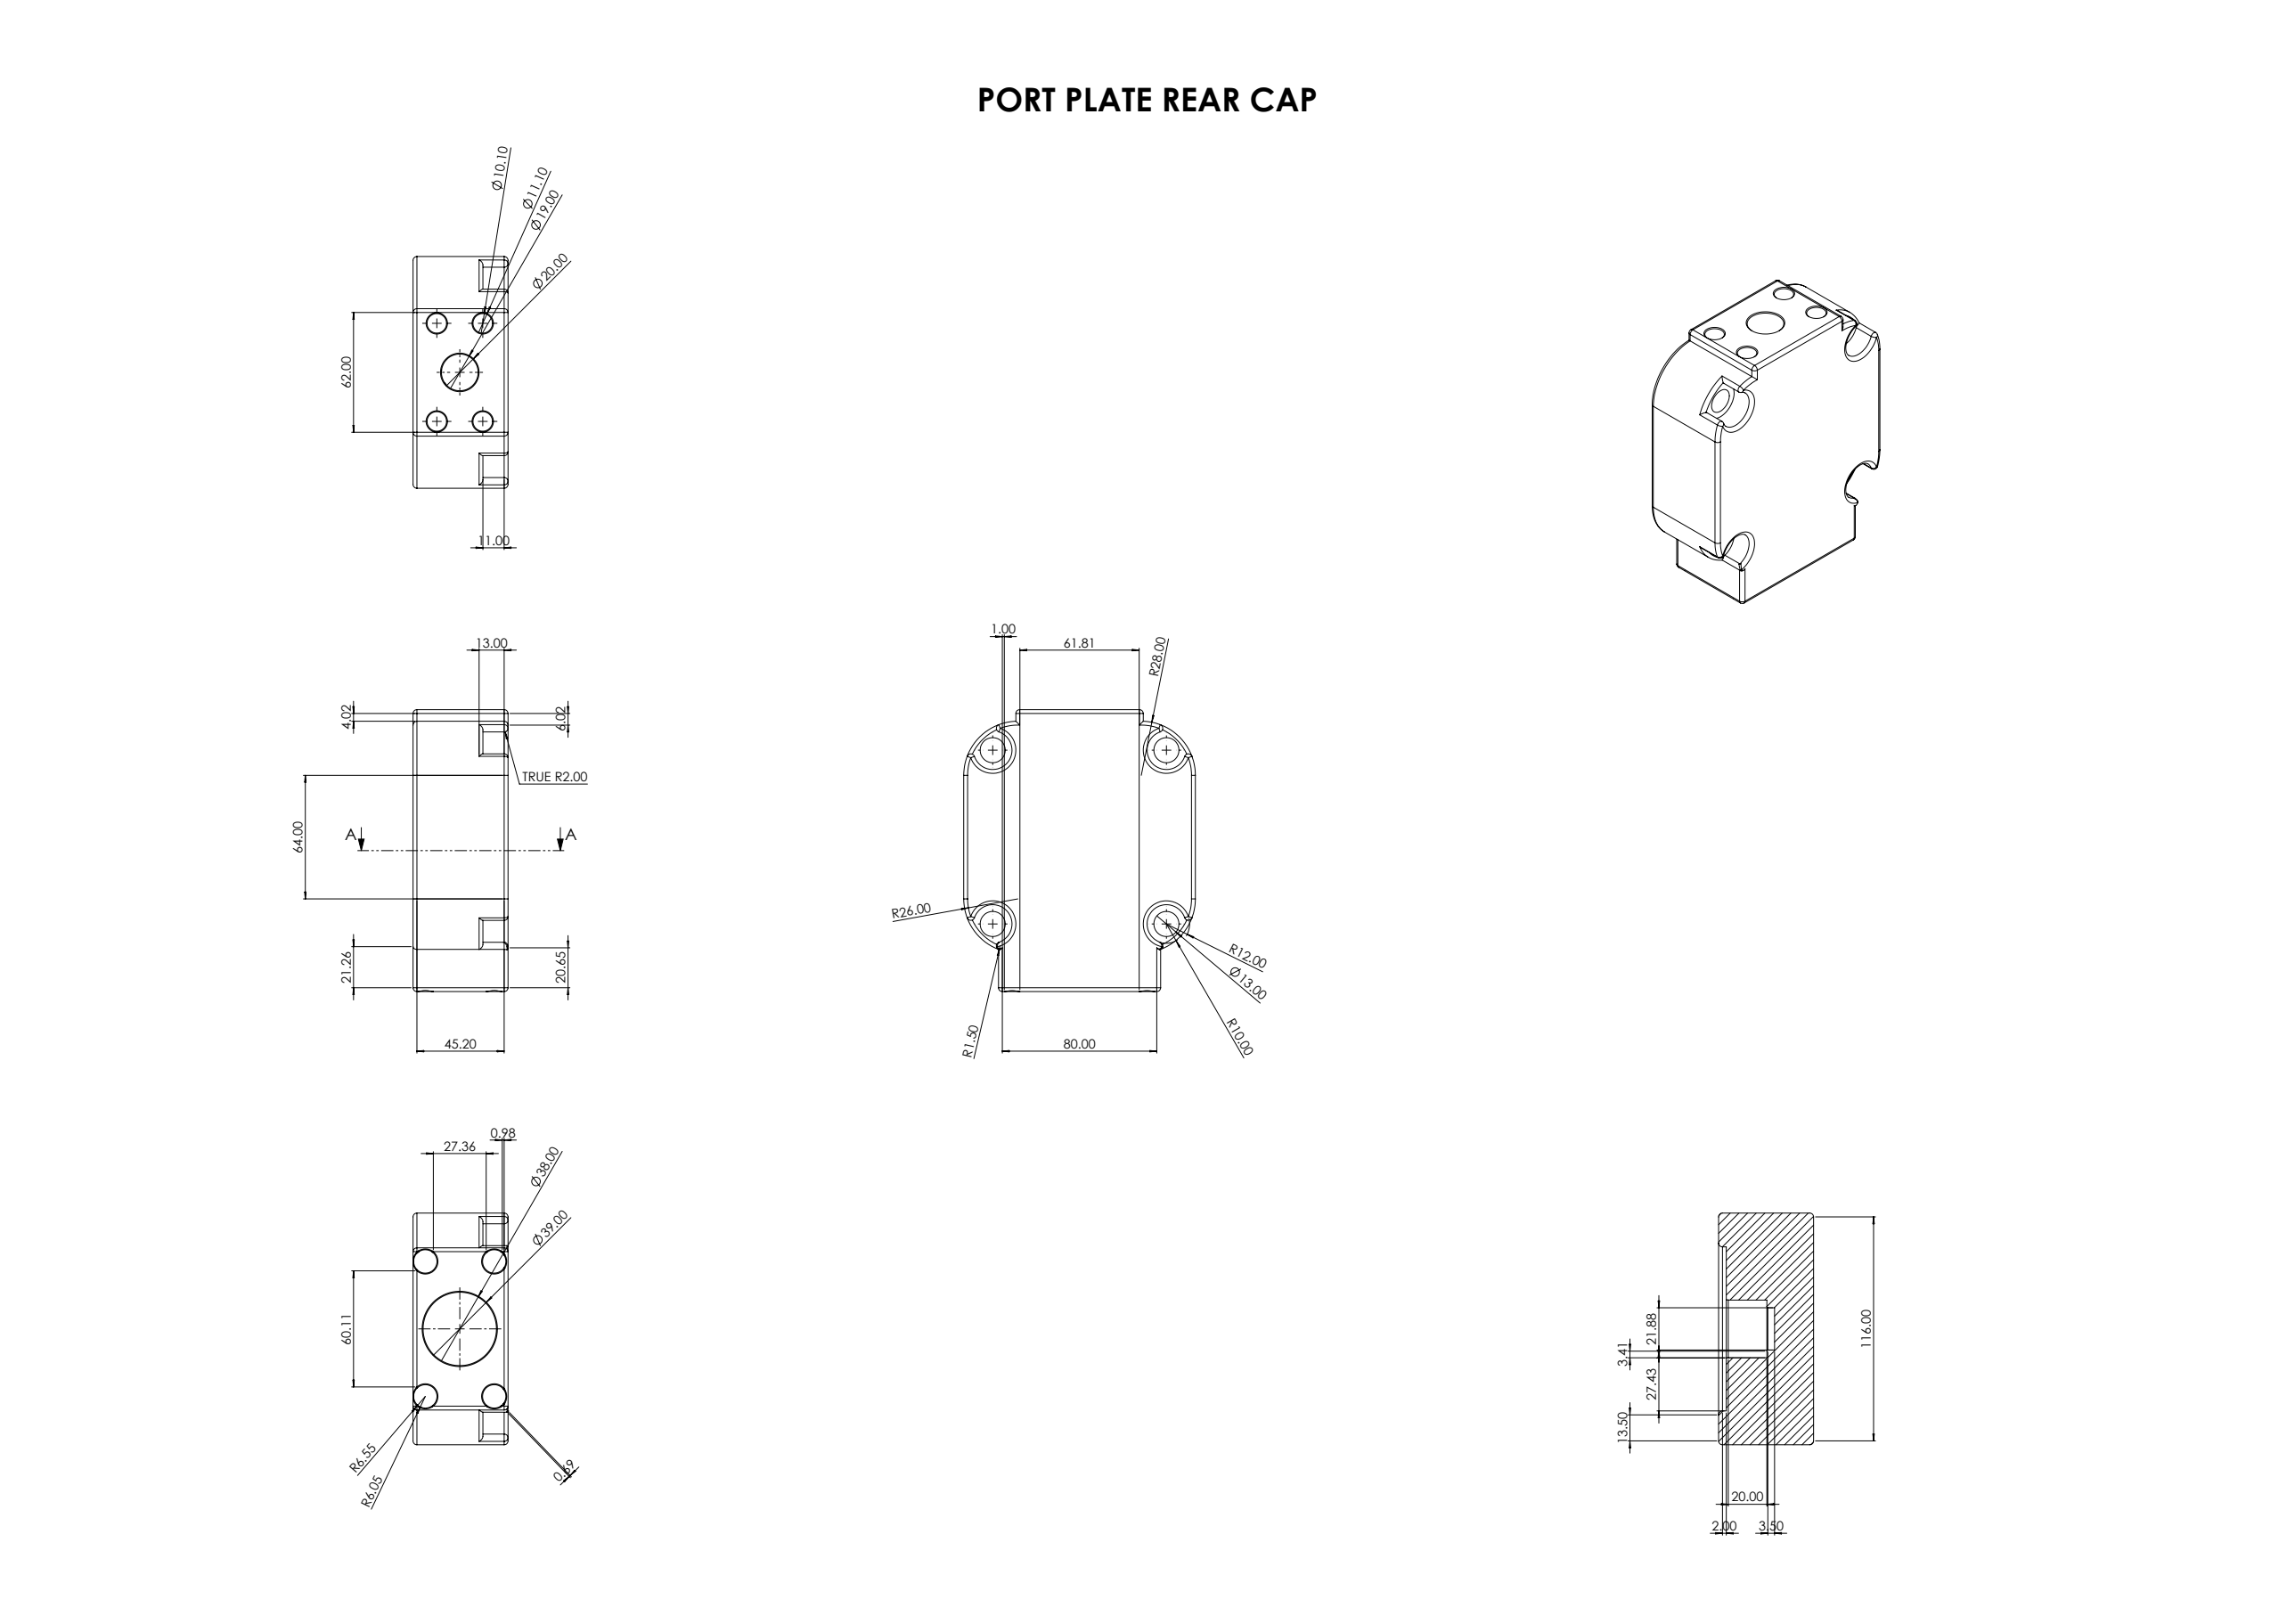
ISO-10303-21;
HEADER;
/* Generated by software containing ST-Developer
 * from STEP Tools, Inc. (www.steptools.com) 
 */

FILE_DESCRIPTION(
/* description */ (''),
/* implementation_level */ '2;1');

FILE_NAME(
/* name */ '02_Port_Plate_Rear_Cap.step',
/* time_stamp */ '2026-10-26T07:49:00-07:00',
/* author */ (''),
/* organization */ (''),
/* preprocessor_version */ 'ST-DEVELOPER v20.2',
/* originating_system */ 'Autodesk Translation Framework v15.15.0.0',
/* authorisation */ '');

FILE_SCHEMA (('AUTOMOTIVE_DESIGN { 1 0 10303 214 3 1 1 }'));
ENDSEC;

DATA;
#10=MECHANICAL_DESIGN_GEOMETRIC_PRESENTATION_REPRESENTATION('',(#178),#38507);
#132=SPHERICAL_SURFACE('',#15608,1.99999999999999);
#133=SPHERICAL_SURFACE('',#15617,2.);
#134=SPHERICAL_SURFACE('',#15621,2.);
#135=SPHERICAL_SURFACE('',#15628,2.);
#136=SPHERICAL_SURFACE('',#15630,2.);
#137=SPHERICAL_SURFACE('',#15636,2.);
#138=SPHERICAL_SURFACE('',#15638,2.);
#139=SPHERICAL_SURFACE('',#15719,2.);
#140=SPHERICAL_SURFACE('',#15722,2.);
#141=SPHERICAL_SURFACE('',#15737,2.);
#142=SPHERICAL_SURFACE('',#15745,1.99999999999999);
#143=SPHERICAL_SURFACE('',#15749,1.99999999999999);
#144=SPHERICAL_SURFACE('',#15753,1.99999999999999);
#145=SPHERICAL_SURFACE('',#15769,1.99999999999999);
#148=SHAPE_REPRESENTATION_RELATIONSHIP('SRR','None',#38576,#163);
#163=ADVANCED_BREP_SHAPE_REPRESENTATION('',(#193),#38493);
#178=STYLED_ITEM('',(#38713),#193);
#193=MANIFOLD_SOLID_BREP('Body1',#15072);
#215=B_SPLINE_SURFACE_WITH_KNOTS('',3,3,((#22745,#22746,#22747,#22748,#22749,
#22750,#22751,#22752,#22753,#22754,#22755,#22756),(#22757,#22758,#22759,
#22760,#22761,#22762,#22763,#22764,#22765,#22766,#22767,#22768),(#22769,
#22770,#22771,#22772,#22773,#22774,#22775,#22776,#22777,#22778,#22779,#22780),
(#22781,#22782,#22783,#22784,#22785,#22786,#22787,#22788,#22789,#22790,
#22791,#22792)),.UNSPECIFIED.,.F.,.F.,.F.,(4,4),(4,2,2,2,2,4),(0.,1.),(1.10145879772751,
1.32414222732706,1.45197453595802,1.57980684458897,1.70763915321993,1.80249027418853),
 .UNSPECIFIED.);
#216=B_SPLINE_SURFACE_WITH_KNOTS('',3,3,((#22823,#22824,#22825,#22826),
(#22827,#22828,#22829,#22830),(#22831,#22832,#22833,#22834),(#22835,#22836,
#22837,#22838)),.UNSPECIFIED.,.F.,.F.,.F.,(4,4),(4,4),(0.,1.),(-2.26119471261739,
-2.15398534032161),.UNSPECIFIED.);
#217=B_SPLINE_SURFACE_WITH_KNOTS('',3,3,((#22856,#22857,#22858,#22859),
(#22860,#22861,#22862,#22863),(#22864,#22865,#22866,#22867),(#22868,#22869,
#22870,#22871)),.UNSPECIFIED.,.F.,.F.,.F.,(4,4),(4,4),(0.,1.),(-0.987607313268187,
-0.880397940972402),.UNSPECIFIED.);
#218=B_SPLINE_SURFACE_WITH_KNOTS('',3,3,((#22880,#22881,#22882,#22883,#22884,
#22885,#22886,#22887),(#22888,#22889,#22890,#22891,#22892,#22893,#22894,
#22895),(#22896,#22897,#22898,#22899,#22900,#22901,#22902,#22903),(#22904,
#22905,#22906,#22907,#22908,#22909,#22910,#22911)),.UNSPECIFIED.,.F.,.F.,
 .F.,(4,4),(4,1,1,2,4),(0.,1.),(2.51916325679745,2.63563179243579,2.86856886371248,
3.10150593498916,3.18038929530694),.UNSPECIFIED.);
#219=B_SPLINE_SURFACE_WITH_KNOTS('',3,3,((#22934,#22935,#22936,#22937),
(#22938,#22939,#22940,#22941),(#22942,#22943,#22944,#22945),(#22946,#22947,
#22948,#22949)),.UNSPECIFIED.,.F.,.F.,.F.,(4,4),(4,4),(0.,1.),(-0.666064399610344,
-0.552453261527181),.UNSPECIFIED.);
#220=B_SPLINE_SURFACE_WITH_KNOTS('',3,3,((#22958,#22959,#22960,#22961),
(#22962,#22963,#22964,#22965),(#22966,#22967,#22968,#22969),(#22970,#22971,
#22972,#22973)),.UNSPECIFIED.,.F.,.F.,.F.,(4,4),(4,4),(0.,1.),(-5.7307320456524,
-5.61712090756923),.UNSPECIFIED.);
#221=B_SPLINE_SURFACE_WITH_KNOTS('',3,3,((#23021,#23022,#23023,#23024,#23025,
#23026,#23027,#23028,#23029,#23030,#23031,#23032),(#23033,#23034,#23035,
#23036,#23037,#23038,#23039,#23040,#23041,#23042,#23043,#23044),(#23045,
#23046,#23047,#23048,#23049,#23050,#23051,#23052,#23053,#23054,#23055,#23056),
(#23057,#23058,#23059,#23060,#23061,#23062,#23063,#23064,#23065,#23066,
#23067,#23068)),.UNSPECIFIED.,.F.,.F.,.F.,(4,4),(4,1,1,1,1,1,1,2,4),(0.,
1.),(1.17201798267167,1.354117347086,1.53621671150032,1.62726639370748,
1.67279123481106,1.71831607591465,1.90041544032897,2.08251480474329,2.14666332293336),
 .UNSPECIFIED.);
#222=B_SPLINE_SURFACE_WITH_KNOTS('',3,3,((#23104,#23105,#23106,#23107),
(#23108,#23109,#23110,#23111),(#23112,#23113,#23114,#23115),(#23116,#23117,
#23118,#23119)),.UNSPECIFIED.,.F.,.F.,.F.,(4,4),(4,4),(0.,1.),(2.29711532831763,
2.37317063593509),.UNSPECIFIED.);
#223=B_SPLINE_SURFACE_WITH_KNOTS('',3,3,((#23137,#23138,#23139,#23140),
(#23141,#23142,#23143,#23144),(#23145,#23146,#23147,#23148),(#23149,#23150,
#23151,#23152)),.UNSPECIFIED.,.F.,.F.,.F.,(4,4),(4,4),(0.,1.),(-2.37317063593509,
-2.29711532831763),.UNSPECIFIED.);
#224=B_SPLINE_SURFACE_WITH_KNOTS('',3,3,((#23161,#23162,#23163,#23164,#23165,
#23166,#23167,#23168),(#23169,#23170,#23171,#23172,#23173,#23174,#23175,
#23176),(#23177,#23178,#23179,#23180,#23181,#23182,#23183,#23184),(#23185,
#23186,#23187,#23188,#23189,#23190,#23191,#23192)),.UNSPECIFIED.,.F.,.F.,
 .F.,(4,4),(4,1,1,2,4),(0.,1.),(1.10145879772751,1.34393093992448,1.46516701102296,
1.70763915321993,1.80249027418852),.UNSPECIFIED.);
#225=B_SPLINE_SURFACE_WITH_KNOTS('',3,3,((#23215,#23216,#23217,#23218),
(#23219,#23220,#23221,#23222),(#23223,#23224,#23225,#23226),(#23227,#23228,
#23229,#23230)),.UNSPECIFIED.,.F.,.F.,.F.,(4,4),(4,4),(0.,1.),(-2.26119471261739,
-2.1539853403216),.UNSPECIFIED.);
#226=B_SPLINE_SURFACE_WITH_KNOTS('',3,3,((#23239,#23240,#23241,#23242),
(#23243,#23244,#23245,#23246),(#23247,#23248,#23249,#23250),(#23251,#23252,
#23253,#23254)),.UNSPECIFIED.,.F.,.F.,.F.,(4,4),(4,4),(0.,1.),(-0.987607313268191,
-0.880397940972402),.UNSPECIFIED.);
#227=B_SPLINE_SURFACE_WITH_KNOTS('',3,3,((#23285,#23286,#23287,#23288,#23289,
#23290,#23291,#23292,#23293,#23294),(#23295,#23296,#23297,#23298,#23299,
#23300,#23301,#23302,#23303,#23304),(#23305,#23306,#23307,#23308,#23309,
#23310,#23311,#23312,#23313,#23314),(#23315,#23316,#23317,#23318,#23319,
#23320,#23321,#23322,#23323,#23324)),.UNSPECIFIED.,.F.,.F.,.F.,(4,4),(4,
2,1,1,1,1,4),(0.,1.),(2.55343333368553,2.64828445465413,2.76952052575261,
2.89075659685109,3.01199266794958,3.07261070349882,3.25446481014654),
 .UNSPECIFIED.);
#228=B_SPLINE_SURFACE_WITH_KNOTS('',3,3,((#23351,#23352,#23353,#23354),
(#23355,#23356,#23357,#23358),(#23359,#23360,#23361,#23362),(#23363,#23364,
#23365,#23366)),.UNSPECIFIED.,.F.,.F.,.F.,(4,4),(4,4),(0.,1.),(-5.40278736620718,
-5.29557799391139),.UNSPECIFIED.);
#229=B_SPLINE_SURFACE_WITH_KNOTS('',3,3,((#23383,#23384,#23385,#23386),
(#23387,#23388,#23389,#23390),(#23391,#23392,#23393,#23394),(#23395,#23396,
#23397,#23398)),.UNSPECIFIED.,.F.,.F.,.F.,(4,4),(4,4),(0.,1.),(-4.12919996685799,
-4.0219905945622),.UNSPECIFIED.);
#230=B_SPLINE_SURFACE_WITH_KNOTS('',3,3,((#23407,#23408,#23409,#23410,#23411,
#23412),(#23413,#23414,#23415,#23416,#23417,#23418),(#23419,#23420,#23421,
#23422,#23423,#23424),(#23425,#23426,#23427,#23428,#23429,#23430)),
 .UNSPECIFIED.,.F.,.F.,.F.,(4,4),(4,1,1,4),(0.,1.),(2.51916325679745,2.70808498208588,
2.8970067073743,3.18038929530694),.UNSPECIFIED.);
#231=B_SPLINE_SURFACE_WITH_KNOTS('',3,3,((#23441,#23442,#23443,#23444),
(#23445,#23446,#23447,#23448),(#23449,#23450,#23451,#23452),(#23453,#23454,
#23455,#23456)),.UNSPECIFIED.,.F.,.F.,.F.,(4,4),(4,4),(0.,1.),(-0.666064399610344,
-0.552453261527181),.UNSPECIFIED.);
#232=B_SPLINE_SURFACE_WITH_KNOTS('',3,3,((#23461,#23462,#23463,#23464),
(#23465,#23466,#23467,#23468),(#23469,#23470,#23471,#23472),(#23473,#23474,
#23475,#23476)),.UNSPECIFIED.,.F.,.F.,.F.,(4,4),(4,4),(0.,1.),(-5.7307320456524,
-5.61712090756924),.UNSPECIFIED.);
#233=B_SPLINE_SURFACE_WITH_KNOTS('',3,3,((#23491,#23492,#23493,#23494,#23495,
#23496),(#23497,#23498,#23499,#23500,#23501,#23502),(#23503,#23504,#23505,
#23506,#23507,#23508),(#23509,#23510,#23511,#23512,#23513,#23514)),
 .UNSPECIFIED.,.F.,.F.,.F.,(4,4),(4,1,1,4),(0.,1.),(2.55343333368552,2.85387539502596,
3.05417010258625,3.25446481014654),.UNSPECIFIED.);
#234=B_SPLINE_SURFACE_WITH_KNOTS('',3,3,((#23533,#23534,#23535,#23536),
(#23537,#23538,#23539,#23540),(#23541,#23542,#23543,#23544),(#23545,#23546,
#23547,#23548)),.UNSPECIFIED.,.F.,.F.,.F.,(4,4),(4,4),(0.,1.),(0.880397940972406,
0.987607313268191),.UNSPECIFIED.);
#235=B_SPLINE_SURFACE_WITH_KNOTS('',3,3,((#23566,#23567,#23568,#23569),
(#23570,#23571,#23572,#23573),(#23574,#23575,#23576,#23577),(#23578,#23579,
#23580,#23581)),.UNSPECIFIED.,.F.,.F.,.F.,(4,4),(4,4),(0.,1.),(2.1539853403216,
2.26119471261739),.UNSPECIFIED.);
#236=B_SPLINE_SURFACE_WITH_KNOTS('',3,3,((#23590,#23591,#23592,#23593,#23594,
#23595,#23596,#23597,#23598,#23599,#23600,#23601,#23602),(#23603,#23604,
#23605,#23606,#23607,#23608,#23609,#23610,#23611,#23612,#23613,#23614,#23615),
(#23616,#23617,#23618,#23619,#23620,#23621,#23622,#23623,#23624,#23625,
#23626,#23627,#23628),(#23629,#23630,#23631,#23632,#23633,#23634,#23635,
#23636,#23637,#23638,#23639,#23640,#23641)),.UNSPECIFIED.,.F.,.F.,.F.,(4,
4),(4,2,1,1,1,1,1,2,4),(0.,1.),(1.17201798267168,1.23616650086174,1.37722455150867,
1.51828260215559,1.58881162747905,1.65934065280252,1.80039870344944,1.94145675409637,
2.14666332293336),.UNSPECIFIED.);
#237=B_SPLINE_SURFACE_WITH_KNOTS('',3,3,((#23679,#23680,#23681,#23682),
(#23683,#23684,#23685,#23686),(#23687,#23688,#23689,#23690),(#23691,#23692,
#23693,#23694)),.UNSPECIFIED.,.F.,.F.,.F.,(4,4),(4,4),(0.,1.),(2.29711532831763,
2.37317063593509),.UNSPECIFIED.);
#238=B_SPLINE_SURFACE_WITH_KNOTS('',3,3,((#23703,#23704,#23705,#23706),
(#23707,#23708,#23709,#23710),(#23711,#23712,#23713,#23714),(#23715,#23716,
#23717,#23718)),.UNSPECIFIED.,.F.,.F.,.F.,(4,4),(4,4),(0.,1.),(-2.37317063593509,
-2.29711532831763),.UNSPECIFIED.);
#239=B_SPLINE_SURFACE_WITH_KNOTS('',3,3,((#23741,#23742,#23743,#23744),
(#23745,#23746,#23747,#23748),(#23749,#23750,#23751,#23752),(#23753,#23754,
#23755,#23756)),.UNSPECIFIED.,.F.,.F.,.F.,(4,4),(4,4),(0.,1.),(-0.626198664785115,
-0.624325079343485),.UNSPECIFIED.);
#240=B_SPLINE_SURFACE_WITH_KNOTS('',3,3,((#23777,#23778,#23779,#23780,#23781,
#23782,#23783,#23784,#23785,#23786),(#23787,#23788,#23789,#23790,#23791,
#23792,#23793,#23794,#23795,#23796),(#23797,#23798,#23799,#23800,#23801,
#23802,#23803,#23804,#23805,#23806),(#23807,#23808,#23809,#23810,#23811,
#23812,#23813,#23814,#23815,#23816)),.UNSPECIFIED.,.F.,.F.,.F.,(4,4),(4,
2,2,2,4),(0.,1.),(-0.624325079343485,-0.380129337104056,-0.301935532404242,
-0.237254059228639,-0.209869946944685),.UNSPECIFIED.);
#241=B_SPLINE_SURFACE_WITH_KNOTS('',3,3,((#23843,#23844,#23845,#23846),
(#23847,#23848,#23849,#23850),(#23851,#23852,#23853,#23854),(#23855,#23856,
#23857,#23858)),.UNSPECIFIED.,.F.,.F.,.F.,(4,4),(4,4),(0.,1.),(-0.626730655849168,
-0.626198664785115),.UNSPECIFIED.);
#242=B_SPLINE_SURFACE_WITH_KNOTS('',3,3,((#23898,#23899,#23900,#23901),
(#23902,#23903,#23904,#23905),(#23906,#23907,#23908,#23909),(#23910,#23911,
#23912,#23913)),.UNSPECIFIED.,.F.,.F.,.F.,(4,4),(4,4),(0.,1.),(1.48736624018428,
1.50825556499841),.UNSPECIFIED.);
#243=B_SPLINE_SURFACE_WITH_KNOTS('',3,3,((#23922,#23923,#23924,#23925),
(#23926,#23927,#23928,#23929),(#23930,#23931,#23932,#23933),(#23934,#23935,
#23936,#23937)),.UNSPECIFIED.,.F.,.F.,.F.,(4,4),(4,4),(0.,1.),(0.,1.),
 .UNSPECIFIED.);
#244=B_SPLINE_SURFACE_WITH_KNOTS('',3,3,((#23981,#23982,#23983,#23984,#23985),
(#23986,#23987,#23988,#23989,#23990),(#23991,#23992,#23993,#23994,#23995),
(#23996,#23997,#23998,#23999,#24000)),.UNSPECIFIED.,.F.,.F.,.F.,(4,4),(4,
1,4),(0.,1.),(0.,0.000208214441420064,0.000485833696646816),
 .UNSPECIFIED.);
#245=B_SPLINE_SURFACE_WITH_KNOTS('',3,3,((#24028,#24029,#24030,#24031),
(#24032,#24033,#24034,#24035),(#24036,#24037,#24038,#24039),(#24040,#24041,
#24042,#24043)),.UNSPECIFIED.,.F.,.F.,.F.,(4,4),(4,4),(0.,1.),(-0.00166298225714781,
0.),.UNSPECIFIED.);
#246=B_SPLINE_SURFACE_WITH_KNOTS('',3,3,((#24062,#24063,#24064,#24065,#24066,
#24067,#24068,#24069,#24070,#24071,#24072,#24073),(#24074,#24075,#24076,
#24077,#24078,#24079,#24080,#24081,#24082,#24083,#24084,#24085),(#24086,
#24087,#24088,#24089,#24090,#24091,#24092,#24093,#24094,#24095,#24096,#24097),
(#24098,#24099,#24100,#24101,#24102,#24103,#24104,#24105,#24106,#24107,
#24108,#24109)),.UNSPECIFIED.,.F.,.F.,.F.,(4,4),(4,2,2,2,2,4),(0.,1.),(-0.369530672027591,
-0.345224711421131,-0.287813854984672,-0.218409540651057,-0.120337282444558,
-0.00166298225714781),.UNSPECIFIED.);
#247=B_SPLINE_SURFACE_WITH_KNOTS('',3,3,((#24157,#24158,#24159,#24160),
(#24161,#24162,#24163,#24164),(#24165,#24166,#24167,#24168),(#24169,#24170,
#24171,#24172)),.UNSPECIFIED.,.F.,.F.,.F.,(4,4),(4,4),(0.,1.),(4.77492974218118,
4.7958190669953),.UNSPECIFIED.);
#248=B_SPLINE_SURFACE_WITH_KNOTS('',3,3,((#24181,#24182,#24183,#24184),
(#24185,#24186,#24187,#24188),(#24189,#24190,#24191,#24192),(#24193,#24194,
#24195,#24196)),.UNSPECIFIED.,.F.,.F.,.F.,(4,4),(4,4),(0.,1.),(0.,1.),
 .UNSPECIFIED.);
#249=B_SPLINE_SURFACE_WITH_KNOTS('',3,3,((#24333,#24334,#24335,#24336,#24337,
#24338,#24339,#24340,#24341,#24342,#24343,#24344,#24345,#24346,#24347,#24348,
#24349,#24350,#24351,#24352,#24353,#24354),(#24355,#24356,#24357,#24358,
#24359,#24360,#24361,#24362,#24363,#24364,#24365,#24366,#24367,#24368,#24369,
#24370,#24371,#24372,#24373,#24374,#24375,#24376),(#24377,#24378,#24379,
#24380,#24381,#24382,#24383,#24384,#24385,#24386,#24387,#24388,#24389,#24390,
#24391,#24392,#24393,#24394,#24395,#24396,#24397,#24398),(#24399,#24400,
#24401,#24402,#24403,#24404,#24405,#24406,#24407,#24408,#24409,#24410,#24411,
#24412,#24413,#24414,#24415,#24416,#24417,#24418,#24419,#24420),(#24421,
#24422,#24423,#24424,#24425,#24426,#24427,#24428,#24429,#24430,#24431,#24432,
#24433,#24434,#24435,#24436,#24437,#24438,#24439,#24440,#24441,#24442)),
 .UNSPECIFIED.,.F.,.T.,.F.,(4,1,4),(4,1,1,1,1,1,1,1,1,1,1,1,1,1,1,1,1,1,
1,4),(0.,0.571428571428571,1.),(0.,0.133807235852271,0.267614471704543,
0.535228943409085,0.802843415113627,1.07045788681817,1.2488675346212,1.42727718242423,
1.60568683022725,1.78409647803028,1.96250612583331,2.14091577363634,2.40853024534088,
2.54233748119315,2.67614471704543,2.94375918874997,3.21137366045451,3.47898813215905,
3.61279536801132,3.74660260386359),.UNSPECIFIED.);
#250=B_SPLINE_SURFACE_WITH_KNOTS('',3,3,((#24656,#24657,#24658,#24659,#24660,
#24661,#24662,#24663,#24664,#24665,#24666,#24667,#24668,#24669,#24670,#24671,
#24672,#24673),(#24674,#24675,#24676,#24677,#24678,#24679,#24680,#24681,
#24682,#24683,#24684,#24685,#24686,#24687,#24688,#24689,#24690,#24691),
(#24692,#24693,#24694,#24695,#24696,#24697,#24698,#24699,#24700,#24701,
#24702,#24703,#24704,#24705,#24706,#24707,#24708,#24709),(#24710,#24711,
#24712,#24713,#24714,#24715,#24716,#24717,#24718,#24719,#24720,#24721,#24722,
#24723,#24724,#24725,#24726,#24727),(#24728,#24729,#24730,#24731,#24732,
#24733,#24734,#24735,#24736,#24737,#24738,#24739,#24740,#24741,#24742,#24743,
#24744,#24745),(#24746,#24747,#24748,#24749,#24750,#24751,#24752,#24753,
#24754,#24755,#24756,#24757,#24758,#24759,#24760,#24761,#24762,#24763)),
 .UNSPECIFIED.,.F.,.F.,.F.,(4,1,1,4),(4,1,1,1,1,1,1,1,1,1,1,1,1,1,1,4),
(0.,0.285714285714286,0.571428571428571,1.),(-4.47914967830435,-4.15921041556833,
-3.8392711528323,-3.51933189009628,-3.19939262736025,-2.98609978553623,
-2.77280694371222,-2.5595141018882,-2.13292841824016,-1.91963557641615,
-1.59969631368012,-1.2797570509441,-0.959817788208071,-0.639878525472046,
-0.319939262736021,4.7375248461733E-15),.UNSPECIFIED.);
#251=B_SPLINE_SURFACE_WITH_KNOTS('',3,3,((#25021,#25022,#25023,#25024,#25025,
#25026,#25027,#25028),(#25029,#25030,#25031,#25032,#25033,#25034,#25035,
#25036),(#25037,#25038,#25039,#25040,#25041,#25042,#25043,#25044),(#25045,
#25046,#25047,#25048,#25049,#25050,#25051,#25052),(#25053,#25054,#25055,
#25056,#25057,#25058,#25059,#25060),(#25061,#25062,#25063,#25064,#25065,
#25066,#25067,#25068)),.UNSPECIFIED.,.F.,.F.,.F.,(4,1,1,4),(4,1,1,1,1,4),
(0.,0.285714285714286,0.571428571428571,1.),(-1.49199371745016,-1.06570979817868,
-0.852567838542947,-0.426283919271474,-0.213141959635737,0.),
 .UNSPECIFIED.);
#274=TOROIDAL_SURFACE('',#15563,12.,2.);
#275=TOROIDAL_SURFACE('',#15654,45.05,2.);
#276=TOROIDAL_SURFACE('',#15660,26.,2.);
#277=TOROIDAL_SURFACE('',#15665,26.,2.);
#278=TOROIDAL_SURFACE('',#15671,26.,2.);
#279=TOROIDAL_SURFACE('',#15678,26.,2.);
#280=TOROIDAL_SURFACE('',#15684,26.,2.);
#281=TOROIDAL_SURFACE('',#15692,26.,2.);
#282=TOROIDAL_SURFACE('',#15703,26.,2.);
#283=TOROIDAL_SURFACE('',#15704,26.,2.);
#284=TOROIDAL_SURFACE('',#15710,26.,2.);
#285=TOROIDAL_SURFACE('',#15716,26.,2.);
#286=TOROIDAL_SURFACE('',#15725,12.,2.);
#287=TOROIDAL_SURFACE('',#15738,12.,2.);
#288=TOROIDAL_SURFACE('',#15756,26.,2.);
#289=TOROIDAL_SURFACE('',#15760,26.,2.);
#290=TOROIDAL_SURFACE('',#15763,12.,2.);
#291=TOROIDAL_SURFACE('',#15766,26.,2.);
#292=TOROIDAL_SURFACE('',#15772,26.,2.);
#336=(
BOUNDED_CURVE()
B_SPLINE_CURVE(3,(#24045,#24046,#24047,#24048,#24049,#24050),
 .UNSPECIFIED.,.F.,.F.)
B_SPLINE_CURVE_WITH_KNOTS((4,2,4),(0.,0.00123256806504644,0.00166298225708981),
 .UNSPECIFIED.)
CURVE()
GEOMETRIC_REPRESENTATION_ITEM()
RATIONAL_B_SPLINE_CURVE((1.,1.,1.,1.,1.,1.))
REPRESENTATION_ITEM('')
);
#337=(
BOUNDED_CURVE()
B_SPLINE_CURVE(3,(#24056,#24057,#24058,#24059,#24060,#24061),
 .UNSPECIFIED.,.F.,.F.)
B_SPLINE_CURVE_WITH_KNOTS((4,2,4),(-0.00166298225712823,-0.00123256806504644,
0.),.UNSPECIFIED.)
CURVE()
GEOMETRIC_REPRESENTATION_ITEM()
RATIONAL_B_SPLINE_CURVE((1.,1.,1.,1.,1.,1.))
REPRESENTATION_ITEM('')
);
#435=FACE_BOUND('',#2644,.T.);
#436=FACE_BOUND('',#2648,.T.);
#437=FACE_BOUND('',#2709,.T.);
#438=FACE_BOUND('',#2710,.T.);
#439=FACE_BOUND('',#2711,.T.);
#440=FACE_BOUND('',#2712,.T.);
#441=FACE_BOUND('',#2713,.T.);
#442=FACE_BOUND('',#2747,.T.);
#443=FACE_BOUND('',#2748,.T.);
#444=FACE_BOUND('',#2749,.T.);
#445=FACE_BOUND('',#2750,.T.);
#446=FACE_BOUND('',#2751,.T.);
#447=FACE_BOUND('',#2760,.T.);
#448=FACE_BOUND('',#2761,.T.);
#449=FACE_BOUND('',#2762,.T.);
#450=FACE_BOUND('',#2765,.T.);
#451=FACE_BOUND('',#2770,.T.);
#452=FACE_BOUND('',#2773,.T.);
#453=FACE_BOUND('',#2818,.T.);
#454=FACE_BOUND('',#2832,.T.);
#594=PLANE('',#15499);
#595=PLANE('',#15506);
#596=PLANE('',#15519);
#597=PLANE('',#15530);
#598=PLANE('',#15549);
#599=PLANE('',#15567);
#600=PLANE('',#15580);
#601=PLANE('',#15623);
#602=PLANE('',#15642);
#603=PLANE('',#15643);
#604=PLANE('',#15644);
#605=PLANE('',#15669);
#606=PLANE('',#15674);
#607=PLANE('',#15687);
#608=PLANE('',#15695);
#609=PLANE('',#15709);
#610=PLANE('',#15731);
#611=PLANE('',#15734);
#612=PLANE('',#15780);
#613=PLANE('',#15782);
#614=PLANE('',#15783);
#615=PLANE('',#15784);
#616=PLANE('',#15785);
#617=PLANE('',#15786);
#618=PLANE('',#15787);
#619=PLANE('',#15788);
#620=PLANE('',#15789);
#621=PLANE('',#15790);
#622=PLANE('',#15791);
#623=PLANE('',#15794);
#624=PLANE('',#15797);
#625=PLANE('',#15798);
#1059=B_SPLINE_CURVE_WITH_KNOTS('',3,(#22669,#22670,#22671,#22672,#22673,
#22674,#22675,#22676,#22677,#22678,#22679,#22680,#22681,#22682,#22683,#22684,
#22685,#22686,#22687,#22688,#22689,#22690,#22691,#22692,#22693,#22694,#22695,
#22696,#22697,#22698,#22699,#22700,#22701,#22702),.UNSPECIFIED.,.F.,.F.,
(4,3,3,3,3,3,3,3,3,3,3,4),(-2.73245898532687,-2.53728230507538,-2.34210562482388,
-2.14692894457238,-1.95175226432089,-1.82163447748656,-1.69151669065223,
-1.56139890381789,-1.30116333014923,-1.1710455433149,-0.975868863063405,
-0.910819924833371),.UNSPECIFIED.);
#1060=B_SPLINE_CURVE_WITH_KNOTS('',3,(#22705,#22706,#22707,#22708,#22709,
#22710,#22711,#22712,#22713,#22714,#22715,#22716,#22717,#22718,#22719,#22720),
 .UNSPECIFIED.,.F.,.F.,(4,3,3,3,3,4),(-3.64328476398188,-3.3830488272233,
-3.25293085884402,-2.99269492208545,-2.86257695370616,-2.73245898532687),
 .UNSPECIFIED.);
#1061=B_SPLINE_CURVE_WITH_KNOTS('',3,(#22721,#22722,#22723,#22724,#22725,
#22726,#22727,#22728,#22729,#22730,#22731,#22732,#22733,#22734,#22735,#22736),
 .UNSPECIFIED.,.F.,.F.,(4,3,3,3,3,4),(-0.910819924833371,-0.780694259832976,
-0.585520694874732,-0.390347129916488,-0.195173564958244,0.),
 .UNSPECIFIED.);
#1062=B_SPLINE_CURVE_WITH_KNOTS('',3,(#22797,#22798,#22799,#22800,#22801,
#22802,#22803,#22804,#22805,#22806,#22807,#22808),.UNSPECIFIED.,.F.,.F.,
(4,2,2,2,2,4),(-1.80249027418853,-1.70763915321993,-1.57980684458897,-1.45197453595802,
-1.32414222732706,-1.10145879772751),.UNSPECIFIED.);
#1063=B_SPLINE_CURVE_WITH_KNOTS('',3,(#22811,#22812,#22813,#22814,#22815,
#22816,#22817,#22818,#22819,#22820,#22821,#22822),.UNSPECIFIED.,.F.,.F.,
(4,2,2,2,2,4),(1.10145879772751,1.32414222732706,1.45197453595802,1.57980684458897,
1.70763915321993,1.80249027418853),.UNSPECIFIED.);
#1064=B_SPLINE_CURVE_WITH_KNOTS('',3,(#22839,#22840,#22841,#22842),
 .UNSPECIFIED.,.F.,.F.,(4,4),(2.15398534032161,2.26119471261739),
 .UNSPECIFIED.);
#1065=B_SPLINE_CURVE_WITH_KNOTS('',3,(#22843,#22844,#22845,#22846),
 .UNSPECIFIED.,.F.,.F.,(4,4),(-2.26119471261739,-2.15398534032161),
 .UNSPECIFIED.);
#1066=B_SPLINE_CURVE_WITH_KNOTS('',3,(#22872,#22873,#22874,#22875),
 .UNSPECIFIED.,.F.,.F.,(4,4),(0.880397940972402,0.987607313268187),
 .UNSPECIFIED.);
#1067=B_SPLINE_CURVE_WITH_KNOTS('',3,(#22876,#22877,#22878,#22879),
 .UNSPECIFIED.,.F.,.F.,(4,4),(-0.987607313268187,-0.880397940972402),
 .UNSPECIFIED.);
#1068=B_SPLINE_CURVE_WITH_KNOTS('',3,(#22916,#22917,#22918,#22919,#22920,
#22921,#22922,#22923),.UNSPECIFIED.,.F.,.F.,(4,2,1,1,4),(-3.18038929530694,
-3.10150593498916,-2.86856886371248,-2.63563179243579,-2.51916325679745),
 .UNSPECIFIED.);
#1069=B_SPLINE_CURVE_WITH_KNOTS('',3,(#22926,#22927,#22928,#22929,#22930,
#22931,#22932,#22933),.UNSPECIFIED.,.F.,.F.,(4,1,1,2,4),(2.51916325679745,
2.63563179243579,2.86856886371248,3.10150593498916,3.18038929530694),
 .UNSPECIFIED.);
#1070=B_SPLINE_CURVE_WITH_KNOTS('',3,(#22950,#22951,#22952,#22953),
 .UNSPECIFIED.,.F.,.F.,(4,4),(0.552453261527181,0.666064399610344),
 .UNSPECIFIED.);
#1071=B_SPLINE_CURVE_WITH_KNOTS('',3,(#22954,#22955,#22956,#22957),
 .UNSPECIFIED.,.F.,.F.,(4,4),(-0.666064399610344,-0.552453261527181),
 .UNSPECIFIED.);
#1072=B_SPLINE_CURVE_WITH_KNOTS('',3,(#22974,#22975,#22976,#22977),
 .UNSPECIFIED.,.F.,.F.,(4,4),(5.61712090756923,5.7307320456524),
 .UNSPECIFIED.);
#1073=B_SPLINE_CURVE_WITH_KNOTS('',3,(#22978,#22979,#22980,#22981),
 .UNSPECIFIED.,.F.,.F.,(4,4),(-5.7307320456524,-5.61712090756923),
 .UNSPECIFIED.);
#1074=B_SPLINE_CURVE_WITH_KNOTS('',3,(#22988,#22989,#22990,#22991),
 .UNSPECIFIED.,.F.,.F.,(4,4),(0.552453261527181,0.666064399610344),
 .UNSPECIFIED.);
#1075=B_SPLINE_CURVE_WITH_KNOTS('',3,(#22993,#22994,#22995,#22996,#22997,
#22998),.UNSPECIFIED.,.F.,.F.,(4,1,1,4),(-3.18038929530694,-2.8970067073743,
-2.70808498208588,-2.51916325679745),.UNSPECIFIED.);
#1076=B_SPLINE_CURVE_WITH_KNOTS('',3,(#23000,#23001,#23002,#23003),
 .UNSPECIFIED.,.F.,.F.,(4,4),(5.61712090756924,5.7307320456524),
 .UNSPECIFIED.);
#1077=B_SPLINE_CURVE_WITH_KNOTS('',3,(#23073,#23074,#23075,#23076,#23077,
#23078,#23079,#23080,#23081,#23082,#23083,#23084),.UNSPECIFIED.,.F.,.F.,
(4,2,1,1,1,1,1,1,4),(-2.14666332293336,-2.08251480474329,-1.90041544032897,
-1.71831607591465,-1.67279123481106,-1.62726639370748,-1.53621671150032,
-1.354117347086,-1.17201798267167),.UNSPECIFIED.);
#1078=B_SPLINE_CURVE_WITH_KNOTS('',3,(#23088,#23089,#23090,#23091,#23092,
#23093,#23094),.UNSPECIFIED.,.F.,.F.,(4,1,1,1,4),(1.17201798267167,1.354117347086,
1.53621671150032,1.62726639370748,1.65922503472488),.UNSPECIFIED.);
#1079=B_SPLINE_CURVE_WITH_KNOTS('',3,(#23095,#23096,#23097,#23098,#23099,
#23100,#23101,#23102,#23103),.UNSPECIFIED.,.F.,.F.,(4,1,1,1,2,4),(1.65922503472488,
1.67279123481106,1.71831607591465,1.90041544032897,2.08251480474329,2.14666332293336),
 .UNSPECIFIED.);
#1080=B_SPLINE_CURVE_WITH_KNOTS('',3,(#23120,#23121,#23122,#23123),
 .UNSPECIFIED.,.F.,.F.,(4,4),(-2.37317063593509,-2.29711532831763),
 .UNSPECIFIED.);
#1081=B_SPLINE_CURVE_WITH_KNOTS('',3,(#23124,#23125,#23126,#23127),
 .UNSPECIFIED.,.F.,.F.,(4,4),(2.29711532831763,2.37317063593509),
 .UNSPECIFIED.);
#1082=B_SPLINE_CURVE_WITH_KNOTS('',3,(#23153,#23154,#23155,#23156),
 .UNSPECIFIED.,.F.,.F.,(4,4),(2.29711532831763,2.37317063593509),
 .UNSPECIFIED.);
#1083=B_SPLINE_CURVE_WITH_KNOTS('',3,(#23157,#23158,#23159,#23160),
 .UNSPECIFIED.,.F.,.F.,(4,4),(-2.37317063593509,-2.29711532831763),
 .UNSPECIFIED.);
#1084=B_SPLINE_CURVE_WITH_KNOTS('',3,(#23197,#23198,#23199,#23200,#23201,
#23202,#23203,#23204),.UNSPECIFIED.,.F.,.F.,(4,2,1,1,4),(-1.80249027418852,
-1.70763915321993,-1.46516701102296,-1.34393093992448,-1.10145879772751),
 .UNSPECIFIED.);
#1085=B_SPLINE_CURVE_WITH_KNOTS('',3,(#23207,#23208,#23209,#23210,#23211,
#23212,#23213,#23214),.UNSPECIFIED.,.F.,.F.,(4,1,1,2,4),(1.10145879772751,
1.34393093992448,1.46516701102296,1.70763915321993,1.80249027418852),
 .UNSPECIFIED.);
#1086=B_SPLINE_CURVE_WITH_KNOTS('',3,(#23231,#23232,#23233,#23234),
 .UNSPECIFIED.,.F.,.F.,(4,4),(2.1539853403216,2.26119471261739),
 .UNSPECIFIED.);
#1087=B_SPLINE_CURVE_WITH_KNOTS('',3,(#23235,#23236,#23237,#23238),
 .UNSPECIFIED.,.F.,.F.,(4,4),(-2.26119471261739,-2.1539853403216),
 .UNSPECIFIED.);
#1088=B_SPLINE_CURVE_WITH_KNOTS('',3,(#23255,#23256,#23257,#23258),
 .UNSPECIFIED.,.F.,.F.,(4,4),(0.880397940972402,0.987607313268191),
 .UNSPECIFIED.);
#1089=B_SPLINE_CURVE_WITH_KNOTS('',3,(#23259,#23260,#23261,#23262),
 .UNSPECIFIED.,.F.,.F.,(4,4),(-0.987607313268191,-0.880397940972402),
 .UNSPECIFIED.);
#1090=B_SPLINE_CURVE_WITH_KNOTS('',3,(#23329,#23330,#23331,#23332,#23333,
#23334,#23335,#23336,#23337,#23338),.UNSPECIFIED.,.F.,.F.,(4,1,1,1,1,2,
4),(-3.25446481014654,-3.07261070349882,-3.01199266794958,-2.89075659685109,
-2.76952052575261,-2.64828445465413,-2.55343333368553),.UNSPECIFIED.);
#1091=B_SPLINE_CURVE_WITH_KNOTS('',3,(#23341,#23342,#23343,#23344,#23345,
#23346,#23347,#23348,#23349,#23350),.UNSPECIFIED.,.F.,.F.,(4,2,1,1,1,1,
4),(2.55343333368553,2.64828445465413,2.76952052575261,2.89075659685109,
3.01199266794958,3.07261070349882,3.25446481014654),.UNSPECIFIED.);
#1092=B_SPLINE_CURVE_WITH_KNOTS('',3,(#23367,#23368,#23369,#23370),
 .UNSPECIFIED.,.F.,.F.,(4,4),(5.29557799391139,5.40278736620718),
 .UNSPECIFIED.);
#1093=B_SPLINE_CURVE_WITH_KNOTS('',3,(#23371,#23372,#23373,#23374),
 .UNSPECIFIED.,.F.,.F.,(4,4),(-5.40278736620718,-5.29557799391139),
 .UNSPECIFIED.);
#1094=B_SPLINE_CURVE_WITH_KNOTS('',3,(#23399,#23400,#23401,#23402),
 .UNSPECIFIED.,.F.,.F.,(4,4),(4.0219905945622,4.12919996685799),
 .UNSPECIFIED.);
#1095=B_SPLINE_CURVE_WITH_KNOTS('',3,(#23403,#23404,#23405,#23406),
 .UNSPECIFIED.,.F.,.F.,(4,4),(-4.12919996685799,-4.0219905945622),
 .UNSPECIFIED.);
#1096=B_SPLINE_CURVE_WITH_KNOTS('',3,(#23435,#23436,#23437,#23438,#23439,
#23440),.UNSPECIFIED.,.F.,.F.,(4,1,1,4),(2.51916325679745,2.70808498208588,
2.8970067073743,3.18038929530694),.UNSPECIFIED.);
#1097=B_SPLINE_CURVE_WITH_KNOTS('',3,(#23457,#23458,#23459,#23460),
 .UNSPECIFIED.,.F.,.F.,(4,4),(-0.666064399610344,-0.552453261527181),
 .UNSPECIFIED.);
#1098=B_SPLINE_CURVE_WITH_KNOTS('',3,(#23477,#23478,#23479,#23480),
 .UNSPECIFIED.,.F.,.F.,(4,4),(-5.7307320456524,-5.61712090756924),
 .UNSPECIFIED.);
#1099=B_SPLINE_CURVE_WITH_KNOTS('',3,(#23519,#23520,#23521,#23522,#23523,
#23524),.UNSPECIFIED.,.F.,.F.,(4,1,1,4),(-3.25446481014654,-3.05417010258625,
-2.85387539502596,-2.55343333368552),.UNSPECIFIED.);
#1100=B_SPLINE_CURVE_WITH_KNOTS('',3,(#23527,#23528,#23529,#23530,#23531,
#23532),.UNSPECIFIED.,.F.,.F.,(4,1,1,4),(2.55343333368552,2.85387539502596,
3.05417010258625,3.25446481014654),.UNSPECIFIED.);
#1101=B_SPLINE_CURVE_WITH_KNOTS('',3,(#23549,#23550,#23551,#23552),
 .UNSPECIFIED.,.F.,.F.,(4,4),(-0.987607313268191,-0.880397940972406),
 .UNSPECIFIED.);
#1102=B_SPLINE_CURVE_WITH_KNOTS('',3,(#23553,#23554,#23555,#23556),
 .UNSPECIFIED.,.F.,.F.,(4,4),(0.880397940972406,0.987607313268191),
 .UNSPECIFIED.);
#1103=B_SPLINE_CURVE_WITH_KNOTS('',3,(#23582,#23583,#23584,#23585),
 .UNSPECIFIED.,.F.,.F.,(4,4),(-2.26119471261739,-2.1539853403216),
 .UNSPECIFIED.);
#1104=B_SPLINE_CURVE_WITH_KNOTS('',3,(#23586,#23587,#23588,#23589),
 .UNSPECIFIED.,.F.,.F.,(4,4),(2.1539853403216,2.26119471261739),
 .UNSPECIFIED.);
#1105=B_SPLINE_CURVE_WITH_KNOTS('',3,(#23646,#23647,#23648,#23649,#23650,
#23651,#23652,#23653,#23654,#23655,#23656,#23657,#23658),.UNSPECIFIED.,
 .F.,.F.,(4,2,1,1,1,1,1,2,4),(-2.14666332293336,-1.94145675409637,-1.80039870344944,
-1.65934065280252,-1.58881162747905,-1.51828260215559,-1.37722455150867,
-1.23616650086174,-1.17201798267168),.UNSPECIFIED.);
#1106=B_SPLINE_CURVE_WITH_KNOTS('',3,(#23662,#23663,#23664,#23665,#23666,
#23667,#23668,#23669,#23670),.UNSPECIFIED.,.F.,.F.,(4,2,1,1,1,4),(1.17201798267168,
1.23616650086174,1.37722455150867,1.51828260215559,1.58881162747905,1.65930014766736),
 .UNSPECIFIED.);
#1107=B_SPLINE_CURVE_WITH_KNOTS('',3,(#23671,#23672,#23673,#23674,#23675,
#23676,#23677,#23678),.UNSPECIFIED.,.F.,.F.,(4,1,1,2,4),(1.65930014766736,
1.65934065280252,1.80039870344944,1.94145675409637,2.14666332293336),
 .UNSPECIFIED.);
#1108=B_SPLINE_CURVE_WITH_KNOTS('',3,(#23695,#23696,#23697,#23698),
 .UNSPECIFIED.,.F.,.F.,(4,4),(-2.37317063593509,-2.29711532831763),
 .UNSPECIFIED.);
#1109=B_SPLINE_CURVE_WITH_KNOTS('',3,(#23699,#23700,#23701,#23702),
 .UNSPECIFIED.,.F.,.F.,(4,4),(2.29711532831763,2.37317063593509),
 .UNSPECIFIED.);
#1110=B_SPLINE_CURVE_WITH_KNOTS('',3,(#23719,#23720,#23721,#23722),
 .UNSPECIFIED.,.F.,.F.,(4,4),(2.29711532831763,2.37317063593509),
 .UNSPECIFIED.);
#1111=B_SPLINE_CURVE_WITH_KNOTS('',3,(#23723,#23724,#23725,#23726),
 .UNSPECIFIED.,.F.,.F.,(4,4),(-2.37317063593509,-2.29711532831763),
 .UNSPECIFIED.);
#1112=B_SPLINE_CURVE_WITH_KNOTS('',3,(#23759,#23760,#23761,#23762),
 .UNSPECIFIED.,.F.,.F.,(4,4),(-1.,0.),.UNSPECIFIED.);
#1113=B_SPLINE_CURVE_WITH_KNOTS('',3,(#23764,#23765,#23766,#23767),
 .UNSPECIFIED.,.F.,.F.,(4,4),(-0.626198664785115,-0.624325079343485),
 .UNSPECIFIED.);
#1114=B_SPLINE_CURVE_WITH_KNOTS('',3,(#23769,#23770,#23771,#23772),
 .UNSPECIFIED.,.F.,.F.,(4,4),(-1.,0.),.UNSPECIFIED.);
#1115=B_SPLINE_CURVE_WITH_KNOTS('',3,(#23773,#23774,#23775,#23776),
 .UNSPECIFIED.,.F.,.F.,(4,4),(0.624325079342602,0.626198664785115),
 .UNSPECIFIED.);
#1116=B_SPLINE_CURVE_WITH_KNOTS('',3,(#23818,#23819,#23820,#23821,#23822,
#23823,#23824,#23825,#23826,#23827,#23828,#23829,#23830),.UNSPECIFIED.,
 .F.,.F.,(4,3,3,3,4),(-0.624325079343337,-0.380129337103437,-0.301935532403907,
-0.237254059228539,-0.209869946944685),.UNSPECIFIED.);
#1117=B_SPLINE_CURVE_WITH_KNOTS('',3,(#23833,#23834,#23835,#23836,#23837,
#23838,#23839,#23840,#23841,#23842),.UNSPECIFIED.,.F.,.F.,(4,2,2,2,4),(0.209869946944685,
0.237254059228639,0.301935532404242,0.380129337104056,0.624325079343485),
 .UNSPECIFIED.);
#1118=B_SPLINE_CURVE_WITH_KNOTS('',3,(#23860,#23861,#23862,#23863),
 .UNSPECIFIED.,.F.,.F.,(4,4),(0.626198664785115,0.626730655849092),
 .UNSPECIFIED.);
#1119=B_SPLINE_CURVE_WITH_KNOTS('',3,(#23865,#23866,#23867,#23868),
 .UNSPECIFIED.,.F.,.F.,(4,4),(0.,0.40461689765448),.UNSPECIFIED.);
#1120=B_SPLINE_CURVE_WITH_KNOTS('',3,(#23870,#23871,#23872,#23873),
 .UNSPECIFIED.,.F.,.F.,(4,4),(0.40461689765448,1.),.UNSPECIFIED.);
#1121=B_SPLINE_CURVE_WITH_KNOTS('',3,(#23874,#23875,#23876,#23877),
 .UNSPECIFIED.,.F.,.F.,(4,4),(-0.626730655849168,-0.626198664785115),
 .UNSPECIFIED.);
#1122=B_SPLINE_CURVE_WITH_KNOTS('',3,(#23881,#23882,#23883,#23884,#23885,
#23886,#23887,#23888,#23889,#23890,#23891,#23892),.UNSPECIFIED.,.F.,.F.,
(4,2,2,2,2,4),(0.138038496450912,0.161248355370673,0.204799871014317,0.238374998155151,
0.276615810149267,0.305604882133989),.UNSPECIFIED.);
#1123=B_SPLINE_CURVE_WITH_KNOTS('',3,(#23914,#23915,#23916,#23917),
 .UNSPECIFIED.,.F.,.F.,(4,4),(-1.50825556499841,-1.48736624018428),
 .UNSPECIFIED.);
#1124=B_SPLINE_CURVE_WITH_KNOTS('',3,(#23918,#23919,#23920,#23921),
 .UNSPECIFIED.,.F.,.F.,(4,4),(1.48736624018428,1.50825556499841),
 .UNSPECIFIED.);
#1125=B_SPLINE_CURVE_WITH_KNOTS('',3,(#23939,#23940,#23941,#23942),
 .UNSPECIFIED.,.F.,.F.,(4,4),(0.,1.),.UNSPECIFIED.);
#1126=B_SPLINE_CURVE_WITH_KNOTS('',3,(#23943,#23944,#23945,#23946),
 .UNSPECIFIED.,.F.,.F.,(4,4),(-1.,0.),.UNSPECIFIED.);
#1127=B_SPLINE_CURVE_WITH_KNOTS('',3,(#23949,#23950,#23951,#23952,#23953,
#23954,#23955,#23956,#23957,#23958),.UNSPECIFIED.,.F.,.F.,(4,2,2,2,4),(0.332744846717523,
0.350102619564171,0.400216488498811,0.450330357433451,0.50044422636809),
 .UNSPECIFIED.);
#1128=B_SPLINE_CURVE_WITH_KNOTS('',3,(#23962,#23963,#23964,#23965,#23966,
#23967,#23968,#23969,#23970,#23971,#23972,#23973,#23974,#23975,#23976,#23977),
 .UNSPECIFIED.,.F.,.F.,(4,2,2,2,2,2,2,4),(0.,0.00679055346363672,0.0146345859059421,
0.0291055700835612,0.0660529231384144,0.0914869265287218,0.111277934482435,
0.124254482609582),.UNSPECIFIED.);
#1129=B_SPLINE_CURVE_WITH_KNOTS('',3,(#24003,#24004,#24005,#24006),
 .UNSPECIFIED.,.F.,.F.,(4,4),(-1.,0.),.UNSPECIFIED.);
#1130=B_SPLINE_CURVE_WITH_KNOTS('',3,(#24008,#24009,#24010,#24011,#24012),
 .UNSPECIFIED.,.F.,.F.,(4,1,4),(0.,0.000208214441420064,0.000485833696646816),
 .UNSPECIFIED.);
#1131=B_SPLINE_CURVE_WITH_KNOTS('',3,(#24014,#24015,#24016,#24017),
 .UNSPECIFIED.,.F.,.F.,(4,4),(-1.,-0.37748786671169),.UNSPECIFIED.);
#1132=B_SPLINE_CURVE_WITH_KNOTS('',3,(#24019,#24020,#24021,#24022),
 .UNSPECIFIED.,.F.,.F.,(4,4),(-0.37748786671169,0.),.UNSPECIFIED.);
#1133=B_SPLINE_CURVE_WITH_KNOTS('',3,(#24023,#24024,#24025,#24026,#24027),
 .UNSPECIFIED.,.F.,.F.,(4,1,4),(-0.000485833696646816,-0.000208214441420064,
0.),.UNSPECIFIED.);
#1134=B_SPLINE_CURVE_WITH_KNOTS('',3,(#24052,#24053,#24054,#24055),
 .UNSPECIFIED.,.F.,.F.,(4,4),(-1.,0.),.UNSPECIFIED.);
#1135=B_SPLINE_CURVE_WITH_KNOTS('',3,(#24111,#24112,#24113,#24114,#24115,
#24116,#24117,#24118,#24119,#24120,#24121,#24122),.UNSPECIFIED.,.F.,.F.,
(4,2,2,2,2,4),(0.00166298225714781,0.120337282444558,0.218409540651057,
0.287813854984672,0.345224711421131,0.369530672027591),.UNSPECIFIED.);
#1136=B_SPLINE_CURVE_WITH_KNOTS('',3,(#24125,#24126,#24127,#24128,#24129,
#24130,#24131,#24132,#24133,#24134,#24135,#24136),.UNSPECIFIED.,.F.,.F.,
(4,2,2,2,2,4),(-0.369530672027591,-0.345224711421131,-0.287813854984672,
-0.218409540651057,-0.120337282444558,-0.00166298225714781),
 .UNSPECIFIED.);
#1137=B_SPLINE_CURVE_WITH_KNOTS('',3,(#24144,#24145,#24146,#24147,#24148,
#24149,#24150,#24151,#24152,#24153,#24154,#24155),.UNSPECIFIED.,.F.,.F.,
(4,2,2,2,2,4),(0.519582720249636,0.548571792234358,0.586812604228477,0.620387731369311,
0.663939247012956,0.687149105932712),.UNSPECIFIED.);
#1138=B_SPLINE_CURVE_WITH_KNOTS('',3,(#24173,#24174,#24175,#24176),
 .UNSPECIFIED.,.F.,.F.,(4,4),(4.77492974218118,4.7958190669953),
 .UNSPECIFIED.);
#1139=B_SPLINE_CURVE_WITH_KNOTS('',3,(#24177,#24178,#24179,#24180),
 .UNSPECIFIED.,.F.,.F.,(4,4),(-4.7958190669953,-4.77492974218118),
 .UNSPECIFIED.);
#1140=B_SPLINE_CURVE_WITH_KNOTS('',3,(#24198,#24199,#24200,#24201),
 .UNSPECIFIED.,.F.,.F.,(4,4),(0.,1.),.UNSPECIFIED.);
#1141=B_SPLINE_CURVE_WITH_KNOTS('',3,(#24202,#24203,#24204,#24205),
 .UNSPECIFIED.,.F.,.F.,(4,4),(-1.,0.),.UNSPECIFIED.);
#1142=B_SPLINE_CURVE_WITH_KNOTS('',3,(#24301,#24302,#24303,#24304,#24305,
#24306,#24307,#24308,#24309,#24310,#24311,#24312,#24313,#24314),
 .UNSPECIFIED.,.F.,.F.,(4,1,1,1,1,1,1,1,1,1,1,4),(-2.80995821199303,-2.67614471704543,
-2.54233748119315,-2.40853024534088,-2.14091577363634,-1.96250612583331,
-1.78409647803028,-1.60568683022725,-1.42727718242423,-1.2488675346212,
-1.07045788681817,-0.936655001901496),.UNSPECIFIED.);
#1143=B_SPLINE_CURVE_WITH_KNOTS('',3,(#24317,#24318,#24319,#24320,#24321,
#24322,#24323,#24324),.UNSPECIFIED.,.F.,.F.,(4,1,1,1,1,4),(-3.74660260386359,
-3.61279536801132,-3.47898813215905,-3.21137366045451,-2.94375918874997,
-2.80995821199303),.UNSPECIFIED.);
#1144=B_SPLINE_CURVE_WITH_KNOTS('',3,(#24325,#24326,#24327,#24328,#24329,
#24330,#24331,#24332),.UNSPECIFIED.,.F.,.F.,(4,1,1,1,1,4),(-0.936655001901496,
-0.802843415113627,-0.535228943409085,-0.267614471704543,-0.133807235852271,
0.),.UNSPECIFIED.);
#1145=B_SPLINE_CURVE_WITH_KNOTS('',3,(#24445,#24446,#24447,#24448,#24449,
#24450,#24451,#24452,#24453,#24454,#24455,#24456,#24457,#24458,#24459,#24460,
#24461,#24462,#24463,#24464,#24465,#24466),.UNSPECIFIED.,.T.,.F.,(4,1,1,
1,1,1,1,1,1,1,1,1,1,1,1,1,1,1,1,4),(0.,0.133807235852271,0.267614471704543,
0.535228943409085,0.802843415113627,1.07045788681817,1.2488675346212,1.42727718242423,
1.60568683022725,1.78409647803028,1.96250612583331,2.14091577363634,2.40853024534088,
2.54233748119315,2.67614471704543,2.94375918874997,3.21137366045451,3.47898813215905,
3.61279536801132,3.74660260386359),.UNSPECIFIED.);
#1146=B_SPLINE_CURVE_WITH_KNOTS('',3,(#24478,#24479,#24480,#24481,#24482,
#24483,#24484,#24485,#24486,#24487,#24488,#24489,#24490,#24491),
 .UNSPECIFIED.,.F.,.F.,(4,2,2,2,2,2,4),(-0.345305288041167,-0.344620712595134,
-0.226569517485857,-0.15131577954814,-0.0758841034235322,-0.030282394435752,
0.),.UNSPECIFIED.);
#1147=B_SPLINE_CURVE_WITH_KNOTS('',3,(#24505,#24506,#24507,#24508,#24509,
#24510,#24511,#24512,#24513,#24514,#24515,#24516,#24517,#24518),
 .UNSPECIFIED.,.F.,.F.,(4,2,2,2,2,2,4),(-0.422554374321187,-0.385423821412686,
-0.329509594686649,-0.237019555721844,-0.144747694460498,0.,0.000839387766042462),
 .UNSPECIFIED.);
#1148=B_SPLINE_CURVE_WITH_KNOTS('',3,(#24531,#24532,#24533,#24534,#24535,
#24536,#24537,#24538,#24539,#24540,#24541,#24542,#24543,#24544),
 .UNSPECIFIED.,.F.,.F.,(4,2,2,2,2,2,4),(-0.345305322448276,-0.344620746646918,
-0.22656951748443,-0.151315779547605,-0.0758841034234829,-0.030282394435745,
0.),.UNSPECIFIED.);
#1149=B_SPLINE_CURVE_WITH_KNOTS('',3,(#24566,#24567,#24568,#24569,#24570,
#24571,#24572,#24573,#24574,#24575,#24576,#24577,#24578,#24579),
 .UNSPECIFIED.,.F.,.F.,(4,2,2,2,2,2,4),(-0.351506503283319,-0.286559194099349,
-0.217668322783822,-0.136952361437555,-0.0679759511705759,0.,0.000711948788676417),
 .UNSPECIFIED.);
#1150=B_SPLINE_CURVE_WITH_KNOTS('',3,(#24594,#24595,#24596,#24597,#24598,
#24599,#24600,#24601,#24602,#24603,#24604,#24605,#24606,#24607),
 .UNSPECIFIED.,.F.,.F.,(4,2,2,2,2,2,4),(-0.350131750560411,-0.349424019690355,
-0.281850788688661,-0.213283025920958,-0.133045262492339,-0.0645625319046002,
0.),.UNSPECIFIED.);
#1151=B_SPLINE_CURVE_WITH_KNOTS('',3,(#24767,#24768,#24769,#24770,#24771,
#24772,#24773,#24774,#24775,#24776,#24777,#24778,#24779,#24780,#24781,#24782,
#24783,#24784,#24785,#24786,#24787,#24788,#24789,#24790,#24791,#24792,#24793,
#24794,#24795,#24796,#24797,#24798,#24799,#24800,#24801,#24802,#24803,#24804,
#24805,#24806,#24807,#24808,#24809,#24810,#24811,#24812,#24813,#24814,#24815,
#24816,#24817,#24818,#24819,#24820,#24821,#24822,#24823,#24824,#24825,#24826,
#24827,#24828,#24829,#24830,#24831,#24832,#24833,#24834,#24835,#24836,#24837,
#24838,#24839,#24840,#24841,#24842,#24843,#24844,#24845,#24846,#24847,#24848,
#24849,#24850,#24851,#24852,#24853,#24854,#24855,#24856,#24857,#24858,#24859,
#24860,#24861,#24862,#24863,#24864,#24865,#24866,#24867,#24868,#24869,#24870,
#24871,#24872,#24873,#24874,#24875,#24876,#24877,#24878,#24879,#24880,#24881,
#24882,#24883,#24884,#24885,#24886,#24887,#24888,#24889,#24890,#24891,#24892,
#24893,#24894,#24895,#24896,#24897,#24898,#24899,#24900,#24901,#24902,#24903,
#24904,#24905,#24906,#24907,#24908,#24909,#24910,#24911,#24912,#24913,#24914,
#24915,#24916,#24917,#24918,#24919,#24920,#24921,#24922,#24923,#24924,#24925,
#24926,#24927,#24928,#24929,#24930,#24931,#24932,#24933,#24934,#24935,#24936,
#24937,#24938,#24939,#24940,#24941,#24942,#24943,#24944,#24945,#24946,#24947,
#24948,#24949,#24950,#24951,#24952,#24953,#24954,#24955,#24956,#24957,#24958,
#24959,#24960,#24961,#24962,#24963,#24964,#24965,#24966,#24967,#24968,#24969,
#24970,#24971,#24972,#24973,#24974,#24975,#24976,#24977,#24978,#24979,#24980,
#24981,#24982,#24983,#24984,#24985,#24986,#24987,#24988,#24989,#24990,#24991,
#24992,#24993,#24994,#24995,#24996,#24997,#24998,#24999,#25000,#25001,#25002,
#25003,#25004,#25005,#25006,#25007,#25008,#25009,#25010,#25011,#25012,#25013,
#25014,#25015,#25016,#25017,#25018,#25019),.UNSPECIFIED.,.F.,.F.,(4,3,3,
3,3,3,3,3,3,3,3,3,3,3,3,3,3,3,3,3,3,3,3,3,3,3,3,3,3,3,3,3,3,3,3,3,3,3,3,
3,3,3,3,3,3,3,3,3,3,3,3,3,3,3,3,3,3,3,3,3,3,3,3,3,3,3,3,3,3,3,3,3,3,3,3,
3,3,3,3,3,3,3,3,3,4),(0.,0.0813280369871104,0.10426271137412,0.17724565415719,
0.248684089577596,0.320122524998002,0.388171850673652,0.45433223954272,
0.496422333197618,0.555732946496683,0.613636795430242,0.640021394627608,
0.696656237449289,0.753087155105956,0.808915529598096,0.836983440014268,
0.892384452514873,0.947440153385303,0.95982385581978,1.01461986638795,1.06994040744583,
1.12583018879548,1.17176297454938,1.23015322407112,1.27982518853794,1.33869000601364,
1.39774705874962,1.4567876494499,1.49291289003645,1.55328529142365,1.5998485198889,
1.66004066589129,1.71941954967881,1.77418606762871,1.83221046372469,1.88941828995785,
1.91970052834762,1.9760468885945,2.032160295288,2.08764355038908,2.11139064429874,
2.13283348679512,2.18717034576841,2.24227858706577,2.29844665483361,2.35506564452401,
2.41206805172476,2.44465988147568,2.51246843122597,2.55981452659546,2.62802745211438,
2.70048101976627,2.77293458741816,2.82461261529351,2.88939162661952,2.95507054101926,
2.98614701351453,3.05100710484421,3.10476710153347,3.17625736575752,3.19959679788099,
3.26972372420938,3.3376297735848,3.40411528115335,3.46846403910524,3.51930648273169,
3.5202225802945,3.57838132493156,3.63653714411098,3.69409893873786,3.75108640250181,
3.80705542924498,3.83890564683775,3.87319766720952,3.93090365877466,3.98960105332232,
4.04855689348964,4.10738895498192,4.15897712336674,4.21313376356879,4.27400032548969,
4.33648185529254,4.39979751513143,4.46403159890671,4.47914967830435),
 .UNSPECIFIED.);
#1152=B_SPLINE_CURVE_WITH_KNOTS('',3,(#25069,#25070,#25071,#25072,#25073,
#25074,#25075,#25076),.UNSPECIFIED.,.F.,.F.,(4,1,1,1,1,4),(0.,0.213141959635737,
0.426283919271474,0.852567838542947,1.06570979817868,1.49199371745016),
 .UNSPECIFIED.);
#1153=B_SPLINE_CURVE_WITH_KNOTS('',3,(#25084,#25085,#25086,#25087,#25088,
#25089,#25090,#25091,#25092,#25093,#25094,#25095,#25096,#25097),
 .UNSPECIFIED.,.F.,.F.,(4,2,2,2,2,2,4),(0.37662094331532,0.433515090571885,
0.499087916949629,0.586028073495358,0.673570485757201,0.765226500919176,
0.766118331324739),.UNSPECIFIED.);
#1154=B_SPLINE_CURVE_WITH_KNOTS('',3,(#25108,#25109,#25110,#25111,#25112,
#25113,#25114,#25115,#25116,#25117,#25118,#25119,#25120,#25121,#25122,#25123,
#25124,#25125,#25126,#25127),.UNSPECIFIED.,.F.,.F.,(4,2,2,2,2,2,2,2,2,4),
(0.422785857755809,0.43703384117159,0.463320009434893,0.49635128790697,
0.541631933053045,0.566268869107166,0.583621071618297,0.593824785751523,
0.601681049890584,0.601998413219366),.UNSPECIFIED.);
#1155=B_SPLINE_CURVE_WITH_KNOTS('',3,(#25131,#25132,#25133,#25134,#25135,
#25136,#25137,#25138,#25139,#25140,#25141,#25142,#25143,#25144),
 .UNSPECIFIED.,.F.,.F.,(4,2,2,2,2,2,4),(-0.000892803052402962,0.,0.0917559770331036,
0.179393864789738,0.266428839998198,0.3320731814037,0.38902937854808),
 .UNSPECIFIED.);
#1156=B_SPLINE_CURVE_WITH_KNOTS('',3,(#25158,#25159,#25160,#25161,#25162,
#25163,#25164,#25165,#25166,#25167,#25168,#25169,#25170,#25171),
 .UNSPECIFIED.,.F.,.F.,(4,2,2,2,2,2,4),(0.376620943315501,0.433515090572235,
0.499087916950171,0.586028073496191,0.673570485758674,0.765226500920609,
0.766118331324419),.UNSPECIFIED.);
#1157=B_SPLINE_CURVE_WITH_KNOTS('',3,(#25175,#25176,#25177,#25178,#25179,
#25180,#25181,#25182,#25183,#25184,#25185,#25186,#25187,#25188),
 .UNSPECIFIED.,.F.,.F.,(4,2,2,2,2,2,4),(-0.00089280305197105,0.,0.0917559770332232,
0.17939386478995,0.266428839998158,0.332073181403452,0.389029378547644),
 .UNSPECIFIED.);
#1158=B_SPLINE_CURVE_WITH_KNOTS('',3,(#25201,#25202,#25203,#25204,#25205,
#25206,#25207,#25208,#25209,#25210,#25211,#25212,#25213,#25214),
 .UNSPECIFIED.,.F.,.F.,(4,2,2,2,2,2,4),(0.376620943315551,0.433515090572292,
0.499087916950247,0.586028073496283,0.673570485758794,0.765226500920732,
0.766118331324744),.UNSPECIFIED.);
#1159=B_SPLINE_CURVE_WITH_KNOTS('',3,(#25218,#25219,#25220,#25221,#25222,
#25223,#25224,#25225,#25226,#25227,#25228,#25229,#25230,#25231),
 .UNSPECIFIED.,.F.,.F.,(4,2,2,2,2,2,4),(-0.000892803051768479,0.,0.0917559770332231,
0.179393864789949,0.266428839998158,0.332073181403451,0.389029378547642),
 .UNSPECIFIED.);
#1160=B_SPLINE_CURVE_WITH_KNOTS('',3,(#25301,#25302,#25303,#25304,#25305,
#25306,#25307,#25308,#25309,#25310),.UNSPECIFIED.,.F.,.F.,(4,2,2,2,4),(0.500444226368088,
0.550558095302727,0.600671964237367,0.650785833172007,0.66814360601866),
 .UNSPECIFIED.);
#1161=B_SPLINE_CURVE_WITH_KNOTS('',3,(#25316,#25317,#25318,#25319,#25320,
#25321,#25322,#25323,#25324,#25325,#25326,#25327,#25328,#25329),
 .UNSPECIFIED.,.F.,.F.,(4,2,2,2,2,2,4),(-0.422554267641051,-0.385423725942617,
-0.329509516097576,-0.237019505055533,-0.1447476716502,0.,0.000839387731405013),
 .UNSPECIFIED.);
#1409=CYLINDRICAL_SURFACE('',#15501,13.);
#1410=CYLINDRICAL_SURFACE('',#15511,19.);
#1411=CYLINDRICAL_SURFACE('',#15520,2.);
#1412=CYLINDRICAL_SURFACE('',#15523,6.05);
#1413=CYLINDRICAL_SURFACE('',#15531,2.);
#1414=CYLINDRICAL_SURFACE('',#15534,6.05);
#1415=CYLINDRICAL_SURFACE('',#15542,6.05);
#1416=CYLINDRICAL_SURFACE('',#15550,2.);
#1417=CYLINDRICAL_SURFACE('',#15553,6.05);
#1418=CYLINDRICAL_SURFACE('',#15558,2.);
#1419=CYLINDRICAL_SURFACE('',#15585,5.05000000000001);
#1420=CYLINDRICAL_SURFACE('',#15589,5.04999999999999);
#1421=CYLINDRICAL_SURFACE('',#15593,5.04999999999999);
#1422=CYLINDRICAL_SURFACE('',#15597,5.05000000000001);
#1423=CYLINDRICAL_SURFACE('',#15601,9.49999999999999);
#1424=CYLINDRICAL_SURFACE('',#15604,6.);
#1425=CYLINDRICAL_SURFACE('',#15606,2.);
#1426=CYLINDRICAL_SURFACE('',#15612,2.);
#1427=CYLINDRICAL_SURFACE('',#15614,2.);
#1428=CYLINDRICAL_SURFACE('',#15615,2.);
#1429=CYLINDRICAL_SURFACE('',#15619,2.);
#1430=CYLINDRICAL_SURFACE('',#15624,2.);
#1431=CYLINDRICAL_SURFACE('',#15626,2.);
#1432=CYLINDRICAL_SURFACE('',#15633,2.);
#1433=CYLINDRICAL_SURFACE('',#15634,2.);
#1434=CYLINDRICAL_SURFACE('',#15640,2.);
#1435=CYLINDRICAL_SURFACE('',#15641,2.);
#1436=CYLINDRICAL_SURFACE('',#15658,43.05);
#1437=CYLINDRICAL_SURFACE('',#15663,2.);
#1438=CYLINDRICAL_SURFACE('',#15681,28.);
#1439=CYLINDRICAL_SURFACE('',#15700,2.);
#1440=CYLINDRICAL_SURFACE('',#15706,28.);
#1441=CYLINDRICAL_SURFACE('',#15714,2.);
#1442=CYLINDRICAL_SURFACE('',#15728,2.);
#1443=CYLINDRICAL_SURFACE('',#15729,28.);
#1444=CYLINDRICAL_SURFACE('',#15732,28.);
#1445=CYLINDRICAL_SURFACE('',#15733,2.);
#1446=CYLINDRICAL_SURFACE('',#15735,2.);
#1447=CYLINDRICAL_SURFACE('',#15740,2.);
#1448=CYLINDRICAL_SURFACE('',#15741,2.);
#1449=CYLINDRICAL_SURFACE('',#15743,10.);
#1450=CYLINDRICAL_SURFACE('',#15758,2.);
#1451=CYLINDRICAL_SURFACE('',#15761,2.);
#1452=CYLINDRICAL_SURFACE('',#15765,2.);
#1453=CYLINDRICAL_SURFACE('',#15767,2.);
#1454=CYLINDRICAL_SURFACE('',#15768,10.);
#1455=CYLINDRICAL_SURFACE('',#15773,2.);
#1456=CYLINDRICAL_SURFACE('',#15774,6.5);
#1457=CYLINDRICAL_SURFACE('',#15775,6.5);
#1458=CYLINDRICAL_SURFACE('',#15777,6.5);
#1459=CYLINDRICAL_SURFACE('',#15778,6.5);
#1460=CYLINDRICAL_SURFACE('',#15779,10.);
#1461=CYLINDRICAL_SURFACE('',#15781,10.);
#1462=CYLINDRICAL_SURFACE('',#15792,16.6);
#1463=CYLINDRICAL_SURFACE('',#15796,16.505);
#1737=FACE_OUTER_BOUND('',#2642,.T.);
#1738=FACE_OUTER_BOUND('',#2643,.T.);
#1739=FACE_OUTER_BOUND('',#2645,.T.);
#1740=FACE_OUTER_BOUND('',#2646,.T.);
#1741=FACE_OUTER_BOUND('',#2647,.T.);
#1742=FACE_OUTER_BOUND('',#2649,.T.);
#1743=FACE_OUTER_BOUND('',#2650,.T.);
#1744=FACE_OUTER_BOUND('',#2651,.T.);
#1745=FACE_OUTER_BOUND('',#2652,.T.);
#1746=FACE_OUTER_BOUND('',#2653,.T.);
#1747=FACE_OUTER_BOUND('',#2654,.T.);
#1748=FACE_OUTER_BOUND('',#2655,.T.);
#1749=FACE_OUTER_BOUND('',#2656,.T.);
#1750=FACE_OUTER_BOUND('',#2657,.T.);
#1751=FACE_OUTER_BOUND('',#2658,.T.);
#1752=FACE_OUTER_BOUND('',#2659,.T.);
#1753=FACE_OUTER_BOUND('',#2660,.T.);
#1754=FACE_OUTER_BOUND('',#2661,.T.);
#1755=FACE_OUTER_BOUND('',#2662,.T.);
#1756=FACE_OUTER_BOUND('',#2663,.T.);
#1757=FACE_OUTER_BOUND('',#2664,.T.);
#1758=FACE_OUTER_BOUND('',#2665,.T.);
#1759=FACE_OUTER_BOUND('',#2666,.T.);
#1760=FACE_OUTER_BOUND('',#2667,.T.);
#1761=FACE_OUTER_BOUND('',#2668,.T.);
#1762=FACE_OUTER_BOUND('',#2669,.T.);
#1763=FACE_OUTER_BOUND('',#2670,.T.);
#1764=FACE_OUTER_BOUND('',#2671,.T.);
#1765=FACE_OUTER_BOUND('',#2672,.T.);
#1766=FACE_OUTER_BOUND('',#2673,.T.);
#1767=FACE_OUTER_BOUND('',#2674,.T.);
#1768=FACE_OUTER_BOUND('',#2675,.T.);
#1769=FACE_OUTER_BOUND('',#2676,.T.);
#1770=FACE_OUTER_BOUND('',#2677,.T.);
#1771=FACE_OUTER_BOUND('',#2678,.T.);
#1772=FACE_OUTER_BOUND('',#2679,.T.);
#1773=FACE_OUTER_BOUND('',#2680,.T.);
#1774=FACE_OUTER_BOUND('',#2681,.T.);
#1775=FACE_OUTER_BOUND('',#2682,.T.);
#1776=FACE_OUTER_BOUND('',#2683,.T.);
#1777=FACE_OUTER_BOUND('',#2684,.T.);
#1778=FACE_OUTER_BOUND('',#2685,.T.);
#1779=FACE_OUTER_BOUND('',#2686,.T.);
#1780=FACE_OUTER_BOUND('',#2687,.T.);
#1781=FACE_OUTER_BOUND('',#2688,.T.);
#1782=FACE_OUTER_BOUND('',#2689,.T.);
#1783=FACE_OUTER_BOUND('',#2690,.T.);
#1784=FACE_OUTER_BOUND('',#2691,.T.);
#1785=FACE_OUTER_BOUND('',#2692,.T.);
#1786=FACE_OUTER_BOUND('',#2693,.T.);
#1787=FACE_OUTER_BOUND('',#2694,.T.);
#1788=FACE_OUTER_BOUND('',#2695,.T.);
#1789=FACE_OUTER_BOUND('',#2696,.T.);
#1790=FACE_OUTER_BOUND('',#2697,.T.);
#1791=FACE_OUTER_BOUND('',#2698,.T.);
#1792=FACE_OUTER_BOUND('',#2699,.T.);
#1793=FACE_OUTER_BOUND('',#2700,.T.);
#1794=FACE_OUTER_BOUND('',#2701,.T.);
#1795=FACE_OUTER_BOUND('',#2702,.T.);
#1796=FACE_OUTER_BOUND('',#2703,.T.);
#1797=FACE_OUTER_BOUND('',#2704,.T.);
#1798=FACE_OUTER_BOUND('',#2705,.T.);
#1799=FACE_OUTER_BOUND('',#2706,.T.);
#1800=FACE_OUTER_BOUND('',#2707,.T.);
#1801=FACE_OUTER_BOUND('',#2708,.T.);
#1802=FACE_OUTER_BOUND('',#2714,.T.);
#1803=FACE_OUTER_BOUND('',#2715,.T.);
#1804=FACE_OUTER_BOUND('',#2716,.T.);
#1805=FACE_OUTER_BOUND('',#2717,.T.);
#1806=FACE_OUTER_BOUND('',#2718,.T.);
#1807=FACE_OUTER_BOUND('',#2719,.T.);
#1808=FACE_OUTER_BOUND('',#2720,.T.);
#1809=FACE_OUTER_BOUND('',#2721,.T.);
#1810=FACE_OUTER_BOUND('',#2722,.T.);
#1811=FACE_OUTER_BOUND('',#2723,.T.);
#1812=FACE_OUTER_BOUND('',#2724,.T.);
#1813=FACE_OUTER_BOUND('',#2725,.T.);
#1814=FACE_OUTER_BOUND('',#2726,.T.);
#1815=FACE_OUTER_BOUND('',#2727,.T.);
#1816=FACE_OUTER_BOUND('',#2728,.T.);
#1817=FACE_OUTER_BOUND('',#2729,.T.);
#1818=FACE_OUTER_BOUND('',#2730,.T.);
#1819=FACE_OUTER_BOUND('',#2731,.T.);
#1820=FACE_OUTER_BOUND('',#2732,.T.);
#1821=FACE_OUTER_BOUND('',#2733,.T.);
#1822=FACE_OUTER_BOUND('',#2734,.T.);
#1823=FACE_OUTER_BOUND('',#2735,.T.);
#1824=FACE_OUTER_BOUND('',#2736,.T.);
#1825=FACE_OUTER_BOUND('',#2737,.T.);
#1826=FACE_OUTER_BOUND('',#2738,.T.);
#1827=FACE_OUTER_BOUND('',#2739,.T.);
#1828=FACE_OUTER_BOUND('',#2740,.T.);
#1829=FACE_OUTER_BOUND('',#2741,.T.);
#1830=FACE_OUTER_BOUND('',#2742,.T.);
#1831=FACE_OUTER_BOUND('',#2743,.T.);
#1832=FACE_OUTER_BOUND('',#2744,.T.);
#1833=FACE_OUTER_BOUND('',#2745,.T.);
#1834=FACE_OUTER_BOUND('',#2746,.T.);
#1835=FACE_OUTER_BOUND('',#2752,.T.);
#1836=FACE_OUTER_BOUND('',#2753,.T.);
#1837=FACE_OUTER_BOUND('',#2754,.T.);
#1838=FACE_OUTER_BOUND('',#2755,.T.);
#1839=FACE_OUTER_BOUND('',#2756,.T.);
#1840=FACE_OUTER_BOUND('',#2757,.T.);
#1841=FACE_OUTER_BOUND('',#2758,.T.);
#1842=FACE_OUTER_BOUND('',#2759,.T.);
#1843=FACE_OUTER_BOUND('',#2763,.T.);
#1844=FACE_OUTER_BOUND('',#2764,.T.);
#1845=FACE_OUTER_BOUND('',#2766,.T.);
#1846=FACE_OUTER_BOUND('',#2767,.T.);
#1847=FACE_OUTER_BOUND('',#2768,.T.);
#1848=FACE_OUTER_BOUND('',#2769,.T.);
#1849=FACE_OUTER_BOUND('',#2771,.T.);
#1850=FACE_OUTER_BOUND('',#2772,.T.);
#1851=FACE_OUTER_BOUND('',#2774,.T.);
#1852=FACE_OUTER_BOUND('',#2775,.T.);
#1853=FACE_OUTER_BOUND('',#2776,.T.);
#1854=FACE_OUTER_BOUND('',#2777,.T.);
#1855=FACE_OUTER_BOUND('',#2778,.T.);
#1856=FACE_OUTER_BOUND('',#2779,.T.);
#1857=FACE_OUTER_BOUND('',#2780,.T.);
#1858=FACE_OUTER_BOUND('',#2781,.T.);
#1859=FACE_OUTER_BOUND('',#2782,.T.);
#1860=FACE_OUTER_BOUND('',#2783,.T.);
#1861=FACE_OUTER_BOUND('',#2784,.T.);
#1862=FACE_OUTER_BOUND('',#2785,.T.);
#1863=FACE_OUTER_BOUND('',#2786,.T.);
#1864=FACE_OUTER_BOUND('',#2787,.T.);
#1865=FACE_OUTER_BOUND('',#2788,.T.);
#1866=FACE_OUTER_BOUND('',#2789,.T.);
#1867=FACE_OUTER_BOUND('',#2790,.T.);
#1868=FACE_OUTER_BOUND('',#2791,.T.);
#1869=FACE_OUTER_BOUND('',#2792,.T.);
#1870=FACE_OUTER_BOUND('',#2793,.T.);
#1871=FACE_OUTER_BOUND('',#2794,.T.);
#1872=FACE_OUTER_BOUND('',#2795,.T.);
#1873=FACE_OUTER_BOUND('',#2796,.T.);
#1874=FACE_OUTER_BOUND('',#2797,.T.);
#1875=FACE_OUTER_BOUND('',#2798,.T.);
#1876=FACE_OUTER_BOUND('',#2799,.T.);
#1877=FACE_OUTER_BOUND('',#2800,.T.);
#1878=FACE_OUTER_BOUND('',#2801,.T.);
#1879=FACE_OUTER_BOUND('',#2802,.T.);
#1880=FACE_OUTER_BOUND('',#2803,.T.);
#1881=FACE_OUTER_BOUND('',#2804,.T.);
#1882=FACE_OUTER_BOUND('',#2805,.T.);
#1883=FACE_OUTER_BOUND('',#2806,.T.);
#1884=FACE_OUTER_BOUND('',#2807,.T.);
#1885=FACE_OUTER_BOUND('',#2808,.T.);
#1886=FACE_OUTER_BOUND('',#2809,.T.);
#1887=FACE_OUTER_BOUND('',#2810,.T.);
#1888=FACE_OUTER_BOUND('',#2811,.T.);
#1889=FACE_OUTER_BOUND('',#2812,.T.);
#1890=FACE_OUTER_BOUND('',#2813,.T.);
#1891=FACE_OUTER_BOUND('',#2814,.T.);
#1892=FACE_OUTER_BOUND('',#2815,.T.);
#1893=FACE_OUTER_BOUND('',#2816,.T.);
#1894=FACE_OUTER_BOUND('',#2817,.T.);
#1895=FACE_OUTER_BOUND('',#2819,.T.);
#1896=FACE_OUTER_BOUND('',#2820,.T.);
#1897=FACE_OUTER_BOUND('',#2821,.T.);
#1898=FACE_OUTER_BOUND('',#2822,.T.);
#1899=FACE_OUTER_BOUND('',#2823,.T.);
#1900=FACE_OUTER_BOUND('',#2824,.T.);
#1901=FACE_OUTER_BOUND('',#2825,.T.);
#1902=FACE_OUTER_BOUND('',#2826,.T.);
#1903=FACE_OUTER_BOUND('',#2827,.T.);
#1904=FACE_OUTER_BOUND('',#2828,.T.);
#1905=FACE_OUTER_BOUND('',#2829,.T.);
#1906=FACE_OUTER_BOUND('',#2830,.T.);
#1907=FACE_OUTER_BOUND('',#2831,.T.);
#1908=FACE_OUTER_BOUND('',#2833,.T.);
#1909=FACE_OUTER_BOUND('',#2834,.T.);
#1910=FACE_OUTER_BOUND('',#2835,.T.);
#2642=EDGE_LOOP('',(#10371,#10372,#10373,#10374,#10375));
#2643=EDGE_LOOP('',(#10376));
#2644=EDGE_LOOP('',(#10377));
#2645=EDGE_LOOP('',(#10378,#10379,#10380,#10381,#10382));
#2646=EDGE_LOOP('',(#10383,#10384,#10385,#10386));
#2647=EDGE_LOOP('',(#10387,#10388,#10389,#10390,#10391,#10392,#10393,#10394));
#2648=EDGE_LOOP('',(#10395));
#2649=EDGE_LOOP('',(#10396,#10397,#10398,#10399,#10400,#10401,#10402));
#2650=EDGE_LOOP('',(#10403,#10404,#10405,#10406,#10407));
#2651=EDGE_LOOP('',(#10408,#10409,#10410,#10411));
#2652=EDGE_LOOP('',(#10412,#10413,#10414,#10415));
#2653=EDGE_LOOP('',(#10416,#10417,#10418,#10419));
#2654=EDGE_LOOP('',(#10420,#10421,#10422,#10423));
#2655=EDGE_LOOP('',(#10424,#10425,#10426,#10427));
#2656=EDGE_LOOP('',(#10428,#10429,#10430,#10431));
#2657=EDGE_LOOP('',(#10432,#10433,#10434,#10435));
#2658=EDGE_LOOP('',(#10436,#10437,#10438));
#2659=EDGE_LOOP('',(#10439,#10440,#10441,#10442,#10443,#10444,#10445,#10446,
#10447,#10448,#10449,#10450));
#2660=EDGE_LOOP('',(#10451,#10452,#10453,#10454,#10455,#10456,#10457,#10458,
#10459,#10460,#10461,#10462));
#2661=EDGE_LOOP('',(#10463,#10464,#10465,#10466));
#2662=EDGE_LOOP('',(#10467,#10468,#10469,#10470,#10471));
#2663=EDGE_LOOP('',(#10472,#10473,#10474,#10475));
#2664=EDGE_LOOP('',(#10476,#10477,#10478,#10479));
#2665=EDGE_LOOP('',(#10480,#10481,#10482,#10483));
#2666=EDGE_LOOP('',(#10484,#10485,#10486,#10487));
#2667=EDGE_LOOP('',(#10488,#10489,#10490,#10491));
#2668=EDGE_LOOP('',(#10492,#10493,#10494,#10495));
#2669=EDGE_LOOP('',(#10496,#10497,#10498));
#2670=EDGE_LOOP('',(#10499,#10500,#10501,#10502,#10503,#10504,#10505,#10506,
#10507,#10508,#10509,#10510));
#2671=EDGE_LOOP('',(#10511,#10512,#10513,#10514,#10515,#10516,#10517,#10518,
#10519,#10520,#10521,#10522));
#2672=EDGE_LOOP('',(#10523,#10524,#10525,#10526));
#2673=EDGE_LOOP('',(#10527,#10528,#10529,#10530));
#2674=EDGE_LOOP('',(#10531,#10532,#10533,#10534));
#2675=EDGE_LOOP('',(#10535,#10536,#10537,#10538,#10539));
#2676=EDGE_LOOP('',(#10540,#10541,#10542,#10543));
#2677=EDGE_LOOP('',(#10544,#10545,#10546,#10547));
#2678=EDGE_LOOP('',(#10548,#10549,#10550,#10551));
#2679=EDGE_LOOP('',(#10552,#10553,#10554,#10555));
#2680=EDGE_LOOP('',(#10556,#10557,#10558,#10559,#10560,#10561,#10562,#10563,
#10564,#10565,#10566,#10567));
#2681=EDGE_LOOP('',(#10568,#10569,#10570,#10571));
#2682=EDGE_LOOP('',(#10572,#10573,#10574,#10575));
#2683=EDGE_LOOP('',(#10576,#10577,#10578,#10579));
#2684=EDGE_LOOP('',(#10580,#10581,#10582,#10583));
#2685=EDGE_LOOP('',(#10584,#10585,#10586,#10587));
#2686=EDGE_LOOP('',(#10588,#10589,#10590,#10591,#10592));
#2687=EDGE_LOOP('',(#10593,#10594,#10595,#10596));
#2688=EDGE_LOOP('',(#10597,#10598,#10599,#10600));
#2689=EDGE_LOOP('',(#10601,#10602,#10603));
#2690=EDGE_LOOP('',(#10604,#10605,#10606,#10607,#10608,#10609,#10610,#10611,
#10612,#10613,#10614,#10615));
#2691=EDGE_LOOP('',(#10616,#10617,#10618,#10619,#10620,#10621,#10622,#10623,
#10624,#10625,#10626,#10627));
#2692=EDGE_LOOP('',(#10628,#10629,#10630,#10631));
#2693=EDGE_LOOP('',(#10632,#10633,#10634,#10635));
#2694=EDGE_LOOP('',(#10636,#10637,#10638,#10639,#10640));
#2695=EDGE_LOOP('',(#10641,#10642,#10643,#10644));
#2696=EDGE_LOOP('',(#10645,#10646,#10647,#10648));
#2697=EDGE_LOOP('',(#10649,#10650,#10651,#10652));
#2698=EDGE_LOOP('',(#10653,#10654,#10655,#10656,#10657,#10658,#10659,#10660,
#10661,#10662,#10663));
#2699=EDGE_LOOP('',(#10664,#10665,#10666,#10667,#10668));
#2700=EDGE_LOOP('',(#10669,#10670,#10671,#10672));
#2701=EDGE_LOOP('',(#10673,#10674,#10675,#10676));
#2702=EDGE_LOOP('',(#10677,#10678,#10679,#10680));
#2703=EDGE_LOOP('',(#10681,#10682,#10683,#10684));
#2704=EDGE_LOOP('',(#10685,#10686,#10687,#10688));
#2705=EDGE_LOOP('',(#10689,#10690,#10691,#10692,#10693,#10694,#10695,#10696));
#2706=EDGE_LOOP('',(#10697,#10698,#10699,#10700,#10701,#10702,#10703,#10704,
#10705,#10706,#10707,#10708,#10709,#10710,#10711,#10712,#10713,#10714,#10715,
#10716));
#2707=EDGE_LOOP('',(#10717,#10718,#10719,#10720));
#2708=EDGE_LOOP('',(#10721,#10722,#10723,#10724));
#2709=EDGE_LOOP('',(#10725));
#2710=EDGE_LOOP('',(#10726));
#2711=EDGE_LOOP('',(#10727));
#2712=EDGE_LOOP('',(#10728));
#2713=EDGE_LOOP('',(#10729));
#2714=EDGE_LOOP('',(#10730,#10731,#10732,#10733));
#2715=EDGE_LOOP('',(#10734,#10735,#10736,#10737));
#2716=EDGE_LOOP('',(#10738,#10739,#10740,#10741));
#2717=EDGE_LOOP('',(#10742,#10743,#10744,#10745));
#2718=EDGE_LOOP('',(#10746,#10747,#10748,#10749));
#2719=EDGE_LOOP('',(#10750,#10751,#10752,#10753));
#2720=EDGE_LOOP('',(#10754,#10755,#10756,#10757));
#2721=EDGE_LOOP('',(#10758,#10759,#10760,#10761));
#2722=EDGE_LOOP('',(#10762,#10763,#10764,#10765,#10766,#10767,#10768));
#2723=EDGE_LOOP('',(#10769,#10770,#10771,#10772,#10773,#10774));
#2724=EDGE_LOOP('',(#10775,#10776,#10777,#10778));
#2725=EDGE_LOOP('',(#10779,#10780,#10781,#10782));
#2726=EDGE_LOOP('',(#10783,#10784,#10785));
#2727=EDGE_LOOP('',(#10786,#10787,#10788,#10789));
#2728=EDGE_LOOP('',(#10790,#10791,#10792,#10793));
#2729=EDGE_LOOP('',(#10794,#10795,#10796,#10797));
#2730=EDGE_LOOP('',(#10798,#10799,#10800));
#2731=EDGE_LOOP('',(#10801,#10802,#10803,#10804));
#2732=EDGE_LOOP('',(#10805,#10806,#10807));
#2733=EDGE_LOOP('',(#10808,#10809,#10810,#10811));
#2734=EDGE_LOOP('',(#10812,#10813,#10814,#10815));
#2735=EDGE_LOOP('',(#10816,#10817,#10818,#10819));
#2736=EDGE_LOOP('',(#10820,#10821,#10822));
#2737=EDGE_LOOP('',(#10823,#10824,#10825));
#2738=EDGE_LOOP('',(#10826,#10827,#10828,#10829));
#2739=EDGE_LOOP('',(#10830,#10831,#10832,#10833,#10834,#10835,#10836,#10837,
#10838,#10839,#10840,#10841));
#2740=EDGE_LOOP('',(#10842,#10843,#10844));
#2741=EDGE_LOOP('',(#10845,#10846,#10847));
#2742=EDGE_LOOP('',(#10848,#10849,#10850,#10851));
#2743=EDGE_LOOP('',(#10852,#10853,#10854,#10855,#10856));
#2744=EDGE_LOOP('',(#10857,#10858,#10859,#10860,#10861));
#2745=EDGE_LOOP('',(#10862,#10863,#10864));
#2746=EDGE_LOOP('',(#10865,#10866,#10867,#10868,#10869,#10870,#10871,#10872,
#10873,#10874,#10875,#10876));
#2747=EDGE_LOOP('',(#10877));
#2748=EDGE_LOOP('',(#10878));
#2749=EDGE_LOOP('',(#10879));
#2750=EDGE_LOOP('',(#10880));
#2751=EDGE_LOOP('',(#10881));
#2752=EDGE_LOOP('',(#10882,#10883,#10884,#10885,#10886));
#2753=EDGE_LOOP('',(#10887,#10888,#10889,#10890,#10891));
#2754=EDGE_LOOP('',(#10892,#10893,#10894,#10895));
#2755=EDGE_LOOP('',(#10896,#10897,#10898,#10899));
#2756=EDGE_LOOP('',(#10900,#10901,#10902,#10903));
#2757=EDGE_LOOP('',(#10904,#10905,#10906,#10907,#10908));
#2758=EDGE_LOOP('',(#10909,#10910,#10911,#10912));
#2759=EDGE_LOOP('',(#10913));
#2760=EDGE_LOOP('',(#10914));
#2761=EDGE_LOOP('',(#10915));
#2762=EDGE_LOOP('',(#10916,#10917));
#2763=EDGE_LOOP('',(#10918,#10919,#10920,#10921));
#2764=EDGE_LOOP('',(#10922,#10923,#10924,#10925));
#2765=EDGE_LOOP('',(#10926));
#2766=EDGE_LOOP('',(#10927,#10928,#10929,#10930));
#2767=EDGE_LOOP('',(#10931,#10932,#10933,#10934,#10935,#10936));
#2768=EDGE_LOOP('',(#10937,#10938,#10939,#10940));
#2769=EDGE_LOOP('',(#10941,#10942,#10943,#10944));
#2770=EDGE_LOOP('',(#10945));
#2771=EDGE_LOOP('',(#10946,#10947,#10948,#10949));
#2772=EDGE_LOOP('',(#10950,#10951,#10952,#10953));
#2773=EDGE_LOOP('',(#10954));
#2774=EDGE_LOOP('',(#10955,#10956,#10957,#10958));
#2775=EDGE_LOOP('',(#10959,#10960,#10961,#10962));
#2776=EDGE_LOOP('',(#10963,#10964,#10965,#10966));
#2777=EDGE_LOOP('',(#10967,#10968,#10969,#10970,#10971,#10972,#10973,#10974));
#2778=EDGE_LOOP('',(#10975,#10976,#10977,#10978));
#2779=EDGE_LOOP('',(#10979,#10980,#10981,#10982));
#2780=EDGE_LOOP('',(#10983,#10984,#10985,#10986));
#2781=EDGE_LOOP('',(#10987,#10988,#10989,#10990));
#2782=EDGE_LOOP('',(#10991,#10992,#10993));
#2783=EDGE_LOOP('',(#10994,#10995,#10996));
#2784=EDGE_LOOP('',(#10997,#10998,#10999,#11000));
#2785=EDGE_LOOP('',(#11001,#11002,#11003,#11004,#11005));
#2786=EDGE_LOOP('',(#11006,#11007,#11008,#11009,#11010,#11011,#11012,#11013));
#2787=EDGE_LOOP('',(#11014,#11015,#11016,#11017));
#2788=EDGE_LOOP('',(#11018,#11019,#11020,#11021,#11022,#11023));
#2789=EDGE_LOOP('',(#11024,#11025,#11026,#11027,#11028));
#2790=EDGE_LOOP('',(#11029,#11030,#11031,#11032,#11033));
#2791=EDGE_LOOP('',(#11034,#11035,#11036,#11037));
#2792=EDGE_LOOP('',(#11038,#11039,#11040));
#2793=EDGE_LOOP('',(#11041,#11042,#11043,#11044,#11045,#11046,#11047,#11048));
#2794=EDGE_LOOP('',(#11049,#11050,#11051,#11052,#11053));
#2795=EDGE_LOOP('',(#11054,#11055,#11056,#11057,#11058,#11059,#11060,#11061,
#11062,#11063,#11064));
#2796=EDGE_LOOP('',(#11065,#11066,#11067,#11068));
#2797=EDGE_LOOP('',(#11069,#11070,#11071));
#2798=EDGE_LOOP('',(#11072,#11073,#11074));
#2799=EDGE_LOOP('',(#11075,#11076,#11077));
#2800=EDGE_LOOP('',(#11078,#11079,#11080,#11081));
#2801=EDGE_LOOP('',(#11082,#11083,#11084,#11085));
#2802=EDGE_LOOP('',(#11086,#11087,#11088,#11089));
#2803=EDGE_LOOP('',(#11090,#11091,#11092,#11093,#11094));
#2804=EDGE_LOOP('',(#11095,#11096,#11097,#11098));
#2805=EDGE_LOOP('',(#11099,#11100,#11101,#11102,#11103));
#2806=EDGE_LOOP('',(#11104,#11105,#11106,#11107));
#2807=EDGE_LOOP('',(#11108,#11109,#11110,#11111,#11112));
#2808=EDGE_LOOP('',(#11113,#11114,#11115,#11116));
#2809=EDGE_LOOP('',(#11117,#11118,#11119));
#2810=EDGE_LOOP('',(#11120,#11121,#11122,#11123));
#2811=EDGE_LOOP('',(#11124,#11125,#11126,#11127,#11128));
#2812=EDGE_LOOP('',(#11129,#11130,#11131,#11132));
#2813=EDGE_LOOP('',(#11133,#11134,#11135,#11136));
#2814=EDGE_LOOP('',(#11137,#11138,#11139,#11140));
#2815=EDGE_LOOP('',(#11141,#11142,#11143,#11144));
#2816=EDGE_LOOP('',(#11145,#11146,#11147,#11148));
#2817=EDGE_LOOP('',(#11149,#11150,#11151,#11152));
#2818=EDGE_LOOP('',(#11153));
#2819=EDGE_LOOP('',(#11154,#11155,#11156,#11157));
#2820=EDGE_LOOP('',(#11158));
#2821=EDGE_LOOP('',(#11159));
#2822=EDGE_LOOP('',(#11160));
#2823=EDGE_LOOP('',(#11161));
#2824=EDGE_LOOP('',(#11162));
#2825=EDGE_LOOP('',(#11163));
#2826=EDGE_LOOP('',(#11164));
#2827=EDGE_LOOP('',(#11165));
#2828=EDGE_LOOP('',(#11166));
#2829=EDGE_LOOP('',(#11167));
#2830=EDGE_LOOP('',(#11168,#11169,#11170,#11171));
#2831=EDGE_LOOP('',(#11172));
#2832=EDGE_LOOP('',(#11173));
#2833=EDGE_LOOP('',(#11174,#11175,#11176,#11177));
#2834=EDGE_LOOP('',(#11178));
#2835=EDGE_LOOP('',(#11179,#11180,#11181,#11182));
#3636=LINE('',#22631,#4705);
#3637=LINE('',#22640,#4706);
#3638=LINE('',#22646,#4707);
#3639=LINE('',#22653,#4708);
#3640=LINE('',#22657,#4709);
#3641=LINE('',#22661,#4710);
#3642=LINE('',#22664,#4711);
#3643=LINE('',#22667,#4712);
#3644=LINE('',#22739,#4713);
#3645=LINE('',#22744,#4714);
#3646=LINE('',#22795,#4715);
#3647=LINE('',#22810,#4716);
#3648=LINE('',#22850,#4717);
#3649=LINE('',#22854,#4718);
#3650=LINE('',#22914,#4719);
#3651=LINE('',#22925,#4720);
#3652=LINE('',#22984,#4721);
#3653=LINE('',#22985,#4722);
#3654=LINE('',#23005,#4723);
#3655=LINE('',#23009,#4724);
#3656=LINE('',#23013,#4725);
#3657=LINE('',#23017,#4726);
#3658=LINE('',#23020,#4727);
#3659=LINE('',#23071,#4728);
#3660=LINE('',#23086,#4729);
#3661=LINE('',#23131,#4730);
#3662=LINE('',#23135,#4731);
#3663=LINE('',#23195,#4732);
#3664=LINE('',#23206,#4733);
#3665=LINE('',#23265,#4734);
#3666=LINE('',#23266,#4735);
#3667=LINE('',#23271,#4736);
#3668=LINE('',#23275,#4737);
#3669=LINE('',#23279,#4738);
#3670=LINE('',#23283,#4739);
#3671=LINE('',#23327,#4740);
#3672=LINE('',#23340,#4741);
#3673=LINE('',#23377,#4742);
#3674=LINE('',#23382,#4743);
#3675=LINE('',#23432,#4744);
#3676=LINE('',#23434,#4745);
#3677=LINE('',#23483,#4746);
#3678=LINE('',#23487,#4747);
#3679=LINE('',#23490,#4748);
#3680=LINE('',#23517,#4749);
#3681=LINE('',#23526,#4750);
#3682=LINE('',#23560,#4751);
#3683=LINE('',#23564,#4752);
#3684=LINE('',#23644,#4753);
#3685=LINE('',#23660,#4754);
#3686=LINE('',#23729,#4755);
#3687=LINE('',#23730,#4756);
#3688=LINE('',#23735,#4757);
#3689=LINE('',#23739,#4758);
#3690=LINE('',#23832,#4759);
#3691=LINE('',#23896,#4760);
#3692=LINE('',#23960,#4761);
#3693=LINE('',#23980,#4762);
#3694=LINE('',#24124,#4763);
#3695=LINE('',#24140,#4764);
#3696=LINE('',#24218,#4765);
#3697=LINE('',#24226,#4766);
#3698=LINE('',#24228,#4767);
#3699=LINE('',#24230,#4768);
#3700=LINE('',#24238,#4769);
#3701=LINE('',#24240,#4770);
#3702=LINE('',#24241,#4771);
#3703=LINE('',#24246,#4772);
#3704=LINE('',#24251,#4773);
#3705=LINE('',#24253,#4774);
#3706=LINE('',#24255,#4775);
#3707=LINE('',#24256,#4776);
#3708=LINE('',#24267,#4777);
#3709=LINE('',#24271,#4778);
#3710=LINE('',#24275,#4779);
#3711=LINE('',#24279,#4780);
#3712=LINE('',#24283,#4781);
#3713=LINE('',#24287,#4782);
#3714=LINE('',#24291,#4783);
#3715=LINE('',#24295,#4784);
#3716=LINE('',#24299,#4785);
#3717=LINE('',#24470,#4786);
#3718=LINE('',#24476,#4787);
#3719=LINE('',#24492,#4788);
#3720=LINE('',#24501,#4789);
#3721=LINE('',#24519,#4790);
#3722=LINE('',#24520,#4791);
#3723=LINE('',#24524,#4792);
#3724=LINE('',#24530,#4793);
#3725=LINE('',#24549,#4794);
#3726=LINE('',#24551,#4795);
#3727=LINE('',#24552,#4796);
#3728=LINE('',#24580,#4797);
#3729=LINE('',#24581,#4798);
#3730=LINE('',#24584,#4799);
#3731=LINE('',#24586,#4800);
#3732=LINE('',#24608,#4801);
#3733=LINE('',#24609,#4802);
#3734=LINE('',#24611,#4803);
#3735=LINE('',#24613,#4804);
#3736=LINE('',#24619,#4805);
#3737=LINE('',#24624,#4806);
#3738=LINE('',#24644,#4807);
#3739=LINE('',#24653,#4808);
#3740=LINE('',#25148,#4809);
#3741=LINE('',#25152,#4810);
#3742=LINE('',#25154,#4811);
#3743=LINE('',#25245,#4812);
#3744=LINE('',#25251,#4813);
#3745=LINE('',#25253,#4814);
#3746=LINE('',#25255,#4815);
#3747=LINE('',#25258,#4816);
#3748=LINE('',#25260,#4817);
#3749=LINE('',#25270,#4818);
#3750=LINE('',#25288,#4819);
#3751=LINE('',#25289,#4820);
#3752=LINE('',#25293,#4821);
#3753=LINE('',#25294,#4822);
#3754=LINE('',#25296,#4823);
#3755=LINE('',#25298,#4824);
#3756=LINE('',#25311,#4825);
#3757=LINE('',#25313,#4826);
#3758=LINE('',#25334,#4827);
#3759=LINE('',#25337,#4828);
#3760=LINE('',#25341,#4829);
#3761=LINE('',#25366,#4830);
#3762=LINE('',#25369,#4831);
#3763=LINE('',#25376,#4832);
#3764=LINE('',#25378,#4833);
#3765=LINE('',#25382,#4834);
#3766=LINE('',#25384,#4835);
#3767=LINE('',#25386,#4836);
#3768=LINE('',#25402,#4837);
#3769=LINE('',#25408,#4838);
#4705=VECTOR('',#17369,13.25);
#4706=VECTOR('',#17380,13.);
#4707=VECTOR('',#17387,19.25);
#4708=VECTOR('',#17394,10.);
#4709=VECTOR('',#17397,10.);
#4710=VECTOR('',#17400,10.);
#4711=VECTOR('',#17403,10.);
#4712=VECTOR('',#17406,19.);
#4713=VECTOR('',#17411,10.);
#4714=VECTOR('',#17416,10.);
#4715=VECTOR('',#17417,10.);
#4716=VECTOR('',#17418,10.);
#4717=VECTOR('',#17421,10.);
#4718=VECTOR('',#17424,10.);
#4719=VECTOR('',#17427,10.);
#4720=VECTOR('',#17428,10.);
#4721=VECTOR('',#17431,10.);
#4722=VECTOR('',#17432,10.);
#4723=VECTOR('',#17435,10.);
#4724=VECTOR('',#17438,10.);
#4725=VECTOR('',#17443,6.05);
#4726=VECTOR('',#17448,10.);
#4727=VECTOR('',#17451,10.);
#4728=VECTOR('',#17452,10.);
#4729=VECTOR('',#17453,10.);
#4730=VECTOR('',#17456,10.);
#4731=VECTOR('',#17459,10.);
#4732=VECTOR('',#17462,10.);
#4733=VECTOR('',#17463,10.);
#4734=VECTOR('',#17466,10.);
#4735=VECTOR('',#17467,10.);
#4736=VECTOR('',#17472,10.);
#4737=VECTOR('',#17477,6.05);
#4738=VECTOR('',#17482,10.);
#4739=VECTOR('',#17485,10.);
#4740=VECTOR('',#17488,10.);
#4741=VECTOR('',#17489,10.);
#4742=VECTOR('',#17492,10.);
#4743=VECTOR('',#17497,10.);
#4744=VECTOR('',#17498,10.);
#4745=VECTOR('',#17499,10.);
#4746=VECTOR('',#17502,6.05);
#4747=VECTOR('',#17507,10.);
#4748=VECTOR('',#17510,10.);
#4749=VECTOR('',#17511,10.);
#4750=VECTOR('',#17512,10.);
#4751=VECTOR('',#17515,10.);
#4752=VECTOR('',#17518,10.);
#4753=VECTOR('',#17521,10.);
#4754=VECTOR('',#17522,10.);
#4755=VECTOR('',#17525,10.);
#4756=VECTOR('',#17526,10.);
#4757=VECTOR('',#17531,10.);
#4758=VECTOR('',#17536,6.05);
#4759=VECTOR('',#17539,10.);
#4760=VECTOR('',#17544,10.);
#4761=VECTOR('',#17549,10.);
#4762=VECTOR('',#17552,2.);
#4763=VECTOR('',#17553,10.);
#4764=VECTOR('',#17556,10.);
#4765=VECTOR('',#17575,10.);
#4766=VECTOR('',#17582,10.);
#4767=VECTOR('',#17583,10.);
#4768=VECTOR('',#17584,10.);
#4769=VECTOR('',#17591,10.);
#4770=VECTOR('',#17594,10.);
#4771=VECTOR('',#17595,10.);
#4772=VECTOR('',#17600,5.30000000000001);
#4773=VECTOR('',#17605,10.);
#4774=VECTOR('',#17606,10.);
#4775=VECTOR('',#17607,10.);
#4776=VECTOR('',#17608,10.);
#4777=VECTOR('',#17619,5.05000000000001);
#4778=VECTOR('',#17624,5.29999999999999);
#4779=VECTOR('',#17629,5.04999999999999);
#4780=VECTOR('',#17634,5.29999999999999);
#4781=VECTOR('',#17639,5.04999999999999);
#4782=VECTOR('',#17644,5.30000000000001);
#4783=VECTOR('',#17649,5.05000000000001);
#4784=VECTOR('',#17654,9.75);
#4785=VECTOR('',#17659,9.49999999999999);
#4786=VECTOR('',#17668,6.);
#4787=VECTOR('',#17673,10.);
#4788=VECTOR('',#17674,10.);
#4789=VECTOR('',#17687,10.);
#4790=VECTOR('',#17690,10.);
#4791=VECTOR('',#17691,10.);
#4792=VECTOR('',#17696,10.);
#4793=VECTOR('',#17705,10.);
#4794=VECTOR('',#17712,10.);
#4795=VECTOR('',#17713,10.);
#4796=VECTOR('',#17714,10.);
#4797=VECTOR('',#17735,10.);
#4798=VECTOR('',#17736,10.);
#4799=VECTOR('',#17739,10.);
#4800=VECTOR('',#17742,10.);
#4801=VECTOR('',#17753,10.);
#4802=VECTOR('',#17754,10.);
#4803=VECTOR('',#17757,10.);
#4804=VECTOR('',#17760,10.);
#4805=VECTOR('',#17767,10.);
#4806=VECTOR('',#17772,10.);
#4807=VECTOR('',#17795,43.05);
#4808=VECTOR('',#17808,10.);
#4809=VECTOR('',#17843,10.);
#4810=VECTOR('',#17846,10.);
#4811=VECTOR('',#17849,10.);
#4812=VECTOR('',#17888,10.);
#4813=VECTOR('',#17897,10.);
#4814=VECTOR('',#17900,10.);
#4815=VECTOR('',#17901,10.);
#4816=VECTOR('',#17904,10.);
#4817=VECTOR('',#17907,10.);
#4818=VECTOR('',#17920,10.);
#4819=VECTOR('',#17947,10.);
#4820=VECTOR('',#17948,10.);
#4821=VECTOR('',#17953,10.);
#4822=VECTOR('',#17954,10.);
#4823=VECTOR('',#17957,10.);
#4824=VECTOR('',#17960,10.);
#4825=VECTOR('',#17963,10.);
#4826=VECTOR('',#17966,10.);
#4827=VECTOR('',#17979,10.);
#4828=VECTOR('',#17982,2.);
#4829=VECTOR('',#17987,10.);
#4830=VECTOR('',#18032,10.);
#4831=VECTOR('',#18037,10.);
#4832=VECTOR('',#18050,10.);
#4833=VECTOR('',#18053,6.5);
#4834=VECTOR('',#18058,6.5);
#4835=VECTOR('',#18061,6.5);
#4836=VECTOR('',#18064,6.5);
#4837=VECTOR('',#18093,16.6);
#4838=VECTOR('',#18102,16.505);
#5790=CIRCLE('',#15496,13.5);
#5791=CIRCLE('',#15497,13.);
#5792=CIRCLE('',#15498,13.);
#5793=CIRCLE('',#15500,16.505);
#5794=CIRCLE('',#15502,13.);
#5795=CIRCLE('',#15504,19.5);
#5796=CIRCLE('',#15505,19.);
#5797=CIRCLE('',#15507,6.54999999999999);
#5798=CIRCLE('',#15508,6.55);
#5799=CIRCLE('',#15509,6.55);
#5800=CIRCLE('',#15510,6.54999999999999);
#5801=CIRCLE('',#15512,19.);
#5802=CIRCLE('',#15514,6.05);
#5803=CIRCLE('',#15515,6.05);
#5804=CIRCLE('',#15517,6.05);
#5805=CIRCLE('',#15518,6.54999999999999);
#5806=CIRCLE('',#15521,2.00000000000001);
#5807=CIRCLE('',#15522,2.00000000000001);
#5808=CIRCLE('',#15524,6.05);
#5809=CIRCLE('',#15526,6.05);
#5810=CIRCLE('',#15528,6.05);
#5811=CIRCLE('',#15529,6.55);
#5812=CIRCLE('',#15532,2.);
#5813=CIRCLE('',#15533,2.00000000000001);
#5814=CIRCLE('',#15535,6.05);
#5815=CIRCLE('',#15537,6.05);
#5816=CIRCLE('',#15538,6.54999999999999);
#5817=CIRCLE('',#15540,6.05);
#5818=CIRCLE('',#15541,6.05);
#5819=CIRCLE('',#15543,6.05);
#5820=CIRCLE('',#15545,6.05);
#5821=CIRCLE('',#15547,6.05);
#5822=CIRCLE('',#15548,6.55);
#5823=CIRCLE('',#15551,2.);
#5824=CIRCLE('',#15552,1.99999999999999);
#5825=CIRCLE('',#15554,6.05);
#5826=CIRCLE('',#15556,2.);
#5827=CIRCLE('',#15557,1.5);
#5828=CIRCLE('',#15559,2.);
#5829=CIRCLE('',#15561,2.);
#5830=CIRCLE('',#15562,1.5);
#5831=CIRCLE('',#15564,12.);
#5832=CIRCLE('',#15565,1.99999999999999);
#5833=CIRCLE('',#15566,10.);
#5834=CIRCLE('',#15568,12.);
#5835=CIRCLE('',#15569,26.);
#5836=CIRCLE('',#15570,26.);
#5837=CIRCLE('',#15571,12.);
#5838=CIRCLE('',#15572,26.);
#5839=CIRCLE('',#15573,26.);
#5840=CIRCLE('',#15574,12.);
#5841=CIRCLE('',#15575,26.);
#5842=CIRCLE('',#15576,26.);
#5843=CIRCLE('',#15578,5.55000000000001);
#5844=CIRCLE('',#15579,5.05000000000001);
#5845=CIRCLE('',#15581,5.55);
#5846=CIRCLE('',#15582,5.55000000000001);
#5847=CIRCLE('',#15583,10.);
#5848=CIRCLE('',#15584,5.55);
#5849=CIRCLE('',#15586,5.05000000000001);
#5850=CIRCLE('',#15588,5.04999999999999);
#5851=CIRCLE('',#15590,5.04999999999999);
#5852=CIRCLE('',#15592,5.04999999999999);
#5853=CIRCLE('',#15594,5.04999999999999);
#5854=CIRCLE('',#15596,5.05000000000001);
#5855=CIRCLE('',#15598,5.05000000000001);
#5856=CIRCLE('',#15600,9.49999999999999);
#5857=CIRCLE('',#15602,9.49999999999999);
#5858=CIRCLE('',#15603,2.00000000000001);
#5859=CIRCLE('',#15605,6.);
#5860=CIRCLE('',#15607,2.00000000000001);
#5861=CIRCLE('',#15609,2.);
#5862=CIRCLE('',#15610,1.99999999999999);
#5863=CIRCLE('',#15611,2.);
#5864=CIRCLE('',#15613,2.);
#5865=CIRCLE('',#15616,2.);
#5866=CIRCLE('',#15618,2.);
#5867=CIRCLE('',#15620,1.99999999999999);
#5868=CIRCLE('',#15622,2.);
#5869=CIRCLE('',#15625,2.);
#5870=CIRCLE('',#15627,2.);
#5871=CIRCLE('',#15629,1.99999999999999);
#5872=CIRCLE('',#15631,2.);
#5873=CIRCLE('',#15632,1.99999999999999);
#5874=CIRCLE('',#15635,2.);
#5875=CIRCLE('',#15637,2.00000000000001);
#5876=CIRCLE('',#15639,2.00000000000001);
#5877=CIRCLE('',#15645,26.);
#5878=CIRCLE('',#15646,26.);
#5879=CIRCLE('',#15647,26.);
#5880=CIRCLE('',#15648,26.);
#5881=CIRCLE('',#15649,45.05);
#5882=CIRCLE('',#15650,6.5);
#5883=CIRCLE('',#15651,6.5);
#5884=CIRCLE('',#15652,6.5);
#5885=CIRCLE('',#15653,6.5);
#5886=CIRCLE('',#15655,2.);
#5887=CIRCLE('',#15656,43.05);
#5888=CIRCLE('',#15657,43.05);
#5889=CIRCLE('',#15659,43.05);
#5890=CIRCLE('',#15661,1.99999999999999);
#5891=CIRCLE('',#15662,28.);
#5892=CIRCLE('',#15664,1.99999999999999);
#5893=CIRCLE('',#15666,28.);
#5894=CIRCLE('',#15667,1.99999999999999);
#5895=CIRCLE('',#15668,1.99999999999999);
#5896=CIRCLE('',#15670,16.6);
#5897=CIRCLE('',#15672,28.);
#5898=CIRCLE('',#15673,26.);
#5899=CIRCLE('',#15675,2.);
#5900=CIRCLE('',#15676,10.);
#5901=CIRCLE('',#15677,6.5);
#5902=CIRCLE('',#15679,26.);
#5903=CIRCLE('',#15680,28.);
#5904=CIRCLE('',#15682,28.);
#5905=CIRCLE('',#15683,28.);
#5906=CIRCLE('',#15685,26.);
#5907=CIRCLE('',#15686,28.);
#5908=CIRCLE('',#15688,2.);
#5909=CIRCLE('',#15689,10.);
#5910=CIRCLE('',#15690,2.);
#5911=CIRCLE('',#15691,6.5);
#5912=CIRCLE('',#15693,26.);
#5913=CIRCLE('',#15694,28.);
#5914=CIRCLE('',#15696,2.);
#5915=CIRCLE('',#15697,10.);
#5916=CIRCLE('',#15698,2.);
#5917=CIRCLE('',#15699,6.5);
#5918=CIRCLE('',#15701,2.);
#5919=CIRCLE('',#15702,1.99999999999999);
#5920=CIRCLE('',#15705,28.);
#5921=CIRCLE('',#15707,28.);
#5922=CIRCLE('',#15708,28.);
#5923=CIRCLE('',#15711,2.);
#5924=CIRCLE('',#15712,2.00000000000003);
#5925=CIRCLE('',#15713,28.);
#5926=CIRCLE('',#15715,2.);
#5927=CIRCLE('',#15717,2.00000000000001);
#5928=CIRCLE('',#15718,28.);
#5929=CIRCLE('',#15720,2.);
#5930=CIRCLE('',#15721,2.);
#5931=CIRCLE('',#15723,2.);
#5932=CIRCLE('',#15724,2.);
#5933=CIRCLE('',#15726,10.);
#5934=CIRCLE('',#15727,2.00000000000001);
#5935=CIRCLE('',#15730,28.);
#5936=CIRCLE('',#15736,2.);
#5937=CIRCLE('',#15739,10.);
#5938=CIRCLE('',#15742,2.);
#5939=CIRCLE('',#15744,10.);
#5940=CIRCLE('',#15746,2.00000000000001);
#5941=CIRCLE('',#15747,1.99999999999999);
#5942=CIRCLE('',#15748,2.00000000000001);
#5943=CIRCLE('',#15750,2.00000000000001);
#5944=CIRCLE('',#15751,1.99999999999999);
#5945=CIRCLE('',#15752,2.00000000000001);
#5946=CIRCLE('',#15754,2.00000000000001);
#5947=CIRCLE('',#15755,2.00000000000001);
#5948=CIRCLE('',#15757,2.);
#5949=CIRCLE('',#15759,2.);
#5950=CIRCLE('',#15762,2.);
#5951=CIRCLE('',#15764,10.);
#5952=CIRCLE('',#15770,2.00000000000001);
#5953=CIRCLE('',#15771,1.99999999999999);
#5954=CIRCLE('',#15776,6.5);
#5955=CIRCLE('',#15793,16.6);
#5956=CIRCLE('',#15795,16.505);
#6447=VERTEX_POINT('',#22628);
#6448=VERTEX_POINT('',#22630);
#6449=VERTEX_POINT('',#22632);
#6450=VERTEX_POINT('',#22636);
#6451=VERTEX_POINT('',#22639);
#6452=VERTEX_POINT('',#22643);
#6453=VERTEX_POINT('',#22645);
#6454=VERTEX_POINT('',#22649);
#6455=VERTEX_POINT('',#22650);
#6456=VERTEX_POINT('',#22652);
#6457=VERTEX_POINT('',#22654);
#6458=VERTEX_POINT('',#22656);
#6459=VERTEX_POINT('',#22658);
#6460=VERTEX_POINT('',#22660);
#6461=VERTEX_POINT('',#22662);
#6462=VERTEX_POINT('',#22666);
#6463=VERTEX_POINT('',#22668);
#6464=VERTEX_POINT('',#22704);
#6465=VERTEX_POINT('',#22738);
#6466=VERTEX_POINT('',#22740);
#6467=VERTEX_POINT('',#22742);
#6468=VERTEX_POINT('',#22793);
#6469=VERTEX_POINT('',#22794);
#6470=VERTEX_POINT('',#22796);
#6471=VERTEX_POINT('',#22809);
#6472=VERTEX_POINT('',#22848);
#6473=VERTEX_POINT('',#22849);
#6474=VERTEX_POINT('',#22851);
#6475=VERTEX_POINT('',#22853);
#6476=VERTEX_POINT('',#22912);
#6477=VERTEX_POINT('',#22913);
#6478=VERTEX_POINT('',#22915);
#6479=VERTEX_POINT('',#22924);
#6480=VERTEX_POINT('',#22983);
#6481=VERTEX_POINT('',#22987);
#6482=VERTEX_POINT('',#22992);
#6483=VERTEX_POINT('',#22999);
#6484=VERTEX_POINT('',#23004);
#6485=VERTEX_POINT('',#23006);
#6486=VERTEX_POINT('',#23008);
#6487=VERTEX_POINT('',#23012);
#6488=VERTEX_POINT('',#23016);
#6489=VERTEX_POINT('',#23018);
#6490=VERTEX_POINT('',#23069);
#6491=VERTEX_POINT('',#23070);
#6492=VERTEX_POINT('',#23072);
#6493=VERTEX_POINT('',#23085);
#6494=VERTEX_POINT('',#23087);
#6495=VERTEX_POINT('',#23129);
#6496=VERTEX_POINT('',#23130);
#6497=VERTEX_POINT('',#23132);
#6498=VERTEX_POINT('',#23134);
#6499=VERTEX_POINT('',#23193);
#6500=VERTEX_POINT('',#23194);
#6501=VERTEX_POINT('',#23196);
#6502=VERTEX_POINT('',#23205);
#6503=VERTEX_POINT('',#23264);
#6504=VERTEX_POINT('',#23268);
#6505=VERTEX_POINT('',#23270);
#6506=VERTEX_POINT('',#23274);
#6507=VERTEX_POINT('',#23278);
#6508=VERTEX_POINT('',#23280);
#6509=VERTEX_POINT('',#23282);
#6510=VERTEX_POINT('',#23325);
#6511=VERTEX_POINT('',#23326);
#6512=VERTEX_POINT('',#23328);
#6513=VERTEX_POINT('',#23339);
#6514=VERTEX_POINT('',#23376);
#6515=VERTEX_POINT('',#23378);
#6516=VERTEX_POINT('',#23380);
#6517=VERTEX_POINT('',#23431);
#6518=VERTEX_POINT('',#23433);
#6519=VERTEX_POINT('',#23482);
#6520=VERTEX_POINT('',#23486);
#6521=VERTEX_POINT('',#23488);
#6522=VERTEX_POINT('',#23515);
#6523=VERTEX_POINT('',#23516);
#6524=VERTEX_POINT('',#23518);
#6525=VERTEX_POINT('',#23525);
#6526=VERTEX_POINT('',#23558);
#6527=VERTEX_POINT('',#23559);
#6528=VERTEX_POINT('',#23561);
#6529=VERTEX_POINT('',#23563);
#6530=VERTEX_POINT('',#23642);
#6531=VERTEX_POINT('',#23643);
#6532=VERTEX_POINT('',#23645);
#6533=VERTEX_POINT('',#23659);
#6534=VERTEX_POINT('',#23661);
#6535=VERTEX_POINT('',#23728);
#6536=VERTEX_POINT('',#23732);
#6537=VERTEX_POINT('',#23734);
#6538=VERTEX_POINT('',#23738);
#6539=VERTEX_POINT('',#23757);
#6540=VERTEX_POINT('',#23758);
#6541=VERTEX_POINT('',#23763);
#6542=VERTEX_POINT('',#23768);
#6543=VERTEX_POINT('',#23817);
#6544=VERTEX_POINT('',#23831);
#6545=VERTEX_POINT('',#23859);
#6546=VERTEX_POINT('',#23864);
#6547=VERTEX_POINT('',#23869);
#6548=VERTEX_POINT('',#23879);
#6549=VERTEX_POINT('',#23880);
#6550=VERTEX_POINT('',#23893);
#6551=VERTEX_POINT('',#23895);
#6552=VERTEX_POINT('',#23938);
#6553=VERTEX_POINT('',#23948);
#6554=VERTEX_POINT('',#23959);
#6555=VERTEX_POINT('',#23961);
#6556=VERTEX_POINT('',#23978);
#6557=VERTEX_POINT('',#24001);
#6558=VERTEX_POINT('',#24002);
#6559=VERTEX_POINT('',#24007);
#6560=VERTEX_POINT('',#24013);
#6561=VERTEX_POINT('',#24018);
#6562=VERTEX_POINT('',#24044);
#6563=VERTEX_POINT('',#24051);
#6564=VERTEX_POINT('',#24110);
#6565=VERTEX_POINT('',#24123);
#6566=VERTEX_POINT('',#24138);
#6567=VERTEX_POINT('',#24139);
#6568=VERTEX_POINT('',#24141);
#6569=VERTEX_POINT('',#24143);
#6570=VERTEX_POINT('',#24197);
#6571=VERTEX_POINT('',#24207);
#6572=VERTEX_POINT('',#24209);
#6573=VERTEX_POINT('',#24213);
#6574=VERTEX_POINT('',#24215);
#6575=VERTEX_POINT('',#24217);
#6576=VERTEX_POINT('',#24219);
#6577=VERTEX_POINT('',#24221);
#6578=VERTEX_POINT('',#24223);
#6579=VERTEX_POINT('',#24225);
#6580=VERTEX_POINT('',#24227);
#6581=VERTEX_POINT('',#24229);
#6582=VERTEX_POINT('',#24231);
#6583=VERTEX_POINT('',#24233);
#6584=VERTEX_POINT('',#24235);
#6585=VERTEX_POINT('',#24237);
#6586=VERTEX_POINT('',#24243);
#6587=VERTEX_POINT('',#24245);
#6588=VERTEX_POINT('',#24249);
#6589=VERTEX_POINT('',#24250);
#6590=VERTEX_POINT('',#24252);
#6591=VERTEX_POINT('',#24254);
#6592=VERTEX_POINT('',#24257);
#6593=VERTEX_POINT('',#24259);
#6594=VERTEX_POINT('',#24261);
#6595=VERTEX_POINT('',#24263);
#6596=VERTEX_POINT('',#24266);
#6597=VERTEX_POINT('',#24270);
#6598=VERTEX_POINT('',#24274);
#6599=VERTEX_POINT('',#24278);
#6600=VERTEX_POINT('',#24282);
#6601=VERTEX_POINT('',#24286);
#6602=VERTEX_POINT('',#24290);
#6603=VERTEX_POINT('',#24294);
#6604=VERTEX_POINT('',#24298);
#6605=VERTEX_POINT('',#24300);
#6606=VERTEX_POINT('',#24316);
#6607=VERTEX_POINT('',#24443);
#6608=VERTEX_POINT('',#24468);
#6609=VERTEX_POINT('',#24472);
#6610=VERTEX_POINT('',#24473);
#6611=VERTEX_POINT('',#24475);
#6612=VERTEX_POINT('',#24477);
#6613=VERTEX_POINT('',#24494);
#6614=VERTEX_POINT('',#24496);
#6615=VERTEX_POINT('',#24503);
#6616=VERTEX_POINT('',#24504);
#6617=VERTEX_POINT('',#24522);
#6618=VERTEX_POINT('',#24529);
#6619=VERTEX_POINT('',#24548);
#6620=VERTEX_POINT('',#24550);
#6621=VERTEX_POINT('',#24560);
#6622=VERTEX_POINT('',#24564);
#6623=VERTEX_POINT('',#24565);
#6624=VERTEX_POINT('',#24583);
#6625=VERTEX_POINT('',#24592);
#6626=VERTEX_POINT('',#24593);
#6627=VERTEX_POINT('',#24616);
#6628=VERTEX_POINT('',#24618);
#6629=VERTEX_POINT('',#24621);
#6630=VERTEX_POINT('',#24623);
#6631=VERTEX_POINT('',#24626);
#6632=VERTEX_POINT('',#24628);
#6633=VERTEX_POINT('',#24630);
#6634=VERTEX_POINT('',#24632);
#6635=VERTEX_POINT('',#24634);
#6636=VERTEX_POINT('',#24637);
#6637=VERTEX_POINT('',#24639);
#6638=VERTEX_POINT('',#24643);
#6639=VERTEX_POINT('',#24647);
#6640=VERTEX_POINT('',#24651);
#6641=VERTEX_POINT('',#24764);
#6642=VERTEX_POINT('',#24766);
#6643=VERTEX_POINT('',#25078);
#6644=VERTEX_POINT('',#25081);
#6645=VERTEX_POINT('',#25083);
#6646=VERTEX_POINT('',#25100);
#6647=VERTEX_POINT('',#25103);
#6648=VERTEX_POINT('',#25106);
#6649=VERTEX_POINT('',#25107);
#6650=VERTEX_POINT('',#25128);
#6651=VERTEX_POINT('',#25130);
#6652=VERTEX_POINT('',#25147);
#6653=VERTEX_POINT('',#25149);
#6654=VERTEX_POINT('',#25151);
#6655=VERTEX_POINT('',#25156);
#6656=VERTEX_POINT('',#25157);
#6657=VERTEX_POINT('',#25172);
#6658=VERTEX_POINT('',#25174);
#6659=VERTEX_POINT('',#25191);
#6660=VERTEX_POINT('',#25193);
#6661=VERTEX_POINT('',#25196);
#6662=VERTEX_POINT('',#25199);
#6663=VERTEX_POINT('',#25200);
#6664=VERTEX_POINT('',#25215);
#6665=VERTEX_POINT('',#25217);
#6666=VERTEX_POINT('',#25234);
#6667=VERTEX_POINT('',#25236);
#6668=VERTEX_POINT('',#25239);
#6669=VERTEX_POINT('',#25242);
#6670=VERTEX_POINT('',#25250);
#6671=VERTEX_POINT('',#25254);
#6672=VERTEX_POINT('',#25256);
#6673=VERTEX_POINT('',#25262);
#6674=VERTEX_POINT('',#25264);
#6675=VERTEX_POINT('',#25268);
#6676=VERTEX_POINT('',#25272);
#6677=VERTEX_POINT('',#25276);
#6678=VERTEX_POINT('',#25280);
#6679=VERTEX_POINT('',#25284);
#6680=VERTEX_POINT('',#25291);
#6681=VERTEX_POINT('',#25300);
#6682=VERTEX_POINT('',#25336);
#6683=VERTEX_POINT('',#25340);
#6684=VERTEX_POINT('',#25344);
#6685=VERTEX_POINT('',#25349);
#6686=VERTEX_POINT('',#25380);
#6687=VERTEX_POINT('',#25401);
#6688=VERTEX_POINT('',#25405);
#7934=EDGE_CURVE('',#6447,#6447,#5790,.T.);
#7935=EDGE_CURVE('',#6447,#6448,#3636,.T.);
#7936=EDGE_CURVE('',#6448,#6449,#5791,.T.);
#7937=EDGE_CURVE('',#6449,#6448,#5792,.T.);
#7938=EDGE_CURVE('',#6450,#6450,#5793,.T.);
#7939=EDGE_CURVE('',#6449,#6451,#3637,.T.);
#7940=EDGE_CURVE('',#6451,#6451,#5794,.T.);
#7941=EDGE_CURVE('',#6452,#6452,#5795,.T.);
#7942=EDGE_CURVE('',#6452,#6453,#3638,.T.);
#7943=EDGE_CURVE('',#6453,#6453,#5796,.T.);
#7944=EDGE_CURVE('',#6454,#6455,#5797,.T.);
#7945=EDGE_CURVE('',#6456,#6454,#3639,.T.);
#7946=EDGE_CURVE('',#6457,#6456,#5798,.T.);
#7947=EDGE_CURVE('',#6458,#6457,#3640,.T.);
#7948=EDGE_CURVE('',#6459,#6458,#5799,.T.);
#7949=EDGE_CURVE('',#6460,#6459,#3641,.T.);
#7950=EDGE_CURVE('',#6461,#6460,#5800,.T.);
#7951=EDGE_CURVE('',#6455,#6461,#3642,.T.);
#7952=EDGE_CURVE('',#6453,#6462,#3643,.T.);
#7953=EDGE_CURVE('',#6463,#6462,#1059,.T.);
#7954=EDGE_CURVE('',#6463,#6463,#5801,.T.);
#7955=EDGE_CURVE('',#6464,#6463,#1060,.T.);
#7956=EDGE_CURVE('',#6462,#6464,#1061,.T.);
#7957=EDGE_CURVE('',#6455,#6465,#3644,.T.);
#7958=EDGE_CURVE('',#6465,#6466,#5802,.T.);
#7959=EDGE_CURVE('',#6466,#6467,#5803,.T.);
#7960=EDGE_CURVE('',#6467,#6454,#3645,.T.);
#7961=EDGE_CURVE('',#6468,#6469,#3646,.T.);
#7962=EDGE_CURVE('',#6469,#6470,#1062,.T.);
#7963=EDGE_CURVE('',#6470,#6471,#3647,.T.);
#7964=EDGE_CURVE('',#6471,#6468,#1063,.T.);
#7965=EDGE_CURVE('',#6470,#6454,#1064,.T.);
#7966=EDGE_CURVE('',#6467,#6471,#1065,.T.);
#7967=EDGE_CURVE('',#6472,#6473,#3648,.T.);
#7968=EDGE_CURVE('',#6473,#6474,#5804,.T.);
#7969=EDGE_CURVE('',#6474,#6475,#3649,.T.);
#7970=EDGE_CURVE('',#6475,#6472,#5805,.T.);
#7971=EDGE_CURVE('',#6472,#6469,#1066,.T.);
#7972=EDGE_CURVE('',#6468,#6473,#1067,.T.);
#7973=EDGE_CURVE('',#6476,#6477,#3650,.T.);
#7974=EDGE_CURVE('',#6477,#6478,#1068,.T.);
#7975=EDGE_CURVE('',#6478,#6479,#3651,.T.);
#7976=EDGE_CURVE('',#6479,#6476,#1069,.T.);
#7977=EDGE_CURVE('',#6478,#6475,#1070,.T.);
#7978=EDGE_CURVE('',#6474,#6479,#1071,.T.);
#7979=EDGE_CURVE('',#6455,#6477,#1072,.T.);
#7980=EDGE_CURVE('',#6476,#6465,#1073,.T.);
#7981=EDGE_CURVE('',#6480,#6475,#3652,.T.);
#7982=EDGE_CURVE('',#6472,#6480,#3653,.T.);
#7983=EDGE_CURVE('',#6481,#6461,#1074,.T.);
#7984=EDGE_CURVE('',#6482,#6481,#1075,.T.);
#7985=EDGE_CURVE('',#6483,#6482,#1076,.T.);
#7986=EDGE_CURVE('',#6483,#6484,#3654,.T.);
#7987=EDGE_CURVE('',#6485,#6484,#5806,.T.);
#7988=EDGE_CURVE('',#6485,#6486,#3655,.T.);
#7989=EDGE_CURVE('',#6480,#6486,#5807,.T.);
#7990=EDGE_CURVE('',#6466,#6487,#3656,.T.);
#7991=EDGE_CURVE('',#6487,#6487,#5808,.T.);
#7992=EDGE_CURVE('',#6456,#6488,#3657,.T.);
#7993=EDGE_CURVE('',#6488,#6489,#5809,.T.);
#7994=EDGE_CURVE('',#6489,#6457,#3658,.T.);
#7995=EDGE_CURVE('',#6490,#6491,#3659,.T.);
#7996=EDGE_CURVE('',#6491,#6492,#1077,.T.);
#7997=EDGE_CURVE('',#6492,#6493,#3660,.T.);
#7998=EDGE_CURVE('',#6493,#6494,#1078,.T.);
#7999=EDGE_CURVE('',#6494,#6490,#1079,.T.);
#8000=EDGE_CURVE('',#6492,#6457,#1080,.T.);
#8001=EDGE_CURVE('',#6489,#6493,#1081,.T.);
#8002=EDGE_CURVE('',#6495,#6496,#3661,.T.);
#8003=EDGE_CURVE('',#6496,#6497,#5810,.T.);
#8004=EDGE_CURVE('',#6497,#6498,#3662,.T.);
#8005=EDGE_CURVE('',#6498,#6495,#5811,.T.);
#8006=EDGE_CURVE('',#6495,#6491,#1082,.T.);
#8007=EDGE_CURVE('',#6490,#6496,#1083,.T.);
#8008=EDGE_CURVE('',#6499,#6500,#3663,.T.);
#8009=EDGE_CURVE('',#6500,#6501,#1084,.T.);
#8010=EDGE_CURVE('',#6501,#6502,#3664,.T.);
#8011=EDGE_CURVE('',#6502,#6499,#1085,.T.);
#8012=EDGE_CURVE('',#6501,#6498,#1086,.T.);
#8013=EDGE_CURVE('',#6497,#6502,#1087,.T.);
#8014=EDGE_CURVE('',#6456,#6500,#1088,.T.);
#8015=EDGE_CURVE('',#6499,#6488,#1089,.T.);
#8016=EDGE_CURVE('',#6503,#6498,#3665,.T.);
#8017=EDGE_CURVE('',#6495,#6503,#3666,.T.);
#8018=EDGE_CURVE('',#6480,#6504,#5812,.T.);
#8019=EDGE_CURVE('',#6504,#6505,#3667,.T.);
#8020=EDGE_CURVE('',#6505,#6503,#5813,.F.);
#8021=EDGE_CURVE('',#6494,#6506,#3668,.T.);
#8022=EDGE_CURVE('',#6506,#6506,#5814,.T.);
#8023=EDGE_CURVE('',#6483,#6507,#3669,.T.);
#8024=EDGE_CURVE('',#6507,#6508,#5815,.T.);
#8025=EDGE_CURVE('',#6508,#6509,#3670,.T.);
#8026=EDGE_CURVE('',#6509,#6483,#5816,.T.);
#8027=EDGE_CURVE('',#6510,#6511,#3671,.T.);
#8028=EDGE_CURVE('',#6511,#6512,#1090,.T.);
#8029=EDGE_CURVE('',#6512,#6513,#3672,.T.);
#8030=EDGE_CURVE('',#6513,#6510,#1091,.T.);
#8031=EDGE_CURVE('',#6512,#6509,#1092,.T.);
#8032=EDGE_CURVE('',#6508,#6513,#1093,.T.);
#8033=EDGE_CURVE('',#6460,#6514,#3673,.T.);
#8034=EDGE_CURVE('',#6514,#6515,#5817,.T.);
#8035=EDGE_CURVE('',#6515,#6516,#5818,.T.);
#8036=EDGE_CURVE('',#6516,#6461,#3674,.T.);
#8037=EDGE_CURVE('',#6460,#6511,#1094,.T.);
#8038=EDGE_CURVE('',#6510,#6514,#1095,.T.);
#8039=EDGE_CURVE('',#6517,#6482,#3675,.T.);
#8040=EDGE_CURVE('',#6481,#6518,#3676,.T.);
#8041=EDGE_CURVE('',#6518,#6517,#1096,.T.);
#8042=EDGE_CURVE('',#6516,#6518,#1097,.T.);
#8043=EDGE_CURVE('',#6517,#6507,#1098,.T.);
#8044=EDGE_CURVE('',#6515,#6519,#3677,.T.);
#8045=EDGE_CURVE('',#6519,#6519,#5819,.T.);
#8046=EDGE_CURVE('',#6458,#6520,#3678,.T.);
#8047=EDGE_CURVE('',#6520,#6521,#5820,.T.);
#8048=EDGE_CURVE('',#6521,#6459,#3679,.T.);
#8049=EDGE_CURVE('',#6522,#6523,#3680,.T.);
#8050=EDGE_CURVE('',#6523,#6524,#1099,.T.);
#8051=EDGE_CURVE('',#6524,#6525,#3681,.T.);
#8052=EDGE_CURVE('',#6525,#6522,#1100,.T.);
#8053=EDGE_CURVE('',#6524,#6459,#1101,.T.);
#8054=EDGE_CURVE('',#6521,#6525,#1102,.T.);
#8055=EDGE_CURVE('',#6526,#6527,#3682,.T.);
#8056=EDGE_CURVE('',#6527,#6528,#5821,.T.);
#8057=EDGE_CURVE('',#6528,#6529,#3683,.T.);
#8058=EDGE_CURVE('',#6529,#6526,#5822,.T.);
#8059=EDGE_CURVE('',#6526,#6523,#1103,.T.);
#8060=EDGE_CURVE('',#6522,#6527,#1104,.T.);
#8061=EDGE_CURVE('',#6530,#6531,#3684,.T.);
#8062=EDGE_CURVE('',#6531,#6532,#1105,.T.);
#8063=EDGE_CURVE('',#6532,#6533,#3685,.T.);
#8064=EDGE_CURVE('',#6533,#6534,#1106,.T.);
#8065=EDGE_CURVE('',#6534,#6530,#1107,.T.);
#8066=EDGE_CURVE('',#6532,#6529,#1108,.T.);
#8067=EDGE_CURVE('',#6528,#6533,#1109,.T.);
#8068=EDGE_CURVE('',#6458,#6531,#1110,.T.);
#8069=EDGE_CURVE('',#6530,#6520,#1111,.T.);
#8070=EDGE_CURVE('',#6535,#6529,#3686,.T.);
#8071=EDGE_CURVE('',#6526,#6535,#3687,.T.);
#8072=EDGE_CURVE('',#6503,#6536,#5823,.F.);
#8073=EDGE_CURVE('',#6536,#6537,#3688,.T.);
#8074=EDGE_CURVE('',#6537,#6535,#5824,.F.);
#8075=EDGE_CURVE('',#6534,#6538,#3689,.T.);
#8076=EDGE_CURVE('',#6538,#6538,#5825,.T.);
#8077=EDGE_CURVE('',#6539,#6540,#1112,.T.);
#8078=EDGE_CURVE('',#6539,#6541,#1113,.T.);
#8079=EDGE_CURVE('',#6541,#6542,#1114,.T.);
#8080=EDGE_CURVE('',#6542,#6540,#1115,.T.);
#8081=EDGE_CURVE('',#6541,#6543,#1116,.T.);
#8082=EDGE_CURVE('',#6543,#6544,#3690,.T.);
#8083=EDGE_CURVE('',#6544,#6542,#1117,.T.);
#8084=EDGE_CURVE('',#6540,#6545,#1118,.T.);
#8085=EDGE_CURVE('',#6545,#6546,#1119,.T.);
#8086=EDGE_CURVE('',#6546,#6547,#1120,.T.);
#8087=EDGE_CURVE('',#6547,#6539,#1121,.T.);
#8088=EDGE_CURVE('',#6548,#6549,#1122,.F.);
#8089=EDGE_CURVE('',#6549,#6550,#5826,.T.);
#8090=EDGE_CURVE('',#6550,#6551,#3691,.T.);
#8091=EDGE_CURVE('',#6551,#6548,#5827,.T.);
#8092=EDGE_CURVE('',#6550,#6544,#1123,.T.);
#8093=EDGE_CURVE('',#6543,#6551,#1124,.T.);
#8094=EDGE_CURVE('',#6545,#6552,#1125,.T.);
#8095=EDGE_CURVE('',#6552,#6547,#1126,.T.);
#8096=EDGE_CURVE('',#6553,#6549,#1127,.F.);
#8097=EDGE_CURVE('',#6553,#6554,#3692,.T.);
#8098=EDGE_CURVE('',#6554,#6555,#1128,.T.);
#8099=EDGE_CURVE('',#6555,#6556,#5828,.F.);
#8100=EDGE_CURVE('',#6556,#6552,#3693,.T.);
#8101=EDGE_CURVE('',#6557,#6558,#1129,.T.);
#8102=EDGE_CURVE('',#6557,#6559,#1130,.T.);
#8103=EDGE_CURVE('',#6559,#6560,#1131,.T.);
#8104=EDGE_CURVE('',#6560,#6561,#1132,.T.);
#8105=EDGE_CURVE('',#6561,#6558,#1133,.T.);
#8106=EDGE_CURVE('',#6558,#6562,#336,.T.);
#8107=EDGE_CURVE('',#6563,#6562,#1134,.T.);
#8108=EDGE_CURVE('',#6563,#6557,#337,.T.);
#8109=EDGE_CURVE('',#6562,#6564,#1135,.T.);
#8110=EDGE_CURVE('',#6564,#6565,#3694,.T.);
#8111=EDGE_CURVE('',#6565,#6563,#1136,.T.);
#8112=EDGE_CURVE('',#6566,#6567,#3695,.T.);
#8113=EDGE_CURVE('',#6567,#6568,#5829,.T.);
#8114=EDGE_CURVE('',#6568,#6569,#1137,.F.);
#8115=EDGE_CURVE('',#6569,#6566,#5830,.T.);
#8116=EDGE_CURVE('',#6566,#6565,#1138,.T.);
#8117=EDGE_CURVE('',#6564,#6567,#1139,.T.);
#8118=EDGE_CURVE('',#6559,#6570,#1140,.T.);
#8119=EDGE_CURVE('',#6570,#6561,#1141,.T.);
#8120=EDGE_CURVE('',#6566,#6571,#5831,.T.);
#8121=EDGE_CURVE('',#6571,#6572,#5832,.F.);
#8122=EDGE_CURVE('',#6572,#6570,#5833,.T.);
#8123=EDGE_CURVE('',#6573,#6551,#5834,.T.);
#8124=EDGE_CURVE('',#6574,#6573,#5835,.T.);
#8125=EDGE_CURVE('',#6575,#6574,#3696,.T.);
#8126=EDGE_CURVE('',#6576,#6575,#5836,.T.);
#8127=EDGE_CURVE('',#6577,#6576,#5837,.T.);
#8128=EDGE_CURVE('',#6578,#6577,#5838,.T.);
#8129=EDGE_CURVE('',#6579,#6578,#3697,.T.);
#8130=EDGE_CURVE('',#6580,#6579,#3698,.T.);
#8131=EDGE_CURVE('',#6581,#6580,#3699,.T.);
#8132=EDGE_CURVE('',#6582,#6581,#5839,.T.);
#8133=EDGE_CURVE('',#6583,#6582,#5840,.T.);
#8134=EDGE_CURVE('',#6584,#6583,#5841,.T.);
#8135=EDGE_CURVE('',#6585,#6584,#3700,.T.);
#8136=EDGE_CURVE('',#6571,#6585,#5842,.T.);
#8137=EDGE_CURVE('',#6486,#6569,#3701,.T.);
#8138=EDGE_CURVE('',#6485,#6548,#3702,.T.);
#8139=EDGE_CURVE('',#6586,#6586,#5843,.T.);
#8140=EDGE_CURVE('',#6586,#6587,#3703,.T.);
#8141=EDGE_CURVE('',#6587,#6587,#5844,.T.);
#8142=EDGE_CURVE('',#6588,#6589,#3704,.T.);
#8143=EDGE_CURVE('',#6590,#6588,#3705,.T.);
#8144=EDGE_CURVE('',#6591,#6590,#3706,.T.);
#8145=EDGE_CURVE('',#6589,#6591,#3707,.T.);
#8146=EDGE_CURVE('',#6592,#6592,#5845,.T.);
#8147=EDGE_CURVE('',#6593,#6593,#5846,.T.);
#8148=EDGE_CURVE('',#6594,#6594,#5847,.T.);
#8149=EDGE_CURVE('',#6595,#6595,#5848,.T.);
#8150=EDGE_CURVE('',#6587,#6596,#3708,.T.);
#8151=EDGE_CURVE('',#6596,#6596,#5849,.T.);
#8152=EDGE_CURVE('',#6592,#6597,#3709,.T.);
#8153=EDGE_CURVE('',#6597,#6597,#5850,.T.);
#8154=EDGE_CURVE('',#6597,#6598,#3710,.T.);
#8155=EDGE_CURVE('',#6598,#6598,#5851,.T.);
#8156=EDGE_CURVE('',#6595,#6599,#3711,.T.);
#8157=EDGE_CURVE('',#6599,#6599,#5852,.T.);
#8158=EDGE_CURVE('',#6599,#6600,#3712,.T.);
#8159=EDGE_CURVE('',#6600,#6600,#5853,.T.);
#8160=EDGE_CURVE('',#6593,#6601,#3713,.T.);
#8161=EDGE_CURVE('',#6601,#6601,#5854,.T.);
#8162=EDGE_CURVE('',#6601,#6602,#3714,.T.);
#8163=EDGE_CURVE('',#6602,#6602,#5855,.T.);
#8164=EDGE_CURVE('',#6594,#6603,#3715,.T.);
#8165=EDGE_CURVE('',#6603,#6603,#5856,.T.);
#8166=EDGE_CURVE('',#6603,#6604,#3716,.T.);
#8167=EDGE_CURVE('',#6605,#6604,#1142,.T.);
#8168=EDGE_CURVE('',#6605,#6605,#5857,.T.);
#8169=EDGE_CURVE('',#6606,#6605,#1143,.T.);
#8170=EDGE_CURVE('',#6604,#6606,#1144,.T.);
#8171=EDGE_CURVE('',#6606,#6607,#5858,.T.);
#8172=EDGE_CURVE('',#6607,#6607,#1145,.T.);
#8173=EDGE_CURVE('',#6608,#6608,#5859,.T.);
#8174=EDGE_CURVE('',#6608,#6607,#3717,.T.);
#8175=EDGE_CURVE('',#6609,#6610,#5860,.T.);
#8176=EDGE_CURVE('',#6610,#6611,#3718,.T.);
#8177=EDGE_CURVE('',#6611,#6612,#1146,.F.);
#8178=EDGE_CURVE('',#6612,#6609,#3719,.T.);
#8179=EDGE_CURVE('',#6588,#6613,#5861,.F.);
#8180=EDGE_CURVE('',#6614,#6588,#5862,.F.);
#8181=EDGE_CURVE('',#6613,#6614,#5863,.F.);
#8182=EDGE_CURVE('',#6589,#6609,#5864,.T.);
#8183=EDGE_CURVE('',#6609,#6614,#3720,.T.);
#8184=EDGE_CURVE('',#6615,#6616,#1147,.F.);
#8185=EDGE_CURVE('',#6616,#6613,#3721,.T.);
#8186=EDGE_CURVE('',#6614,#6615,#3722,.T.);
#8187=EDGE_CURVE('',#6617,#6590,#5865,.T.);
#8188=EDGE_CURVE('',#6613,#6617,#3723,.T.);
#8189=EDGE_CURVE('',#6589,#6610,#5866,.T.);
#8190=EDGE_CURVE('',#6580,#6617,#5867,.T.);
#8191=EDGE_CURVE('',#6617,#6618,#3724,.T.);
#8192=EDGE_CURVE('',#6618,#6581,#1148,.F.);
#8193=EDGE_CURVE('',#6580,#6590,#5868,.T.);
#8194=EDGE_CURVE('',#6619,#6610,#3725,.T.);
#8195=EDGE_CURVE('',#6620,#6619,#3726,.T.);
#8196=EDGE_CURVE('',#6611,#6620,#3727,.T.);
#8197=EDGE_CURVE('',#6591,#6619,#5869,.T.);
#8198=EDGE_CURVE('',#6591,#6579,#5870,.T.);
#8199=EDGE_CURVE('',#6536,#6505,#5871,.F.);
#8200=EDGE_CURVE('',#6621,#6537,#5872,.F.);
#8201=EDGE_CURVE('',#6535,#6621,#5873,.F.);
#8202=EDGE_CURVE('',#6622,#6623,#1149,.F.);
#8203=EDGE_CURVE('',#6623,#6621,#3728,.T.);
#8204=EDGE_CURVE('',#6537,#6622,#3729,.T.);
#8205=EDGE_CURVE('',#6621,#6624,#3730,.T.);
#8206=EDGE_CURVE('',#6624,#6484,#5874,.T.);
#8207=EDGE_CURVE('',#6484,#6509,#3731,.T.);
#8208=EDGE_CURVE('',#6624,#6485,#5875,.T.);
#8209=EDGE_CURVE('',#6486,#6504,#5876,.T.);
#8210=EDGE_CURVE('',#6625,#6626,#1150,.F.);
#8211=EDGE_CURVE('',#6626,#6536,#3732,.T.);
#8212=EDGE_CURVE('',#6505,#6625,#3733,.T.);
#8213=EDGE_CURVE('',#6624,#6553,#3734,.T.);
#8214=EDGE_CURVE('',#6554,#6623,#3735,.T.);
#8215=EDGE_CURVE('',#6627,#6612,#5877,.T.);
#8216=EDGE_CURVE('',#6628,#6627,#3736,.T.);
#8217=EDGE_CURVE('',#6622,#6628,#5878,.T.);
#8218=EDGE_CURVE('',#6629,#6626,#5879,.T.);
#8219=EDGE_CURVE('',#6630,#6629,#3737,.T.);
#8220=EDGE_CURVE('',#6615,#6630,#5880,.T.);
#8221=EDGE_CURVE('',#6631,#6631,#5881,.T.);
#8222=EDGE_CURVE('',#6632,#6632,#5882,.T.);
#8223=EDGE_CURVE('',#6633,#6633,#5883,.T.);
#8224=EDGE_CURVE('',#6634,#6634,#5884,.T.);
#8225=EDGE_CURVE('',#6635,#6635,#5885,.T.);
#8226=EDGE_CURVE('',#6631,#6636,#5886,.T.);
#8227=EDGE_CURVE('',#6636,#6637,#5887,.T.);
#8228=EDGE_CURVE('',#6637,#6636,#5888,.T.);
#8229=EDGE_CURVE('',#6637,#6638,#3738,.T.);
#8230=EDGE_CURVE('',#6638,#6638,#5889,.T.);
#8231=EDGE_CURVE('',#6628,#6639,#5890,.T.);
#8232=EDGE_CURVE('',#6639,#6623,#5891,.T.);
#8233=EDGE_CURVE('',#6627,#6640,#5892,.T.);
#8234=EDGE_CURVE('',#6640,#6639,#3739,.T.);
#8235=EDGE_CURVE('',#6611,#6640,#5893,.T.);
#8236=EDGE_CURVE('',#6464,#6641,#5894,.T.);
#8237=EDGE_CURVE('',#6641,#6642,#1151,.T.);
#8238=EDGE_CURVE('',#6642,#6463,#5895,.T.);
#8239=EDGE_CURVE('',#6642,#6641,#1152,.T.);
#8240=EDGE_CURVE('',#6643,#6643,#5896,.T.);
#8241=EDGE_CURVE('',#6554,#6644,#5897,.T.);
#8242=EDGE_CURVE('',#6644,#6645,#1153,.F.);
#8243=EDGE_CURVE('',#6645,#6555,#5898,.T.);
#8244=EDGE_CURVE('',#6646,#6645,#5899,.F.);
#8245=EDGE_CURVE('',#6556,#6646,#5900,.T.);
#8246=EDGE_CURVE('',#6647,#6647,#5901,.T.);
#8247=EDGE_CURVE('',#6648,#6649,#1154,.F.);
#8248=EDGE_CURVE('',#6649,#6650,#5902,.T.);
#8249=EDGE_CURVE('',#6650,#6651,#1155,.F.);
#8250=EDGE_CURVE('',#6651,#6648,#5903,.T.);
#8251=EDGE_CURVE('',#6652,#6651,#3740,.T.);
#8252=EDGE_CURVE('',#6653,#6652,#5904,.T.);
#8253=EDGE_CURVE('',#6654,#6653,#3741,.T.);
#8254=EDGE_CURVE('',#6625,#6654,#5905,.T.);
#8255=EDGE_CURVE('',#6625,#6648,#3742,.T.);
#8256=EDGE_CURVE('',#6655,#6656,#1156,.F.);
#8257=EDGE_CURVE('',#6656,#6657,#5906,.T.);
#8258=EDGE_CURVE('',#6657,#6658,#1157,.F.);
#8259=EDGE_CURVE('',#6658,#6655,#5907,.T.);
#8260=EDGE_CURVE('',#6659,#6656,#5908,.F.);
#8261=EDGE_CURVE('',#6660,#6659,#5909,.T.);
#8262=EDGE_CURVE('',#6657,#6660,#5910,.F.);
#8263=EDGE_CURVE('',#6661,#6661,#5911,.T.);
#8264=EDGE_CURVE('',#6662,#6663,#1158,.F.);
#8265=EDGE_CURVE('',#6663,#6664,#5912,.T.);
#8266=EDGE_CURVE('',#6664,#6665,#1159,.F.);
#8267=EDGE_CURVE('',#6665,#6662,#5913,.T.);
#8268=EDGE_CURVE('',#6666,#6663,#5914,.F.);
#8269=EDGE_CURVE('',#6667,#6666,#5915,.T.);
#8270=EDGE_CURVE('',#6664,#6667,#5916,.F.);
#8271=EDGE_CURVE('',#6668,#6668,#5917,.T.);
#8272=EDGE_CURVE('',#6669,#6630,#5918,.T.);
#8273=EDGE_CURVE('',#6629,#6654,#5919,.T.);
#8274=EDGE_CURVE('',#6654,#6669,#3743,.T.);
#8275=EDGE_CURVE('',#6669,#6616,#5920,.T.);
#8276=EDGE_CURVE('',#6670,#6665,#3744,.T.);
#8277=EDGE_CURVE('',#6618,#6670,#5921,.T.);
#8278=EDGE_CURVE('',#6618,#6616,#3745,.T.);
#8279=EDGE_CURVE('',#6669,#6671,#3746,.T.);
#8280=EDGE_CURVE('',#6672,#6671,#5922,.T.);
#8281=EDGE_CURVE('',#6662,#6672,#3747,.T.);
#8282=EDGE_CURVE('',#6671,#6653,#3748,.T.);
#8283=EDGE_CURVE('',#6673,#6574,#5923,.T.);
#8284=EDGE_CURVE('',#6573,#6674,#5924,.T.);
#8285=EDGE_CURVE('',#6674,#6673,#5925,.T.);
#8286=EDGE_CURVE('',#6675,#6575,#5926,.T.);
#8287=EDGE_CURVE('',#6673,#6675,#3749,.T.);
#8288=EDGE_CURVE('',#6676,#6576,#5927,.T.);
#8289=EDGE_CURVE('',#6675,#6676,#5928,.T.);
#8290=EDGE_CURVE('',#6676,#6677,#5929,.T.);
#8291=EDGE_CURVE('',#6677,#6576,#5930,.T.);
#8292=EDGE_CURVE('',#6573,#6678,#5931,.T.);
#8293=EDGE_CURVE('',#6678,#6674,#5932,.T.);
#8294=EDGE_CURVE('',#6677,#6679,#5933,.T.);
#8295=EDGE_CURVE('',#6679,#6577,#5934,.F.);
#8296=EDGE_CURVE('',#6676,#6658,#3750,.T.);
#8297=EDGE_CURVE('',#6660,#6677,#3751,.T.);
#8298=EDGE_CURVE('',#6680,#6620,#5935,.T.);
#8299=EDGE_CURVE('',#6655,#6680,#3752,.T.);
#8300=EDGE_CURVE('',#6640,#6675,#3753,.T.);
#8301=EDGE_CURVE('',#6639,#6673,#3754,.T.);
#8302=EDGE_CURVE('',#6644,#6674,#3755,.T.);
#8303=EDGE_CURVE('',#6568,#6681,#1160,.F.);
#8304=EDGE_CURVE('',#6681,#6504,#3756,.T.);
#8305=EDGE_CURVE('',#6648,#6681,#3757,.T.);
#8306=EDGE_CURVE('',#6619,#6579,#5936,.T.);
#8307=EDGE_CURVE('',#6578,#6620,#1161,.F.);
#8308=EDGE_CURVE('',#6552,#6678,#5937,.T.);
#8309=EDGE_CURVE('',#6678,#6646,#3758,.T.);
#8310=EDGE_CURVE('',#6570,#6682,#3759,.T.);
#8311=EDGE_CURVE('',#6649,#6682,#5938,.T.);
#8312=EDGE_CURVE('',#6683,#6572,#3760,.T.);
#8313=EDGE_CURVE('',#6683,#6682,#5939,.T.);
#8314=EDGE_CURVE('',#6684,#6670,#5940,.F.);
#8315=EDGE_CURVE('',#6582,#6684,#5941,.F.);
#8316=EDGE_CURVE('',#6670,#6582,#5942,.F.);
#8317=EDGE_CURVE('',#6672,#6685,#5943,.F.);
#8318=EDGE_CURVE('',#6583,#6672,#5944,.F.);
#8319=EDGE_CURVE('',#6685,#6583,#5945,.F.);
#8320=EDGE_CURVE('',#6572,#6652,#5946,.F.);
#8321=EDGE_CURVE('',#6652,#6571,#5947,.F.);
#8322=EDGE_CURVE('',#6671,#6584,#5948,.T.);
#8323=EDGE_CURVE('',#6653,#6585,#5949,.T.);
#8324=EDGE_CURVE('',#6650,#6683,#5950,.F.);
#8325=EDGE_CURVE('',#6684,#6685,#5951,.T.);
#8326=EDGE_CURVE('',#6685,#6666,#3761,.T.);
#8327=EDGE_CURVE('',#6667,#6684,#3762,.T.);
#8328=EDGE_CURVE('',#6680,#6679,#5952,.F.);
#8329=EDGE_CURVE('',#6577,#6680,#5953,.F.);
#8330=EDGE_CURVE('',#6679,#6659,#3763,.T.);
#8331=EDGE_CURVE('',#6661,#6635,#3764,.T.);
#8332=EDGE_CURVE('',#6686,#6686,#5954,.T.);
#8333=EDGE_CURVE('',#6686,#6634,#3765,.T.);
#8334=EDGE_CURVE('',#6668,#6633,#3766,.T.);
#8335=EDGE_CURVE('',#6647,#6632,#3767,.T.);
#8336=EDGE_CURVE('',#6643,#6687,#3768,.T.);
#8337=EDGE_CURVE('',#6687,#6687,#5955,.T.);
#8338=EDGE_CURVE('',#6688,#6688,#5956,.T.);
#8339=EDGE_CURVE('',#6688,#6450,#3769,.T.);
#10371=ORIENTED_EDGE('',*,*,#7934,.T.);
#10372=ORIENTED_EDGE('',*,*,#7935,.T.);
#10373=ORIENTED_EDGE('',*,*,#7936,.T.);
#10374=ORIENTED_EDGE('',*,*,#7937,.T.);
#10375=ORIENTED_EDGE('',*,*,#7935,.F.);
#10376=ORIENTED_EDGE('',*,*,#7938,.F.);
#10377=ORIENTED_EDGE('',*,*,#7934,.F.);
#10378=ORIENTED_EDGE('',*,*,#7936,.F.);
#10379=ORIENTED_EDGE('',*,*,#7937,.F.);
#10380=ORIENTED_EDGE('',*,*,#7939,.T.);
#10381=ORIENTED_EDGE('',*,*,#7940,.T.);
#10382=ORIENTED_EDGE('',*,*,#7939,.F.);
#10383=ORIENTED_EDGE('',*,*,#7941,.T.);
#10384=ORIENTED_EDGE('',*,*,#7942,.T.);
#10385=ORIENTED_EDGE('',*,*,#7943,.T.);
#10386=ORIENTED_EDGE('',*,*,#7942,.F.);
#10387=ORIENTED_EDGE('',*,*,#7944,.F.);
#10388=ORIENTED_EDGE('',*,*,#7945,.F.);
#10389=ORIENTED_EDGE('',*,*,#7946,.F.);
#10390=ORIENTED_EDGE('',*,*,#7947,.F.);
#10391=ORIENTED_EDGE('',*,*,#7948,.F.);
#10392=ORIENTED_EDGE('',*,*,#7949,.F.);
#10393=ORIENTED_EDGE('',*,*,#7950,.F.);
#10394=ORIENTED_EDGE('',*,*,#7951,.F.);
#10395=ORIENTED_EDGE('',*,*,#7941,.F.);
#10396=ORIENTED_EDGE('',*,*,#7943,.F.);
#10397=ORIENTED_EDGE('',*,*,#7952,.T.);
#10398=ORIENTED_EDGE('',*,*,#7953,.F.);
#10399=ORIENTED_EDGE('',*,*,#7954,.T.);
#10400=ORIENTED_EDGE('',*,*,#7955,.F.);
#10401=ORIENTED_EDGE('',*,*,#7956,.F.);
#10402=ORIENTED_EDGE('',*,*,#7952,.F.);
#10403=ORIENTED_EDGE('',*,*,#7957,.T.);
#10404=ORIENTED_EDGE('',*,*,#7958,.T.);
#10405=ORIENTED_EDGE('',*,*,#7959,.T.);
#10406=ORIENTED_EDGE('',*,*,#7960,.T.);
#10407=ORIENTED_EDGE('',*,*,#7944,.T.);
#10408=ORIENTED_EDGE('',*,*,#7961,.T.);
#10409=ORIENTED_EDGE('',*,*,#7962,.T.);
#10410=ORIENTED_EDGE('',*,*,#7963,.T.);
#10411=ORIENTED_EDGE('',*,*,#7964,.T.);
#10412=ORIENTED_EDGE('',*,*,#7963,.F.);
#10413=ORIENTED_EDGE('',*,*,#7965,.T.);
#10414=ORIENTED_EDGE('',*,*,#7960,.F.);
#10415=ORIENTED_EDGE('',*,*,#7966,.T.);
#10416=ORIENTED_EDGE('',*,*,#7967,.T.);
#10417=ORIENTED_EDGE('',*,*,#7968,.T.);
#10418=ORIENTED_EDGE('',*,*,#7969,.T.);
#10419=ORIENTED_EDGE('',*,*,#7970,.T.);
#10420=ORIENTED_EDGE('',*,*,#7967,.F.);
#10421=ORIENTED_EDGE('',*,*,#7971,.T.);
#10422=ORIENTED_EDGE('',*,*,#7961,.F.);
#10423=ORIENTED_EDGE('',*,*,#7972,.T.);
#10424=ORIENTED_EDGE('',*,*,#7973,.T.);
#10425=ORIENTED_EDGE('',*,*,#7974,.T.);
#10426=ORIENTED_EDGE('',*,*,#7975,.T.);
#10427=ORIENTED_EDGE('',*,*,#7976,.T.);
#10428=ORIENTED_EDGE('',*,*,#7975,.F.);
#10429=ORIENTED_EDGE('',*,*,#7977,.T.);
#10430=ORIENTED_EDGE('',*,*,#7969,.F.);
#10431=ORIENTED_EDGE('',*,*,#7978,.T.);
#10432=ORIENTED_EDGE('',*,*,#7957,.F.);
#10433=ORIENTED_EDGE('',*,*,#7979,.T.);
#10434=ORIENTED_EDGE('',*,*,#7973,.F.);
#10435=ORIENTED_EDGE('',*,*,#7980,.T.);
#10436=ORIENTED_EDGE('',*,*,#7970,.F.);
#10437=ORIENTED_EDGE('',*,*,#7981,.F.);
#10438=ORIENTED_EDGE('',*,*,#7982,.F.);
#10439=ORIENTED_EDGE('',*,*,#7977,.F.);
#10440=ORIENTED_EDGE('',*,*,#7974,.F.);
#10441=ORIENTED_EDGE('',*,*,#7979,.F.);
#10442=ORIENTED_EDGE('',*,*,#7951,.T.);
#10443=ORIENTED_EDGE('',*,*,#7983,.F.);
#10444=ORIENTED_EDGE('',*,*,#7984,.F.);
#10445=ORIENTED_EDGE('',*,*,#7985,.F.);
#10446=ORIENTED_EDGE('',*,*,#7986,.T.);
#10447=ORIENTED_EDGE('',*,*,#7987,.F.);
#10448=ORIENTED_EDGE('',*,*,#7988,.T.);
#10449=ORIENTED_EDGE('',*,*,#7989,.F.);
#10450=ORIENTED_EDGE('',*,*,#7981,.T.);
#10451=ORIENTED_EDGE('',*,*,#7976,.F.);
#10452=ORIENTED_EDGE('',*,*,#7978,.F.);
#10453=ORIENTED_EDGE('',*,*,#7968,.F.);
#10454=ORIENTED_EDGE('',*,*,#7972,.F.);
#10455=ORIENTED_EDGE('',*,*,#7964,.F.);
#10456=ORIENTED_EDGE('',*,*,#7966,.F.);
#10457=ORIENTED_EDGE('',*,*,#7959,.F.);
#10458=ORIENTED_EDGE('',*,*,#7990,.T.);
#10459=ORIENTED_EDGE('',*,*,#7991,.T.);
#10460=ORIENTED_EDGE('',*,*,#7990,.F.);
#10461=ORIENTED_EDGE('',*,*,#7958,.F.);
#10462=ORIENTED_EDGE('',*,*,#7980,.F.);
#10463=ORIENTED_EDGE('',*,*,#7992,.T.);
#10464=ORIENTED_EDGE('',*,*,#7993,.T.);
#10465=ORIENTED_EDGE('',*,*,#7994,.T.);
#10466=ORIENTED_EDGE('',*,*,#7946,.T.);
#10467=ORIENTED_EDGE('',*,*,#7995,.T.);
#10468=ORIENTED_EDGE('',*,*,#7996,.T.);
#10469=ORIENTED_EDGE('',*,*,#7997,.T.);
#10470=ORIENTED_EDGE('',*,*,#7998,.T.);
#10471=ORIENTED_EDGE('',*,*,#7999,.T.);
#10472=ORIENTED_EDGE('',*,*,#7997,.F.);
#10473=ORIENTED_EDGE('',*,*,#8000,.T.);
#10474=ORIENTED_EDGE('',*,*,#7994,.F.);
#10475=ORIENTED_EDGE('',*,*,#8001,.T.);
#10476=ORIENTED_EDGE('',*,*,#8002,.T.);
#10477=ORIENTED_EDGE('',*,*,#8003,.T.);
#10478=ORIENTED_EDGE('',*,*,#8004,.T.);
#10479=ORIENTED_EDGE('',*,*,#8005,.T.);
#10480=ORIENTED_EDGE('',*,*,#8002,.F.);
#10481=ORIENTED_EDGE('',*,*,#8006,.T.);
#10482=ORIENTED_EDGE('',*,*,#7995,.F.);
#10483=ORIENTED_EDGE('',*,*,#8007,.T.);
#10484=ORIENTED_EDGE('',*,*,#8008,.T.);
#10485=ORIENTED_EDGE('',*,*,#8009,.T.);
#10486=ORIENTED_EDGE('',*,*,#8010,.T.);
#10487=ORIENTED_EDGE('',*,*,#8011,.T.);
#10488=ORIENTED_EDGE('',*,*,#8010,.F.);
#10489=ORIENTED_EDGE('',*,*,#8012,.T.);
#10490=ORIENTED_EDGE('',*,*,#8004,.F.);
#10491=ORIENTED_EDGE('',*,*,#8013,.T.);
#10492=ORIENTED_EDGE('',*,*,#7992,.F.);
#10493=ORIENTED_EDGE('',*,*,#8014,.T.);
#10494=ORIENTED_EDGE('',*,*,#8008,.F.);
#10495=ORIENTED_EDGE('',*,*,#8015,.T.);
#10496=ORIENTED_EDGE('',*,*,#8005,.F.);
#10497=ORIENTED_EDGE('',*,*,#8016,.F.);
#10498=ORIENTED_EDGE('',*,*,#8017,.F.);
#10499=ORIENTED_EDGE('',*,*,#7971,.F.);
#10500=ORIENTED_EDGE('',*,*,#7982,.T.);
#10501=ORIENTED_EDGE('',*,*,#8018,.T.);
#10502=ORIENTED_EDGE('',*,*,#8019,.T.);
#10503=ORIENTED_EDGE('',*,*,#8020,.T.);
#10504=ORIENTED_EDGE('',*,*,#8016,.T.);
#10505=ORIENTED_EDGE('',*,*,#8012,.F.);
#10506=ORIENTED_EDGE('',*,*,#8009,.F.);
#10507=ORIENTED_EDGE('',*,*,#8014,.F.);
#10508=ORIENTED_EDGE('',*,*,#7945,.T.);
#10509=ORIENTED_EDGE('',*,*,#7965,.F.);
#10510=ORIENTED_EDGE('',*,*,#7962,.F.);
#10511=ORIENTED_EDGE('',*,*,#8011,.F.);
#10512=ORIENTED_EDGE('',*,*,#8013,.F.);
#10513=ORIENTED_EDGE('',*,*,#8003,.F.);
#10514=ORIENTED_EDGE('',*,*,#8007,.F.);
#10515=ORIENTED_EDGE('',*,*,#7999,.F.);
#10516=ORIENTED_EDGE('',*,*,#8021,.T.);
#10517=ORIENTED_EDGE('',*,*,#8022,.T.);
#10518=ORIENTED_EDGE('',*,*,#8021,.F.);
#10519=ORIENTED_EDGE('',*,*,#7998,.F.);
#10520=ORIENTED_EDGE('',*,*,#8001,.F.);
#10521=ORIENTED_EDGE('',*,*,#7993,.F.);
#10522=ORIENTED_EDGE('',*,*,#8015,.F.);
#10523=ORIENTED_EDGE('',*,*,#8023,.T.);
#10524=ORIENTED_EDGE('',*,*,#8024,.T.);
#10525=ORIENTED_EDGE('',*,*,#8025,.T.);
#10526=ORIENTED_EDGE('',*,*,#8026,.T.);
#10527=ORIENTED_EDGE('',*,*,#8027,.T.);
#10528=ORIENTED_EDGE('',*,*,#8028,.T.);
#10529=ORIENTED_EDGE('',*,*,#8029,.T.);
#10530=ORIENTED_EDGE('',*,*,#8030,.T.);
#10531=ORIENTED_EDGE('',*,*,#8029,.F.);
#10532=ORIENTED_EDGE('',*,*,#8031,.T.);
#10533=ORIENTED_EDGE('',*,*,#8025,.F.);
#10534=ORIENTED_EDGE('',*,*,#8032,.T.);
#10535=ORIENTED_EDGE('',*,*,#8033,.T.);
#10536=ORIENTED_EDGE('',*,*,#8034,.T.);
#10537=ORIENTED_EDGE('',*,*,#8035,.T.);
#10538=ORIENTED_EDGE('',*,*,#8036,.T.);
#10539=ORIENTED_EDGE('',*,*,#7950,.T.);
#10540=ORIENTED_EDGE('',*,*,#8033,.F.);
#10541=ORIENTED_EDGE('',*,*,#8037,.T.);
#10542=ORIENTED_EDGE('',*,*,#8027,.F.);
#10543=ORIENTED_EDGE('',*,*,#8038,.T.);
#10544=ORIENTED_EDGE('',*,*,#8039,.T.);
#10545=ORIENTED_EDGE('',*,*,#7984,.T.);
#10546=ORIENTED_EDGE('',*,*,#8040,.T.);
#10547=ORIENTED_EDGE('',*,*,#8041,.T.);
#10548=ORIENTED_EDGE('',*,*,#8040,.F.);
#10549=ORIENTED_EDGE('',*,*,#7983,.T.);
#10550=ORIENTED_EDGE('',*,*,#8036,.F.);
#10551=ORIENTED_EDGE('',*,*,#8042,.T.);
#10552=ORIENTED_EDGE('',*,*,#8023,.F.);
#10553=ORIENTED_EDGE('',*,*,#7985,.T.);
#10554=ORIENTED_EDGE('',*,*,#8039,.F.);
#10555=ORIENTED_EDGE('',*,*,#8043,.T.);
#10556=ORIENTED_EDGE('',*,*,#8041,.F.);
#10557=ORIENTED_EDGE('',*,*,#8042,.F.);
#10558=ORIENTED_EDGE('',*,*,#8035,.F.);
#10559=ORIENTED_EDGE('',*,*,#8044,.T.);
#10560=ORIENTED_EDGE('',*,*,#8045,.T.);
#10561=ORIENTED_EDGE('',*,*,#8044,.F.);
#10562=ORIENTED_EDGE('',*,*,#8034,.F.);
#10563=ORIENTED_EDGE('',*,*,#8038,.F.);
#10564=ORIENTED_EDGE('',*,*,#8030,.F.);
#10565=ORIENTED_EDGE('',*,*,#8032,.F.);
#10566=ORIENTED_EDGE('',*,*,#8024,.F.);
#10567=ORIENTED_EDGE('',*,*,#8043,.F.);
#10568=ORIENTED_EDGE('',*,*,#8046,.T.);
#10569=ORIENTED_EDGE('',*,*,#8047,.T.);
#10570=ORIENTED_EDGE('',*,*,#8048,.T.);
#10571=ORIENTED_EDGE('',*,*,#7948,.T.);
#10572=ORIENTED_EDGE('',*,*,#8049,.T.);
#10573=ORIENTED_EDGE('',*,*,#8050,.T.);
#10574=ORIENTED_EDGE('',*,*,#8051,.T.);
#10575=ORIENTED_EDGE('',*,*,#8052,.T.);
#10576=ORIENTED_EDGE('',*,*,#8051,.F.);
#10577=ORIENTED_EDGE('',*,*,#8053,.T.);
#10578=ORIENTED_EDGE('',*,*,#8048,.F.);
#10579=ORIENTED_EDGE('',*,*,#8054,.T.);
#10580=ORIENTED_EDGE('',*,*,#8055,.T.);
#10581=ORIENTED_EDGE('',*,*,#8056,.T.);
#10582=ORIENTED_EDGE('',*,*,#8057,.T.);
#10583=ORIENTED_EDGE('',*,*,#8058,.T.);
#10584=ORIENTED_EDGE('',*,*,#8055,.F.);
#10585=ORIENTED_EDGE('',*,*,#8059,.T.);
#10586=ORIENTED_EDGE('',*,*,#8049,.F.);
#10587=ORIENTED_EDGE('',*,*,#8060,.T.);
#10588=ORIENTED_EDGE('',*,*,#8061,.T.);
#10589=ORIENTED_EDGE('',*,*,#8062,.T.);
#10590=ORIENTED_EDGE('',*,*,#8063,.T.);
#10591=ORIENTED_EDGE('',*,*,#8064,.T.);
#10592=ORIENTED_EDGE('',*,*,#8065,.T.);
#10593=ORIENTED_EDGE('',*,*,#8063,.F.);
#10594=ORIENTED_EDGE('',*,*,#8066,.T.);
#10595=ORIENTED_EDGE('',*,*,#8057,.F.);
#10596=ORIENTED_EDGE('',*,*,#8067,.T.);
#10597=ORIENTED_EDGE('',*,*,#8046,.F.);
#10598=ORIENTED_EDGE('',*,*,#8068,.T.);
#10599=ORIENTED_EDGE('',*,*,#8061,.F.);
#10600=ORIENTED_EDGE('',*,*,#8069,.T.);
#10601=ORIENTED_EDGE('',*,*,#8058,.F.);
#10602=ORIENTED_EDGE('',*,*,#8070,.F.);
#10603=ORIENTED_EDGE('',*,*,#8071,.F.);
#10604=ORIENTED_EDGE('',*,*,#8006,.F.);
#10605=ORIENTED_EDGE('',*,*,#8017,.T.);
#10606=ORIENTED_EDGE('',*,*,#8072,.T.);
#10607=ORIENTED_EDGE('',*,*,#8073,.T.);
#10608=ORIENTED_EDGE('',*,*,#8074,.T.);
#10609=ORIENTED_EDGE('',*,*,#8070,.T.);
#10610=ORIENTED_EDGE('',*,*,#8066,.F.);
#10611=ORIENTED_EDGE('',*,*,#8062,.F.);
#10612=ORIENTED_EDGE('',*,*,#8068,.F.);
#10613=ORIENTED_EDGE('',*,*,#7947,.T.);
#10614=ORIENTED_EDGE('',*,*,#8000,.F.);
#10615=ORIENTED_EDGE('',*,*,#7996,.F.);
#10616=ORIENTED_EDGE('',*,*,#8064,.F.);
#10617=ORIENTED_EDGE('',*,*,#8067,.F.);
#10618=ORIENTED_EDGE('',*,*,#8056,.F.);
#10619=ORIENTED_EDGE('',*,*,#8060,.F.);
#10620=ORIENTED_EDGE('',*,*,#8052,.F.);
#10621=ORIENTED_EDGE('',*,*,#8054,.F.);
#10622=ORIENTED_EDGE('',*,*,#8047,.F.);
#10623=ORIENTED_EDGE('',*,*,#8069,.F.);
#10624=ORIENTED_EDGE('',*,*,#8065,.F.);
#10625=ORIENTED_EDGE('',*,*,#8075,.T.);
#10626=ORIENTED_EDGE('',*,*,#8076,.T.);
#10627=ORIENTED_EDGE('',*,*,#8075,.F.);
#10628=ORIENTED_EDGE('',*,*,#8077,.F.);
#10629=ORIENTED_EDGE('',*,*,#8078,.T.);
#10630=ORIENTED_EDGE('',*,*,#8079,.T.);
#10631=ORIENTED_EDGE('',*,*,#8080,.T.);
#10632=ORIENTED_EDGE('',*,*,#8079,.F.);
#10633=ORIENTED_EDGE('',*,*,#8081,.T.);
#10634=ORIENTED_EDGE('',*,*,#8082,.T.);
#10635=ORIENTED_EDGE('',*,*,#8083,.T.);
#10636=ORIENTED_EDGE('',*,*,#8077,.T.);
#10637=ORIENTED_EDGE('',*,*,#8084,.T.);
#10638=ORIENTED_EDGE('',*,*,#8085,.T.);
#10639=ORIENTED_EDGE('',*,*,#8086,.T.);
#10640=ORIENTED_EDGE('',*,*,#8087,.T.);
#10641=ORIENTED_EDGE('',*,*,#8088,.T.);
#10642=ORIENTED_EDGE('',*,*,#8089,.T.);
#10643=ORIENTED_EDGE('',*,*,#8090,.T.);
#10644=ORIENTED_EDGE('',*,*,#8091,.T.);
#10645=ORIENTED_EDGE('',*,*,#8090,.F.);
#10646=ORIENTED_EDGE('',*,*,#8092,.T.);
#10647=ORIENTED_EDGE('',*,*,#8082,.F.);
#10648=ORIENTED_EDGE('',*,*,#8093,.T.);
#10649=ORIENTED_EDGE('',*,*,#8085,.F.);
#10650=ORIENTED_EDGE('',*,*,#8094,.T.);
#10651=ORIENTED_EDGE('',*,*,#8095,.T.);
#10652=ORIENTED_EDGE('',*,*,#8086,.F.);
#10653=ORIENTED_EDGE('',*,*,#8094,.F.);
#10654=ORIENTED_EDGE('',*,*,#8084,.F.);
#10655=ORIENTED_EDGE('',*,*,#8080,.F.);
#10656=ORIENTED_EDGE('',*,*,#8083,.F.);
#10657=ORIENTED_EDGE('',*,*,#8092,.F.);
#10658=ORIENTED_EDGE('',*,*,#8089,.F.);
#10659=ORIENTED_EDGE('',*,*,#8096,.F.);
#10660=ORIENTED_EDGE('',*,*,#8097,.T.);
#10661=ORIENTED_EDGE('',*,*,#8098,.T.);
#10662=ORIENTED_EDGE('',*,*,#8099,.T.);
#10663=ORIENTED_EDGE('',*,*,#8100,.T.);
#10664=ORIENTED_EDGE('',*,*,#8101,.F.);
#10665=ORIENTED_EDGE('',*,*,#8102,.T.);
#10666=ORIENTED_EDGE('',*,*,#8103,.T.);
#10667=ORIENTED_EDGE('',*,*,#8104,.T.);
#10668=ORIENTED_EDGE('',*,*,#8105,.T.);
#10669=ORIENTED_EDGE('',*,*,#8101,.T.);
#10670=ORIENTED_EDGE('',*,*,#8106,.T.);
#10671=ORIENTED_EDGE('',*,*,#8107,.F.);
#10672=ORIENTED_EDGE('',*,*,#8108,.T.);
#10673=ORIENTED_EDGE('',*,*,#8107,.T.);
#10674=ORIENTED_EDGE('',*,*,#8109,.T.);
#10675=ORIENTED_EDGE('',*,*,#8110,.T.);
#10676=ORIENTED_EDGE('',*,*,#8111,.T.);
#10677=ORIENTED_EDGE('',*,*,#8112,.T.);
#10678=ORIENTED_EDGE('',*,*,#8113,.T.);
#10679=ORIENTED_EDGE('',*,*,#8114,.T.);
#10680=ORIENTED_EDGE('',*,*,#8115,.T.);
#10681=ORIENTED_EDGE('',*,*,#8112,.F.);
#10682=ORIENTED_EDGE('',*,*,#8116,.T.);
#10683=ORIENTED_EDGE('',*,*,#8110,.F.);
#10684=ORIENTED_EDGE('',*,*,#8117,.T.);
#10685=ORIENTED_EDGE('',*,*,#8103,.F.);
#10686=ORIENTED_EDGE('',*,*,#8118,.T.);
#10687=ORIENTED_EDGE('',*,*,#8119,.T.);
#10688=ORIENTED_EDGE('',*,*,#8104,.F.);
#10689=ORIENTED_EDGE('',*,*,#8118,.F.);
#10690=ORIENTED_EDGE('',*,*,#8102,.F.);
#10691=ORIENTED_EDGE('',*,*,#8108,.F.);
#10692=ORIENTED_EDGE('',*,*,#8111,.F.);
#10693=ORIENTED_EDGE('',*,*,#8116,.F.);
#10694=ORIENTED_EDGE('',*,*,#8120,.T.);
#10695=ORIENTED_EDGE('',*,*,#8121,.T.);
#10696=ORIENTED_EDGE('',*,*,#8122,.T.);
#10697=ORIENTED_EDGE('',*,*,#8091,.F.);
#10698=ORIENTED_EDGE('',*,*,#8123,.F.);
#10699=ORIENTED_EDGE('',*,*,#8124,.F.);
#10700=ORIENTED_EDGE('',*,*,#8125,.F.);
#10701=ORIENTED_EDGE('',*,*,#8126,.F.);
#10702=ORIENTED_EDGE('',*,*,#8127,.F.);
#10703=ORIENTED_EDGE('',*,*,#8128,.F.);
#10704=ORIENTED_EDGE('',*,*,#8129,.F.);
#10705=ORIENTED_EDGE('',*,*,#8130,.F.);
#10706=ORIENTED_EDGE('',*,*,#8131,.F.);
#10707=ORIENTED_EDGE('',*,*,#8132,.F.);
#10708=ORIENTED_EDGE('',*,*,#8133,.F.);
#10709=ORIENTED_EDGE('',*,*,#8134,.F.);
#10710=ORIENTED_EDGE('',*,*,#8135,.F.);
#10711=ORIENTED_EDGE('',*,*,#8136,.F.);
#10712=ORIENTED_EDGE('',*,*,#8120,.F.);
#10713=ORIENTED_EDGE('',*,*,#8115,.F.);
#10714=ORIENTED_EDGE('',*,*,#8137,.F.);
#10715=ORIENTED_EDGE('',*,*,#7988,.F.);
#10716=ORIENTED_EDGE('',*,*,#8138,.T.);
#10717=ORIENTED_EDGE('',*,*,#8139,.T.);
#10718=ORIENTED_EDGE('',*,*,#8140,.T.);
#10719=ORIENTED_EDGE('',*,*,#8141,.T.);
#10720=ORIENTED_EDGE('',*,*,#8140,.F.);
#10721=ORIENTED_EDGE('',*,*,#8142,.F.);
#10722=ORIENTED_EDGE('',*,*,#8143,.F.);
#10723=ORIENTED_EDGE('',*,*,#8144,.F.);
#10724=ORIENTED_EDGE('',*,*,#8145,.F.);
#10725=ORIENTED_EDGE('',*,*,#8146,.F.);
#10726=ORIENTED_EDGE('',*,*,#8147,.F.);
#10727=ORIENTED_EDGE('',*,*,#8148,.F.);
#10728=ORIENTED_EDGE('',*,*,#8149,.F.);
#10729=ORIENTED_EDGE('',*,*,#8139,.F.);
#10730=ORIENTED_EDGE('',*,*,#8141,.F.);
#10731=ORIENTED_EDGE('',*,*,#8150,.T.);
#10732=ORIENTED_EDGE('',*,*,#8151,.T.);
#10733=ORIENTED_EDGE('',*,*,#8150,.F.);
#10734=ORIENTED_EDGE('',*,*,#8146,.T.);
#10735=ORIENTED_EDGE('',*,*,#8152,.T.);
#10736=ORIENTED_EDGE('',*,*,#8153,.T.);
#10737=ORIENTED_EDGE('',*,*,#8152,.F.);
#10738=ORIENTED_EDGE('',*,*,#8153,.F.);
#10739=ORIENTED_EDGE('',*,*,#8154,.T.);
#10740=ORIENTED_EDGE('',*,*,#8155,.T.);
#10741=ORIENTED_EDGE('',*,*,#8154,.F.);
#10742=ORIENTED_EDGE('',*,*,#8149,.T.);
#10743=ORIENTED_EDGE('',*,*,#8156,.T.);
#10744=ORIENTED_EDGE('',*,*,#8157,.T.);
#10745=ORIENTED_EDGE('',*,*,#8156,.F.);
#10746=ORIENTED_EDGE('',*,*,#8157,.F.);
#10747=ORIENTED_EDGE('',*,*,#8158,.T.);
#10748=ORIENTED_EDGE('',*,*,#8159,.T.);
#10749=ORIENTED_EDGE('',*,*,#8158,.F.);
#10750=ORIENTED_EDGE('',*,*,#8147,.T.);
#10751=ORIENTED_EDGE('',*,*,#8160,.T.);
#10752=ORIENTED_EDGE('',*,*,#8161,.T.);
#10753=ORIENTED_EDGE('',*,*,#8160,.F.);
#10754=ORIENTED_EDGE('',*,*,#8161,.F.);
#10755=ORIENTED_EDGE('',*,*,#8162,.T.);
#10756=ORIENTED_EDGE('',*,*,#8163,.T.);
#10757=ORIENTED_EDGE('',*,*,#8162,.F.);
#10758=ORIENTED_EDGE('',*,*,#8148,.T.);
#10759=ORIENTED_EDGE('',*,*,#8164,.T.);
#10760=ORIENTED_EDGE('',*,*,#8165,.T.);
#10761=ORIENTED_EDGE('',*,*,#8164,.F.);
#10762=ORIENTED_EDGE('',*,*,#8165,.F.);
#10763=ORIENTED_EDGE('',*,*,#8166,.T.);
#10764=ORIENTED_EDGE('',*,*,#8167,.F.);
#10765=ORIENTED_EDGE('',*,*,#8168,.T.);
#10766=ORIENTED_EDGE('',*,*,#8169,.F.);
#10767=ORIENTED_EDGE('',*,*,#8170,.F.);
#10768=ORIENTED_EDGE('',*,*,#8166,.F.);
#10769=ORIENTED_EDGE('',*,*,#8171,.T.);
#10770=ORIENTED_EDGE('',*,*,#8172,.T.);
#10771=ORIENTED_EDGE('',*,*,#8171,.F.);
#10772=ORIENTED_EDGE('',*,*,#8169,.T.);
#10773=ORIENTED_EDGE('',*,*,#8167,.T.);
#10774=ORIENTED_EDGE('',*,*,#8170,.T.);
#10775=ORIENTED_EDGE('',*,*,#8173,.F.);
#10776=ORIENTED_EDGE('',*,*,#8174,.T.);
#10777=ORIENTED_EDGE('',*,*,#8172,.F.);
#10778=ORIENTED_EDGE('',*,*,#8174,.F.);
#10779=ORIENTED_EDGE('',*,*,#8175,.T.);
#10780=ORIENTED_EDGE('',*,*,#8176,.T.);
#10781=ORIENTED_EDGE('',*,*,#8177,.T.);
#10782=ORIENTED_EDGE('',*,*,#8178,.T.);
#10783=ORIENTED_EDGE('',*,*,#8179,.F.);
#10784=ORIENTED_EDGE('',*,*,#8180,.F.);
#10785=ORIENTED_EDGE('',*,*,#8181,.F.);
#10786=ORIENTED_EDGE('',*,*,#8182,.T.);
#10787=ORIENTED_EDGE('',*,*,#8183,.T.);
#10788=ORIENTED_EDGE('',*,*,#8180,.T.);
#10789=ORIENTED_EDGE('',*,*,#8142,.T.);
#10790=ORIENTED_EDGE('',*,*,#8184,.T.);
#10791=ORIENTED_EDGE('',*,*,#8185,.T.);
#10792=ORIENTED_EDGE('',*,*,#8181,.T.);
#10793=ORIENTED_EDGE('',*,*,#8186,.T.);
#10794=ORIENTED_EDGE('',*,*,#8187,.T.);
#10795=ORIENTED_EDGE('',*,*,#8143,.T.);
#10796=ORIENTED_EDGE('',*,*,#8179,.T.);
#10797=ORIENTED_EDGE('',*,*,#8188,.T.);
#10798=ORIENTED_EDGE('',*,*,#8182,.F.);
#10799=ORIENTED_EDGE('',*,*,#8189,.T.);
#10800=ORIENTED_EDGE('',*,*,#8175,.F.);
#10801=ORIENTED_EDGE('',*,*,#8190,.T.);
#10802=ORIENTED_EDGE('',*,*,#8191,.T.);
#10803=ORIENTED_EDGE('',*,*,#8192,.T.);
#10804=ORIENTED_EDGE('',*,*,#8131,.T.);
#10805=ORIENTED_EDGE('',*,*,#8190,.F.);
#10806=ORIENTED_EDGE('',*,*,#8193,.T.);
#10807=ORIENTED_EDGE('',*,*,#8187,.F.);
#10808=ORIENTED_EDGE('',*,*,#8176,.F.);
#10809=ORIENTED_EDGE('',*,*,#8194,.F.);
#10810=ORIENTED_EDGE('',*,*,#8195,.F.);
#10811=ORIENTED_EDGE('',*,*,#8196,.F.);
#10812=ORIENTED_EDGE('',*,*,#8189,.F.);
#10813=ORIENTED_EDGE('',*,*,#8145,.T.);
#10814=ORIENTED_EDGE('',*,*,#8197,.T.);
#10815=ORIENTED_EDGE('',*,*,#8194,.T.);
#10816=ORIENTED_EDGE('',*,*,#8193,.F.);
#10817=ORIENTED_EDGE('',*,*,#8130,.T.);
#10818=ORIENTED_EDGE('',*,*,#8198,.F.);
#10819=ORIENTED_EDGE('',*,*,#8144,.T.);
#10820=ORIENTED_EDGE('',*,*,#8199,.F.);
#10821=ORIENTED_EDGE('',*,*,#8072,.F.);
#10822=ORIENTED_EDGE('',*,*,#8020,.F.);
#10823=ORIENTED_EDGE('',*,*,#8074,.F.);
#10824=ORIENTED_EDGE('',*,*,#8200,.F.);
#10825=ORIENTED_EDGE('',*,*,#8201,.F.);
#10826=ORIENTED_EDGE('',*,*,#8202,.T.);
#10827=ORIENTED_EDGE('',*,*,#8203,.T.);
#10828=ORIENTED_EDGE('',*,*,#8200,.T.);
#10829=ORIENTED_EDGE('',*,*,#8204,.T.);
#10830=ORIENTED_EDGE('',*,*,#8037,.F.);
#10831=ORIENTED_EDGE('',*,*,#7949,.T.);
#10832=ORIENTED_EDGE('',*,*,#8053,.F.);
#10833=ORIENTED_EDGE('',*,*,#8050,.F.);
#10834=ORIENTED_EDGE('',*,*,#8059,.F.);
#10835=ORIENTED_EDGE('',*,*,#8071,.T.);
#10836=ORIENTED_EDGE('',*,*,#8201,.T.);
#10837=ORIENTED_EDGE('',*,*,#8205,.T.);
#10838=ORIENTED_EDGE('',*,*,#8206,.T.);
#10839=ORIENTED_EDGE('',*,*,#8207,.T.);
#10840=ORIENTED_EDGE('',*,*,#8031,.F.);
#10841=ORIENTED_EDGE('',*,*,#8028,.F.);
#10842=ORIENTED_EDGE('',*,*,#8206,.F.);
#10843=ORIENTED_EDGE('',*,*,#8208,.T.);
#10844=ORIENTED_EDGE('',*,*,#7987,.T.);
#10845=ORIENTED_EDGE('',*,*,#8018,.F.);
#10846=ORIENTED_EDGE('',*,*,#7989,.T.);
#10847=ORIENTED_EDGE('',*,*,#8209,.T.);
#10848=ORIENTED_EDGE('',*,*,#8210,.T.);
#10849=ORIENTED_EDGE('',*,*,#8211,.T.);
#10850=ORIENTED_EDGE('',*,*,#8199,.T.);
#10851=ORIENTED_EDGE('',*,*,#8212,.T.);
#10852=ORIENTED_EDGE('',*,*,#8208,.F.);
#10853=ORIENTED_EDGE('',*,*,#8213,.T.);
#10854=ORIENTED_EDGE('',*,*,#8096,.T.);
#10855=ORIENTED_EDGE('',*,*,#8088,.F.);
#10856=ORIENTED_EDGE('',*,*,#8138,.F.);
#10857=ORIENTED_EDGE('',*,*,#8205,.F.);
#10858=ORIENTED_EDGE('',*,*,#8203,.F.);
#10859=ORIENTED_EDGE('',*,*,#8214,.F.);
#10860=ORIENTED_EDGE('',*,*,#8097,.F.);
#10861=ORIENTED_EDGE('',*,*,#8213,.F.);
#10862=ORIENTED_EDGE('',*,*,#8026,.F.);
#10863=ORIENTED_EDGE('',*,*,#8207,.F.);
#10864=ORIENTED_EDGE('',*,*,#7986,.F.);
#10865=ORIENTED_EDGE('',*,*,#8215,.F.);
#10866=ORIENTED_EDGE('',*,*,#8216,.F.);
#10867=ORIENTED_EDGE('',*,*,#8217,.F.);
#10868=ORIENTED_EDGE('',*,*,#8204,.F.);
#10869=ORIENTED_EDGE('',*,*,#8073,.F.);
#10870=ORIENTED_EDGE('',*,*,#8211,.F.);
#10871=ORIENTED_EDGE('',*,*,#8218,.F.);
#10872=ORIENTED_EDGE('',*,*,#8219,.F.);
#10873=ORIENTED_EDGE('',*,*,#8220,.F.);
#10874=ORIENTED_EDGE('',*,*,#8186,.F.);
#10875=ORIENTED_EDGE('',*,*,#8183,.F.);
#10876=ORIENTED_EDGE('',*,*,#8178,.F.);
#10877=ORIENTED_EDGE('',*,*,#8221,.F.);
#10878=ORIENTED_EDGE('',*,*,#8222,.T.);
#10879=ORIENTED_EDGE('',*,*,#8223,.T.);
#10880=ORIENTED_EDGE('',*,*,#8224,.T.);
#10881=ORIENTED_EDGE('',*,*,#8225,.T.);
#10882=ORIENTED_EDGE('',*,*,#8221,.T.);
#10883=ORIENTED_EDGE('',*,*,#8226,.T.);
#10884=ORIENTED_EDGE('',*,*,#8227,.T.);
#10885=ORIENTED_EDGE('',*,*,#8228,.T.);
#10886=ORIENTED_EDGE('',*,*,#8226,.F.);
#10887=ORIENTED_EDGE('',*,*,#8228,.F.);
#10888=ORIENTED_EDGE('',*,*,#8229,.T.);
#10889=ORIENTED_EDGE('',*,*,#8230,.T.);
#10890=ORIENTED_EDGE('',*,*,#8229,.F.);
#10891=ORIENTED_EDGE('',*,*,#8227,.F.);
#10892=ORIENTED_EDGE('',*,*,#8231,.T.);
#10893=ORIENTED_EDGE('',*,*,#8232,.T.);
#10894=ORIENTED_EDGE('',*,*,#8202,.F.);
#10895=ORIENTED_EDGE('',*,*,#8217,.T.);
#10896=ORIENTED_EDGE('',*,*,#8233,.T.);
#10897=ORIENTED_EDGE('',*,*,#8234,.T.);
#10898=ORIENTED_EDGE('',*,*,#8231,.F.);
#10899=ORIENTED_EDGE('',*,*,#8216,.T.);
#10900=ORIENTED_EDGE('',*,*,#8235,.T.);
#10901=ORIENTED_EDGE('',*,*,#8233,.F.);
#10902=ORIENTED_EDGE('',*,*,#8215,.T.);
#10903=ORIENTED_EDGE('',*,*,#8177,.F.);
#10904=ORIENTED_EDGE('',*,*,#8236,.T.);
#10905=ORIENTED_EDGE('',*,*,#8237,.T.);
#10906=ORIENTED_EDGE('',*,*,#8238,.T.);
#10907=ORIENTED_EDGE('',*,*,#7953,.T.);
#10908=ORIENTED_EDGE('',*,*,#7956,.T.);
#10909=ORIENTED_EDGE('',*,*,#8236,.F.);
#10910=ORIENTED_EDGE('',*,*,#7955,.T.);
#10911=ORIENTED_EDGE('',*,*,#8238,.F.);
#10912=ORIENTED_EDGE('',*,*,#8239,.T.);
#10913=ORIENTED_EDGE('',*,*,#8230,.F.);
#10914=ORIENTED_EDGE('',*,*,#8240,.T.);
#10915=ORIENTED_EDGE('',*,*,#8173,.T.);
#10916=ORIENTED_EDGE('',*,*,#8237,.F.);
#10917=ORIENTED_EDGE('',*,*,#8239,.F.);
#10918=ORIENTED_EDGE('',*,*,#8098,.F.);
#10919=ORIENTED_EDGE('',*,*,#8241,.T.);
#10920=ORIENTED_EDGE('',*,*,#8242,.T.);
#10921=ORIENTED_EDGE('',*,*,#8243,.T.);
#10922=ORIENTED_EDGE('',*,*,#8243,.F.);
#10923=ORIENTED_EDGE('',*,*,#8244,.F.);
#10924=ORIENTED_EDGE('',*,*,#8245,.F.);
#10925=ORIENTED_EDGE('',*,*,#8099,.F.);
#10926=ORIENTED_EDGE('',*,*,#8246,.T.);
#10927=ORIENTED_EDGE('',*,*,#8247,.T.);
#10928=ORIENTED_EDGE('',*,*,#8248,.T.);
#10929=ORIENTED_EDGE('',*,*,#8249,.T.);
#10930=ORIENTED_EDGE('',*,*,#8250,.T.);
#10931=ORIENTED_EDGE('',*,*,#8250,.F.);
#10932=ORIENTED_EDGE('',*,*,#8251,.F.);
#10933=ORIENTED_EDGE('',*,*,#8252,.F.);
#10934=ORIENTED_EDGE('',*,*,#8253,.F.);
#10935=ORIENTED_EDGE('',*,*,#8254,.F.);
#10936=ORIENTED_EDGE('',*,*,#8255,.T.);
#10937=ORIENTED_EDGE('',*,*,#8256,.T.);
#10938=ORIENTED_EDGE('',*,*,#8257,.T.);
#10939=ORIENTED_EDGE('',*,*,#8258,.T.);
#10940=ORIENTED_EDGE('',*,*,#8259,.T.);
#10941=ORIENTED_EDGE('',*,*,#8257,.F.);
#10942=ORIENTED_EDGE('',*,*,#8260,.F.);
#10943=ORIENTED_EDGE('',*,*,#8261,.F.);
#10944=ORIENTED_EDGE('',*,*,#8262,.F.);
#10945=ORIENTED_EDGE('',*,*,#8263,.T.);
#10946=ORIENTED_EDGE('',*,*,#8264,.T.);
#10947=ORIENTED_EDGE('',*,*,#8265,.T.);
#10948=ORIENTED_EDGE('',*,*,#8266,.T.);
#10949=ORIENTED_EDGE('',*,*,#8267,.T.);
#10950=ORIENTED_EDGE('',*,*,#8265,.F.);
#10951=ORIENTED_EDGE('',*,*,#8268,.F.);
#10952=ORIENTED_EDGE('',*,*,#8269,.F.);
#10953=ORIENTED_EDGE('',*,*,#8270,.F.);
#10954=ORIENTED_EDGE('',*,*,#8271,.T.);
#10955=ORIENTED_EDGE('',*,*,#8272,.T.);
#10956=ORIENTED_EDGE('',*,*,#8219,.T.);
#10957=ORIENTED_EDGE('',*,*,#8273,.T.);
#10958=ORIENTED_EDGE('',*,*,#8274,.T.);
#10959=ORIENTED_EDGE('',*,*,#8254,.T.);
#10960=ORIENTED_EDGE('',*,*,#8273,.F.);
#10961=ORIENTED_EDGE('',*,*,#8218,.T.);
#10962=ORIENTED_EDGE('',*,*,#8210,.F.);
#10963=ORIENTED_EDGE('',*,*,#8220,.T.);
#10964=ORIENTED_EDGE('',*,*,#8272,.F.);
#10965=ORIENTED_EDGE('',*,*,#8275,.T.);
#10966=ORIENTED_EDGE('',*,*,#8184,.F.);
#10967=ORIENTED_EDGE('',*,*,#8276,.F.);
#10968=ORIENTED_EDGE('',*,*,#8277,.F.);
#10969=ORIENTED_EDGE('',*,*,#8278,.T.);
#10970=ORIENTED_EDGE('',*,*,#8275,.F.);
#10971=ORIENTED_EDGE('',*,*,#8279,.T.);
#10972=ORIENTED_EDGE('',*,*,#8280,.F.);
#10973=ORIENTED_EDGE('',*,*,#8281,.F.);
#10974=ORIENTED_EDGE('',*,*,#8267,.F.);
#10975=ORIENTED_EDGE('',*,*,#8274,.F.);
#10976=ORIENTED_EDGE('',*,*,#8253,.T.);
#10977=ORIENTED_EDGE('',*,*,#8282,.F.);
#10978=ORIENTED_EDGE('',*,*,#8279,.F.);
#10979=ORIENTED_EDGE('',*,*,#8283,.T.);
#10980=ORIENTED_EDGE('',*,*,#8124,.T.);
#10981=ORIENTED_EDGE('',*,*,#8284,.T.);
#10982=ORIENTED_EDGE('',*,*,#8285,.T.);
#10983=ORIENTED_EDGE('',*,*,#8286,.T.);
#10984=ORIENTED_EDGE('',*,*,#8125,.T.);
#10985=ORIENTED_EDGE('',*,*,#8283,.F.);
#10986=ORIENTED_EDGE('',*,*,#8287,.T.);
#10987=ORIENTED_EDGE('',*,*,#8288,.T.);
#10988=ORIENTED_EDGE('',*,*,#8126,.T.);
#10989=ORIENTED_EDGE('',*,*,#8286,.F.);
#10990=ORIENTED_EDGE('',*,*,#8289,.T.);
#10991=ORIENTED_EDGE('',*,*,#8288,.F.);
#10992=ORIENTED_EDGE('',*,*,#8290,.T.);
#10993=ORIENTED_EDGE('',*,*,#8291,.T.);
#10994=ORIENTED_EDGE('',*,*,#8284,.F.);
#10995=ORIENTED_EDGE('',*,*,#8292,.T.);
#10996=ORIENTED_EDGE('',*,*,#8293,.T.);
#10997=ORIENTED_EDGE('',*,*,#8291,.F.);
#10998=ORIENTED_EDGE('',*,*,#8294,.T.);
#10999=ORIENTED_EDGE('',*,*,#8295,.T.);
#11000=ORIENTED_EDGE('',*,*,#8127,.T.);
#11001=ORIENTED_EDGE('',*,*,#8290,.F.);
#11002=ORIENTED_EDGE('',*,*,#8296,.T.);
#11003=ORIENTED_EDGE('',*,*,#8258,.F.);
#11004=ORIENTED_EDGE('',*,*,#8262,.T.);
#11005=ORIENTED_EDGE('',*,*,#8297,.T.);
#11006=ORIENTED_EDGE('',*,*,#8235,.F.);
#11007=ORIENTED_EDGE('',*,*,#8196,.T.);
#11008=ORIENTED_EDGE('',*,*,#8298,.F.);
#11009=ORIENTED_EDGE('',*,*,#8299,.F.);
#11010=ORIENTED_EDGE('',*,*,#8259,.F.);
#11011=ORIENTED_EDGE('',*,*,#8296,.F.);
#11012=ORIENTED_EDGE('',*,*,#8289,.F.);
#11013=ORIENTED_EDGE('',*,*,#8300,.F.);
#11014=ORIENTED_EDGE('',*,*,#8234,.F.);
#11015=ORIENTED_EDGE('',*,*,#8300,.T.);
#11016=ORIENTED_EDGE('',*,*,#8287,.F.);
#11017=ORIENTED_EDGE('',*,*,#8301,.F.);
#11018=ORIENTED_EDGE('',*,*,#8232,.F.);
#11019=ORIENTED_EDGE('',*,*,#8301,.T.);
#11020=ORIENTED_EDGE('',*,*,#8285,.F.);
#11021=ORIENTED_EDGE('',*,*,#8302,.F.);
#11022=ORIENTED_EDGE('',*,*,#8241,.F.);
#11023=ORIENTED_EDGE('',*,*,#8214,.T.);
#11024=ORIENTED_EDGE('',*,*,#8209,.F.);
#11025=ORIENTED_EDGE('',*,*,#8137,.T.);
#11026=ORIENTED_EDGE('',*,*,#8114,.F.);
#11027=ORIENTED_EDGE('',*,*,#8303,.T.);
#11028=ORIENTED_EDGE('',*,*,#8304,.T.);
#11029=ORIENTED_EDGE('',*,*,#8019,.F.);
#11030=ORIENTED_EDGE('',*,*,#8304,.F.);
#11031=ORIENTED_EDGE('',*,*,#8305,.F.);
#11032=ORIENTED_EDGE('',*,*,#8255,.F.);
#11033=ORIENTED_EDGE('',*,*,#8212,.F.);
#11034=ORIENTED_EDGE('',*,*,#8306,.T.);
#11035=ORIENTED_EDGE('',*,*,#8129,.T.);
#11036=ORIENTED_EDGE('',*,*,#8307,.T.);
#11037=ORIENTED_EDGE('',*,*,#8195,.T.);
#11038=ORIENTED_EDGE('',*,*,#8197,.F.);
#11039=ORIENTED_EDGE('',*,*,#8198,.T.);
#11040=ORIENTED_EDGE('',*,*,#8306,.F.);
#11041=ORIENTED_EDGE('',*,*,#8095,.F.);
#11042=ORIENTED_EDGE('',*,*,#8308,.T.);
#11043=ORIENTED_EDGE('',*,*,#8292,.F.);
#11044=ORIENTED_EDGE('',*,*,#8123,.T.);
#11045=ORIENTED_EDGE('',*,*,#8093,.F.);
#11046=ORIENTED_EDGE('',*,*,#8081,.F.);
#11047=ORIENTED_EDGE('',*,*,#8078,.F.);
#11048=ORIENTED_EDGE('',*,*,#8087,.F.);
#11049=ORIENTED_EDGE('',*,*,#8293,.F.);
#11050=ORIENTED_EDGE('',*,*,#8309,.T.);
#11051=ORIENTED_EDGE('',*,*,#8244,.T.);
#11052=ORIENTED_EDGE('',*,*,#8242,.F.);
#11053=ORIENTED_EDGE('',*,*,#8302,.T.);
#11054=ORIENTED_EDGE('',*,*,#8119,.F.);
#11055=ORIENTED_EDGE('',*,*,#8310,.T.);
#11056=ORIENTED_EDGE('',*,*,#8311,.F.);
#11057=ORIENTED_EDGE('',*,*,#8247,.F.);
#11058=ORIENTED_EDGE('',*,*,#8305,.T.);
#11059=ORIENTED_EDGE('',*,*,#8303,.F.);
#11060=ORIENTED_EDGE('',*,*,#8113,.F.);
#11061=ORIENTED_EDGE('',*,*,#8117,.F.);
#11062=ORIENTED_EDGE('',*,*,#8109,.F.);
#11063=ORIENTED_EDGE('',*,*,#8106,.F.);
#11064=ORIENTED_EDGE('',*,*,#8105,.F.);
#11065=ORIENTED_EDGE('',*,*,#8310,.F.);
#11066=ORIENTED_EDGE('',*,*,#8122,.F.);
#11067=ORIENTED_EDGE('',*,*,#8312,.F.);
#11068=ORIENTED_EDGE('',*,*,#8313,.T.);
#11069=ORIENTED_EDGE('',*,*,#8314,.F.);
#11070=ORIENTED_EDGE('',*,*,#8315,.F.);
#11071=ORIENTED_EDGE('',*,*,#8316,.F.);
#11072=ORIENTED_EDGE('',*,*,#8317,.F.);
#11073=ORIENTED_EDGE('',*,*,#8318,.F.);
#11074=ORIENTED_EDGE('',*,*,#8319,.F.);
#11075=ORIENTED_EDGE('',*,*,#8320,.F.);
#11076=ORIENTED_EDGE('',*,*,#8121,.F.);
#11077=ORIENTED_EDGE('',*,*,#8321,.F.);
#11078=ORIENTED_EDGE('',*,*,#8322,.T.);
#11079=ORIENTED_EDGE('',*,*,#8134,.T.);
#11080=ORIENTED_EDGE('',*,*,#8318,.T.);
#11081=ORIENTED_EDGE('',*,*,#8280,.T.);
#11082=ORIENTED_EDGE('',*,*,#8323,.T.);
#11083=ORIENTED_EDGE('',*,*,#8135,.T.);
#11084=ORIENTED_EDGE('',*,*,#8322,.F.);
#11085=ORIENTED_EDGE('',*,*,#8282,.T.);
#11086=ORIENTED_EDGE('',*,*,#8321,.T.);
#11087=ORIENTED_EDGE('',*,*,#8136,.T.);
#11088=ORIENTED_EDGE('',*,*,#8323,.F.);
#11089=ORIENTED_EDGE('',*,*,#8252,.T.);
#11090=ORIENTED_EDGE('',*,*,#8324,.T.);
#11091=ORIENTED_EDGE('',*,*,#8312,.T.);
#11092=ORIENTED_EDGE('',*,*,#8320,.T.);
#11093=ORIENTED_EDGE('',*,*,#8251,.T.);
#11094=ORIENTED_EDGE('',*,*,#8249,.F.);
#11095=ORIENTED_EDGE('',*,*,#8319,.T.);
#11096=ORIENTED_EDGE('',*,*,#8133,.T.);
#11097=ORIENTED_EDGE('',*,*,#8315,.T.);
#11098=ORIENTED_EDGE('',*,*,#8325,.T.);
#11099=ORIENTED_EDGE('',*,*,#8268,.T.);
#11100=ORIENTED_EDGE('',*,*,#8264,.F.);
#11101=ORIENTED_EDGE('',*,*,#8281,.T.);
#11102=ORIENTED_EDGE('',*,*,#8317,.T.);
#11103=ORIENTED_EDGE('',*,*,#8326,.T.);
#11104=ORIENTED_EDGE('',*,*,#8277,.T.);
#11105=ORIENTED_EDGE('',*,*,#8316,.T.);
#11106=ORIENTED_EDGE('',*,*,#8132,.T.);
#11107=ORIENTED_EDGE('',*,*,#8192,.F.);
#11108=ORIENTED_EDGE('',*,*,#8270,.T.);
#11109=ORIENTED_EDGE('',*,*,#8327,.T.);
#11110=ORIENTED_EDGE('',*,*,#8314,.T.);
#11111=ORIENTED_EDGE('',*,*,#8276,.T.);
#11112=ORIENTED_EDGE('',*,*,#8266,.F.);
#11113=ORIENTED_EDGE('',*,*,#8326,.F.);
#11114=ORIENTED_EDGE('',*,*,#8325,.F.);
#11115=ORIENTED_EDGE('',*,*,#8327,.F.);
#11116=ORIENTED_EDGE('',*,*,#8269,.T.);
#11117=ORIENTED_EDGE('',*,*,#8328,.F.);
#11118=ORIENTED_EDGE('',*,*,#8329,.F.);
#11119=ORIENTED_EDGE('',*,*,#8295,.F.);
#11120=ORIENTED_EDGE('',*,*,#8128,.T.);
#11121=ORIENTED_EDGE('',*,*,#8329,.T.);
#11122=ORIENTED_EDGE('',*,*,#8298,.T.);
#11123=ORIENTED_EDGE('',*,*,#8307,.F.);
#11124=ORIENTED_EDGE('',*,*,#8260,.T.);
#11125=ORIENTED_EDGE('',*,*,#8256,.F.);
#11126=ORIENTED_EDGE('',*,*,#8299,.T.);
#11127=ORIENTED_EDGE('',*,*,#8328,.T.);
#11128=ORIENTED_EDGE('',*,*,#8330,.T.);
#11129=ORIENTED_EDGE('',*,*,#8263,.F.);
#11130=ORIENTED_EDGE('',*,*,#8331,.T.);
#11131=ORIENTED_EDGE('',*,*,#8225,.F.);
#11132=ORIENTED_EDGE('',*,*,#8331,.F.);
#11133=ORIENTED_EDGE('',*,*,#8332,.F.);
#11134=ORIENTED_EDGE('',*,*,#8333,.T.);
#11135=ORIENTED_EDGE('',*,*,#8224,.F.);
#11136=ORIENTED_EDGE('',*,*,#8333,.F.);
#11137=ORIENTED_EDGE('',*,*,#8271,.F.);
#11138=ORIENTED_EDGE('',*,*,#8334,.T.);
#11139=ORIENTED_EDGE('',*,*,#8223,.F.);
#11140=ORIENTED_EDGE('',*,*,#8334,.F.);
#11141=ORIENTED_EDGE('',*,*,#8246,.F.);
#11142=ORIENTED_EDGE('',*,*,#8335,.T.);
#11143=ORIENTED_EDGE('',*,*,#8222,.F.);
#11144=ORIENTED_EDGE('',*,*,#8335,.F.);
#11145=ORIENTED_EDGE('',*,*,#8297,.F.);
#11146=ORIENTED_EDGE('',*,*,#8261,.T.);
#11147=ORIENTED_EDGE('',*,*,#8330,.F.);
#11148=ORIENTED_EDGE('',*,*,#8294,.F.);
#11149=ORIENTED_EDGE('',*,*,#8248,.F.);
#11150=ORIENTED_EDGE('',*,*,#8311,.T.);
#11151=ORIENTED_EDGE('',*,*,#8313,.F.);
#11152=ORIENTED_EDGE('',*,*,#8324,.F.);
#11153=ORIENTED_EDGE('',*,*,#8332,.T.);
#11154=ORIENTED_EDGE('',*,*,#8100,.F.);
#11155=ORIENTED_EDGE('',*,*,#8245,.T.);
#11156=ORIENTED_EDGE('',*,*,#8309,.F.);
#11157=ORIENTED_EDGE('',*,*,#8308,.F.);
#11158=ORIENTED_EDGE('',*,*,#8022,.F.);
#11159=ORIENTED_EDGE('',*,*,#8045,.F.);
#11160=ORIENTED_EDGE('',*,*,#7991,.F.);
#11161=ORIENTED_EDGE('',*,*,#8076,.F.);
#11162=ORIENTED_EDGE('',*,*,#7954,.F.);
#11163=ORIENTED_EDGE('',*,*,#8151,.F.);
#11164=ORIENTED_EDGE('',*,*,#8155,.F.);
#11165=ORIENTED_EDGE('',*,*,#8159,.F.);
#11166=ORIENTED_EDGE('',*,*,#8163,.F.);
#11167=ORIENTED_EDGE('',*,*,#8168,.F.);
#11168=ORIENTED_EDGE('',*,*,#8240,.F.);
#11169=ORIENTED_EDGE('',*,*,#8336,.T.);
#11170=ORIENTED_EDGE('',*,*,#8337,.T.);
#11171=ORIENTED_EDGE('',*,*,#8336,.F.);
#11172=ORIENTED_EDGE('',*,*,#8337,.F.);
#11173=ORIENTED_EDGE('',*,*,#8338,.T.);
#11174=ORIENTED_EDGE('',*,*,#8338,.F.);
#11175=ORIENTED_EDGE('',*,*,#8339,.T.);
#11176=ORIENTED_EDGE('',*,*,#7938,.T.);
#11177=ORIENTED_EDGE('',*,*,#8339,.F.);
#11178=ORIENTED_EDGE('',*,*,#7940,.F.);
#11179=ORIENTED_EDGE('',*,*,#8185,.F.);
#11180=ORIENTED_EDGE('',*,*,#8278,.F.);
#11181=ORIENTED_EDGE('',*,*,#8191,.F.);
#11182=ORIENTED_EDGE('',*,*,#8188,.F.);
#14116=CONICAL_SURFACE('',#15495,13.25,0.785398163397442);
#14117=CONICAL_SURFACE('',#15503,19.25,0.785398163397457);
#14118=CONICAL_SURFACE('',#15513,6.3,0.785398163397435);
#14119=CONICAL_SURFACE('',#15516,6.3,0.785398163397435);
#14120=CONICAL_SURFACE('',#15525,6.3,0.785398163397442);
#14121=CONICAL_SURFACE('',#15527,6.3,0.785398163397442);
#14122=CONICAL_SURFACE('',#15536,6.3,0.785398163397435);
#14123=CONICAL_SURFACE('',#15539,6.3,0.785398163397438);
#14124=CONICAL_SURFACE('',#15544,6.3,0.785398163397442);
#14125=CONICAL_SURFACE('',#15546,6.3,0.785398163397442);
#14126=CONICAL_SURFACE('',#15555,1.75,0.785398163397441);
#14127=CONICAL_SURFACE('',#15560,1.75,0.785398163397441);
#14128=CONICAL_SURFACE('',#15577,5.30000000000001,0.785398163397457);
#14129=CONICAL_SURFACE('',#15587,5.29999999999999,0.785398163397457);
#14130=CONICAL_SURFACE('',#15591,5.29999999999999,0.785398163397457);
#14131=CONICAL_SURFACE('',#15595,5.30000000000001,0.785398163397457);
#14132=CONICAL_SURFACE('',#15599,9.75,0.785398163397457);
#14304=ADVANCED_FACE('',(#1737),#14116,.F.);
#14305=ADVANCED_FACE('',(#1738,#435),#594,.F.);
#14306=ADVANCED_FACE('',(#1739),#1409,.F.);
#14307=ADVANCED_FACE('',(#1740),#14117,.F.);
#14308=ADVANCED_FACE('',(#1741,#436),#595,.T.);
#14309=ADVANCED_FACE('',(#1742),#1410,.F.);
#14310=ADVANCED_FACE('',(#1743),#14118,.F.);
#14311=ADVANCED_FACE('',(#1744),#215,.T.);
#14312=ADVANCED_FACE('',(#1745),#216,.T.);
#14313=ADVANCED_FACE('',(#1746),#14119,.F.);
#14314=ADVANCED_FACE('',(#1747),#217,.T.);
#14315=ADVANCED_FACE('',(#1748),#218,.T.);
#14316=ADVANCED_FACE('',(#1749),#219,.T.);
#14317=ADVANCED_FACE('',(#1750),#220,.T.);
#14318=ADVANCED_FACE('',(#1751),#596,.T.);
#14319=ADVANCED_FACE('',(#1752),#1411,.T.);
#14320=ADVANCED_FACE('',(#1753),#1412,.F.);
#14321=ADVANCED_FACE('',(#1754),#14120,.F.);
#14322=ADVANCED_FACE('',(#1755),#221,.T.);
#14323=ADVANCED_FACE('',(#1756),#222,.T.);
#14324=ADVANCED_FACE('',(#1757),#14121,.F.);
#14325=ADVANCED_FACE('',(#1758),#223,.T.);
#14326=ADVANCED_FACE('',(#1759),#224,.T.);
#14327=ADVANCED_FACE('',(#1760),#225,.T.);
#14328=ADVANCED_FACE('',(#1761),#226,.T.);
#14329=ADVANCED_FACE('',(#1762),#597,.T.);
#14330=ADVANCED_FACE('',(#1763),#1413,.T.);
#14331=ADVANCED_FACE('',(#1764),#1414,.F.);
#14332=ADVANCED_FACE('',(#1765),#14122,.F.);
#14333=ADVANCED_FACE('',(#1766),#227,.T.);
#14334=ADVANCED_FACE('',(#1767),#228,.T.);
#14335=ADVANCED_FACE('',(#1768),#14123,.F.);
#14336=ADVANCED_FACE('',(#1769),#229,.T.);
#14337=ADVANCED_FACE('',(#1770),#230,.T.);
#14338=ADVANCED_FACE('',(#1771),#231,.T.);
#14339=ADVANCED_FACE('',(#1772),#232,.T.);
#14340=ADVANCED_FACE('',(#1773),#1415,.F.);
#14341=ADVANCED_FACE('',(#1774),#14124,.F.);
#14342=ADVANCED_FACE('',(#1775),#233,.T.);
#14343=ADVANCED_FACE('',(#1776),#234,.T.);
#14344=ADVANCED_FACE('',(#1777),#14125,.F.);
#14345=ADVANCED_FACE('',(#1778),#235,.T.);
#14346=ADVANCED_FACE('',(#1779),#236,.T.);
#14347=ADVANCED_FACE('',(#1780),#237,.T.);
#14348=ADVANCED_FACE('',(#1781),#238,.T.);
#14349=ADVANCED_FACE('',(#1782),#598,.T.);
#14350=ADVANCED_FACE('',(#1783),#1416,.T.);
#14351=ADVANCED_FACE('',(#1784),#1417,.F.);
#14352=ADVANCED_FACE('',(#1785),#239,.T.);
#14353=ADVANCED_FACE('',(#1786),#240,.T.);
#14354=ADVANCED_FACE('',(#1787),#241,.T.);
#14355=ADVANCED_FACE('',(#1788),#14126,.T.);
#14356=ADVANCED_FACE('',(#1789),#242,.T.);
#14357=ADVANCED_FACE('',(#1790),#243,.F.);
#14358=ADVANCED_FACE('',(#1791),#1418,.T.);
#14359=ADVANCED_FACE('',(#1792),#244,.T.);
#14360=ADVANCED_FACE('',(#1793),#245,.T.);
#14361=ADVANCED_FACE('',(#1794),#246,.T.);
#14362=ADVANCED_FACE('',(#1795),#14127,.T.);
#14363=ADVANCED_FACE('',(#1796),#247,.T.);
#14364=ADVANCED_FACE('',(#1797),#248,.F.);
#14365=ADVANCED_FACE('',(#1798),#274,.T.);
#14366=ADVANCED_FACE('',(#1799),#599,.T.);
#14367=ADVANCED_FACE('',(#1800),#14128,.F.);
#14368=ADVANCED_FACE('',(#1801,#437,#438,#439,#440,#441),#600,.T.);
#14369=ADVANCED_FACE('',(#1802),#1419,.F.);
#14370=ADVANCED_FACE('',(#1803),#14129,.F.);
#14371=ADVANCED_FACE('',(#1804),#1420,.F.);
#14372=ADVANCED_FACE('',(#1805),#14130,.F.);
#14373=ADVANCED_FACE('',(#1806),#1421,.F.);
#14374=ADVANCED_FACE('',(#1807),#14131,.F.);
#14375=ADVANCED_FACE('',(#1808),#1422,.F.);
#14376=ADVANCED_FACE('',(#1809),#14132,.F.);
#14377=ADVANCED_FACE('',(#1810),#1423,.F.);
#14378=ADVANCED_FACE('',(#1811),#249,.F.);
#14379=ADVANCED_FACE('',(#1812),#1424,.F.);
#14380=ADVANCED_FACE('',(#1813),#1425,.T.);
#14381=ADVANCED_FACE('',(#1814),#132,.T.);
#14382=ADVANCED_FACE('',(#1815),#1426,.T.);
#14383=ADVANCED_FACE('',(#1816),#1427,.T.);
#14384=ADVANCED_FACE('',(#1817),#1428,.T.);
#14385=ADVANCED_FACE('',(#1818),#133,.T.);
#14386=ADVANCED_FACE('',(#1819),#1429,.T.);
#14387=ADVANCED_FACE('',(#1820),#134,.T.);
#14388=ADVANCED_FACE('',(#1821),#601,.F.);
#14389=ADVANCED_FACE('',(#1822),#1430,.T.);
#14390=ADVANCED_FACE('',(#1823),#1431,.T.);
#14391=ADVANCED_FACE('',(#1824),#135,.T.);
#14392=ADVANCED_FACE('',(#1825),#136,.T.);
#14393=ADVANCED_FACE('',(#1826),#1432,.T.);
#14394=ADVANCED_FACE('',(#1827),#1433,.T.);
#14395=ADVANCED_FACE('',(#1828),#137,.T.);
#14396=ADVANCED_FACE('',(#1829),#138,.T.);
#14397=ADVANCED_FACE('',(#1830),#1434,.T.);
#14398=ADVANCED_FACE('',(#1831),#1435,.T.);
#14399=ADVANCED_FACE('',(#1832),#602,.F.);
#14400=ADVANCED_FACE('',(#1833),#603,.T.);
#14401=ADVANCED_FACE('',(#1834,#442,#443,#444,#445,#446),#604,.F.);
#14402=ADVANCED_FACE('',(#1835),#275,.T.);
#14403=ADVANCED_FACE('',(#1836),#1436,.F.);
#14404=ADVANCED_FACE('',(#1837),#276,.T.);
#14405=ADVANCED_FACE('',(#1838),#1437,.T.);
#14406=ADVANCED_FACE('',(#1839),#277,.T.);
#14407=ADVANCED_FACE('',(#1840),#250,.F.);
#14408=ADVANCED_FACE('',(#1841),#251,.F.);
#14409=ADVANCED_FACE('',(#1842,#447,#448,#449),#605,.F.);
#14410=ADVANCED_FACE('',(#1843),#278,.T.);
#14411=ADVANCED_FACE('',(#1844,#450),#606,.T.);
#14412=ADVANCED_FACE('',(#1845),#279,.T.);
#14413=ADVANCED_FACE('',(#1846),#1438,.T.);
#14414=ADVANCED_FACE('',(#1847),#280,.T.);
#14415=ADVANCED_FACE('',(#1848,#451),#607,.T.);
#14416=ADVANCED_FACE('',(#1849),#281,.T.);
#14417=ADVANCED_FACE('',(#1850,#452),#608,.T.);
#14418=ADVANCED_FACE('',(#1851),#1439,.T.);
#14419=ADVANCED_FACE('',(#1852),#282,.T.);
#14420=ADVANCED_FACE('',(#1853),#283,.T.);
#14421=ADVANCED_FACE('',(#1854),#1440,.T.);
#14422=ADVANCED_FACE('',(#1855),#609,.T.);
#14423=ADVANCED_FACE('',(#1856),#284,.T.);
#14424=ADVANCED_FACE('',(#1857),#1441,.T.);
#14425=ADVANCED_FACE('',(#1858),#285,.T.);
#14426=ADVANCED_FACE('',(#1859),#139,.T.);
#14427=ADVANCED_FACE('',(#1860),#140,.T.);
#14428=ADVANCED_FACE('',(#1861),#286,.T.);
#14429=ADVANCED_FACE('',(#1862),#1442,.T.);
#14430=ADVANCED_FACE('',(#1863),#1443,.T.);
#14431=ADVANCED_FACE('',(#1864),#610,.T.);
#14432=ADVANCED_FACE('',(#1865),#1444,.T.);
#14433=ADVANCED_FACE('',(#1866),#1445,.T.);
#14434=ADVANCED_FACE('',(#1867),#611,.T.);
#14435=ADVANCED_FACE('',(#1868),#1446,.T.);
#14436=ADVANCED_FACE('',(#1869),#141,.T.);
#14437=ADVANCED_FACE('',(#1870),#287,.T.);
#14438=ADVANCED_FACE('',(#1871),#1447,.T.);
#14439=ADVANCED_FACE('',(#1872),#1448,.T.);
#14440=ADVANCED_FACE('',(#1873),#1449,.F.);
#14441=ADVANCED_FACE('',(#1874),#142,.T.);
#14442=ADVANCED_FACE('',(#1875),#143,.T.);
#14443=ADVANCED_FACE('',(#1876),#144,.T.);
#14444=ADVANCED_FACE('',(#1877),#288,.T.);
#14445=ADVANCED_FACE('',(#1878),#1450,.T.);
#14446=ADVANCED_FACE('',(#1879),#289,.T.);
#14447=ADVANCED_FACE('',(#1880),#1451,.T.);
#14448=ADVANCED_FACE('',(#1881),#290,.T.);
#14449=ADVANCED_FACE('',(#1882),#1452,.T.);
#14450=ADVANCED_FACE('',(#1883),#291,.T.);
#14451=ADVANCED_FACE('',(#1884),#1453,.T.);
#14452=ADVANCED_FACE('',(#1885),#1454,.F.);
#14453=ADVANCED_FACE('',(#1886),#145,.T.);
#14454=ADVANCED_FACE('',(#1887),#292,.T.);
#14455=ADVANCED_FACE('',(#1888),#1455,.T.);
#14456=ADVANCED_FACE('',(#1889),#1456,.F.);
#14457=ADVANCED_FACE('',(#1890),#1457,.F.);
#14458=ADVANCED_FACE('',(#1891),#1458,.F.);
#14459=ADVANCED_FACE('',(#1892),#1459,.F.);
#14460=ADVANCED_FACE('',(#1893),#1460,.F.);
#14461=ADVANCED_FACE('',(#1894,#453),#612,.T.);
#14462=ADVANCED_FACE('',(#1895),#1461,.F.);
#14463=ADVANCED_FACE('',(#1896),#613,.F.);
#14464=ADVANCED_FACE('',(#1897),#614,.F.);
#14465=ADVANCED_FACE('',(#1898),#615,.F.);
#14466=ADVANCED_FACE('',(#1899),#616,.F.);
#14467=ADVANCED_FACE('',(#1900),#617,.F.);
#14468=ADVANCED_FACE('',(#1901),#618,.T.);
#14469=ADVANCED_FACE('',(#1902),#619,.T.);
#14470=ADVANCED_FACE('',(#1903),#620,.T.);
#14471=ADVANCED_FACE('',(#1904),#621,.T.);
#14472=ADVANCED_FACE('',(#1905),#622,.T.);
#14473=ADVANCED_FACE('',(#1906),#1462,.F.);
#14474=ADVANCED_FACE('',(#1907,#454),#623,.F.);
#14475=ADVANCED_FACE('',(#1908),#1463,.F.);
#14476=ADVANCED_FACE('',(#1909),#624,.F.);
#14477=ADVANCED_FACE('',(#1910),#625,.T.);
#15072=CLOSED_SHELL('',(#14304,#14305,#14306,#14307,#14308,#14309,#14310,
#14311,#14312,#14313,#14314,#14315,#14316,#14317,#14318,#14319,#14320,#14321,
#14322,#14323,#14324,#14325,#14326,#14327,#14328,#14329,#14330,#14331,#14332,
#14333,#14334,#14335,#14336,#14337,#14338,#14339,#14340,#14341,#14342,#14343,
#14344,#14345,#14346,#14347,#14348,#14349,#14350,#14351,#14352,#14353,#14354,
#14355,#14356,#14357,#14358,#14359,#14360,#14361,#14362,#14363,#14364,#14365,
#14366,#14367,#14368,#14369,#14370,#14371,#14372,#14373,#14374,#14375,#14376,
#14377,#14378,#14379,#14380,#14381,#14382,#14383,#14384,#14385,#14386,#14387,
#14388,#14389,#14390,#14391,#14392,#14393,#14394,#14395,#14396,#14397,#14398,
#14399,#14400,#14401,#14402,#14403,#14404,#14405,#14406,#14407,#14408,#14409,
#14410,#14411,#14412,#14413,#14414,#14415,#14416,#14417,#14418,#14419,#14420,
#14421,#14422,#14423,#14424,#14425,#14426,#14427,#14428,#14429,#14430,#14431,
#14432,#14433,#14434,#14435,#14436,#14437,#14438,#14439,#14440,#14441,#14442,
#14443,#14444,#14445,#14446,#14447,#14448,#14449,#14450,#14451,#14452,#14453,
#14454,#14455,#14456,#14457,#14458,#14459,#14460,#14461,#14462,#14463,#14464,
#14465,#14466,#14467,#14468,#14469,#14470,#14471,#14472,#14473,#14474,#14475,
#14476,#14477));
#15494=AXIS2_PLACEMENT_3D('',#22626,#17363,#17364);
#15495=AXIS2_PLACEMENT_3D('',#22627,#17365,#17366);
#15496=AXIS2_PLACEMENT_3D('',#22629,#17367,#17368);
#15497=AXIS2_PLACEMENT_3D('',#22633,#17370,#17371);
#15498=AXIS2_PLACEMENT_3D('',#22634,#17372,#17373);
#15499=AXIS2_PLACEMENT_3D('',#22635,#17374,#17375);
#15500=AXIS2_PLACEMENT_3D('',#22637,#17376,#17377);
#15501=AXIS2_PLACEMENT_3D('',#22638,#17378,#17379);
#15502=AXIS2_PLACEMENT_3D('',#22641,#17381,#17382);
#15503=AXIS2_PLACEMENT_3D('',#22642,#17383,#17384);
#15504=AXIS2_PLACEMENT_3D('',#22644,#17385,#17386);
#15505=AXIS2_PLACEMENT_3D('',#22647,#17388,#17389);
#15506=AXIS2_PLACEMENT_3D('',#22648,#17390,#17391);
#15507=AXIS2_PLACEMENT_3D('',#22651,#17392,#17393);
#15508=AXIS2_PLACEMENT_3D('',#22655,#17395,#17396);
#15509=AXIS2_PLACEMENT_3D('',#22659,#17398,#17399);
#15510=AXIS2_PLACEMENT_3D('',#22663,#17401,#17402);
#15511=AXIS2_PLACEMENT_3D('',#22665,#17404,#17405);
#15512=AXIS2_PLACEMENT_3D('',#22703,#17407,#17408);
#15513=AXIS2_PLACEMENT_3D('',#22737,#17409,#17410);
#15514=AXIS2_PLACEMENT_3D('',#22741,#17412,#17413);
#15515=AXIS2_PLACEMENT_3D('',#22743,#17414,#17415);
#15516=AXIS2_PLACEMENT_3D('',#22847,#17419,#17420);
#15517=AXIS2_PLACEMENT_3D('',#22852,#17422,#17423);
#15518=AXIS2_PLACEMENT_3D('',#22855,#17425,#17426);
#15519=AXIS2_PLACEMENT_3D('',#22982,#17429,#17430);
#15520=AXIS2_PLACEMENT_3D('',#22986,#17433,#17434);
#15521=AXIS2_PLACEMENT_3D('',#23007,#17436,#17437);
#15522=AXIS2_PLACEMENT_3D('',#23010,#17439,#17440);
#15523=AXIS2_PLACEMENT_3D('',#23011,#17441,#17442);
#15524=AXIS2_PLACEMENT_3D('',#23014,#17444,#17445);
#15525=AXIS2_PLACEMENT_3D('',#23015,#17446,#17447);
#15526=AXIS2_PLACEMENT_3D('',#23019,#17449,#17450);
#15527=AXIS2_PLACEMENT_3D('',#23128,#17454,#17455);
#15528=AXIS2_PLACEMENT_3D('',#23133,#17457,#17458);
#15529=AXIS2_PLACEMENT_3D('',#23136,#17460,#17461);
#15530=AXIS2_PLACEMENT_3D('',#23263,#17464,#17465);
#15531=AXIS2_PLACEMENT_3D('',#23267,#17468,#17469);
#15532=AXIS2_PLACEMENT_3D('',#23269,#17470,#17471);
#15533=AXIS2_PLACEMENT_3D('',#23272,#17473,#17474);
#15534=AXIS2_PLACEMENT_3D('',#23273,#17475,#17476);
#15535=AXIS2_PLACEMENT_3D('',#23276,#17478,#17479);
#15536=AXIS2_PLACEMENT_3D('',#23277,#17480,#17481);
#15537=AXIS2_PLACEMENT_3D('',#23281,#17483,#17484);
#15538=AXIS2_PLACEMENT_3D('',#23284,#17486,#17487);
#15539=AXIS2_PLACEMENT_3D('',#23375,#17490,#17491);
#15540=AXIS2_PLACEMENT_3D('',#23379,#17493,#17494);
#15541=AXIS2_PLACEMENT_3D('',#23381,#17495,#17496);
#15542=AXIS2_PLACEMENT_3D('',#23481,#17500,#17501);
#15543=AXIS2_PLACEMENT_3D('',#23484,#17503,#17504);
#15544=AXIS2_PLACEMENT_3D('',#23485,#17505,#17506);
#15545=AXIS2_PLACEMENT_3D('',#23489,#17508,#17509);
#15546=AXIS2_PLACEMENT_3D('',#23557,#17513,#17514);
#15547=AXIS2_PLACEMENT_3D('',#23562,#17516,#17517);
#15548=AXIS2_PLACEMENT_3D('',#23565,#17519,#17520);
#15549=AXIS2_PLACEMENT_3D('',#23727,#17523,#17524);
#15550=AXIS2_PLACEMENT_3D('',#23731,#17527,#17528);
#15551=AXIS2_PLACEMENT_3D('',#23733,#17529,#17530);
#15552=AXIS2_PLACEMENT_3D('',#23736,#17532,#17533);
#15553=AXIS2_PLACEMENT_3D('',#23737,#17534,#17535);
#15554=AXIS2_PLACEMENT_3D('',#23740,#17537,#17538);
#15555=AXIS2_PLACEMENT_3D('',#23878,#17540,#17541);
#15556=AXIS2_PLACEMENT_3D('',#23894,#17542,#17543);
#15557=AXIS2_PLACEMENT_3D('',#23897,#17545,#17546);
#15558=AXIS2_PLACEMENT_3D('',#23947,#17547,#17548);
#15559=AXIS2_PLACEMENT_3D('',#23979,#17550,#17551);
#15560=AXIS2_PLACEMENT_3D('',#24137,#17554,#17555);
#15561=AXIS2_PLACEMENT_3D('',#24142,#17557,#17558);
#15562=AXIS2_PLACEMENT_3D('',#24156,#17559,#17560);
#15563=AXIS2_PLACEMENT_3D('',#24206,#17561,#17562);
#15564=AXIS2_PLACEMENT_3D('',#24208,#17563,#17564);
#15565=AXIS2_PLACEMENT_3D('',#24210,#17565,#17566);
#15566=AXIS2_PLACEMENT_3D('',#24211,#17567,#17568);
#15567=AXIS2_PLACEMENT_3D('',#24212,#17569,#17570);
#15568=AXIS2_PLACEMENT_3D('',#24214,#17571,#17572);
#15569=AXIS2_PLACEMENT_3D('',#24216,#17573,#17574);
#15570=AXIS2_PLACEMENT_3D('',#24220,#17576,#17577);
#15571=AXIS2_PLACEMENT_3D('',#24222,#17578,#17579);
#15572=AXIS2_PLACEMENT_3D('',#24224,#17580,#17581);
#15573=AXIS2_PLACEMENT_3D('',#24232,#17585,#17586);
#15574=AXIS2_PLACEMENT_3D('',#24234,#17587,#17588);
#15575=AXIS2_PLACEMENT_3D('',#24236,#17589,#17590);
#15576=AXIS2_PLACEMENT_3D('',#24239,#17592,#17593);
#15577=AXIS2_PLACEMENT_3D('',#24242,#17596,#17597);
#15578=AXIS2_PLACEMENT_3D('',#24244,#17598,#17599);
#15579=AXIS2_PLACEMENT_3D('',#24247,#17601,#17602);
#15580=AXIS2_PLACEMENT_3D('',#24248,#17603,#17604);
#15581=AXIS2_PLACEMENT_3D('',#24258,#17609,#17610);
#15582=AXIS2_PLACEMENT_3D('',#24260,#17611,#17612);
#15583=AXIS2_PLACEMENT_3D('',#24262,#17613,#17614);
#15584=AXIS2_PLACEMENT_3D('',#24264,#17615,#17616);
#15585=AXIS2_PLACEMENT_3D('',#24265,#17617,#17618);
#15586=AXIS2_PLACEMENT_3D('',#24268,#17620,#17621);
#15587=AXIS2_PLACEMENT_3D('',#24269,#17622,#17623);
#15588=AXIS2_PLACEMENT_3D('',#24272,#17625,#17626);
#15589=AXIS2_PLACEMENT_3D('',#24273,#17627,#17628);
#15590=AXIS2_PLACEMENT_3D('',#24276,#17630,#17631);
#15591=AXIS2_PLACEMENT_3D('',#24277,#17632,#17633);
#15592=AXIS2_PLACEMENT_3D('',#24280,#17635,#17636);
#15593=AXIS2_PLACEMENT_3D('',#24281,#17637,#17638);
#15594=AXIS2_PLACEMENT_3D('',#24284,#17640,#17641);
#15595=AXIS2_PLACEMENT_3D('',#24285,#17642,#17643);
#15596=AXIS2_PLACEMENT_3D('',#24288,#17645,#17646);
#15597=AXIS2_PLACEMENT_3D('',#24289,#17647,#17648);
#15598=AXIS2_PLACEMENT_3D('',#24292,#17650,#17651);
#15599=AXIS2_PLACEMENT_3D('',#24293,#17652,#17653);
#15600=AXIS2_PLACEMENT_3D('',#24296,#17655,#17656);
#15601=AXIS2_PLACEMENT_3D('',#24297,#17657,#17658);
#15602=AXIS2_PLACEMENT_3D('',#24315,#17660,#17661);
#15603=AXIS2_PLACEMENT_3D('',#24444,#17662,#17663);
#15604=AXIS2_PLACEMENT_3D('',#24467,#17664,#17665);
#15605=AXIS2_PLACEMENT_3D('',#24469,#17666,#17667);
#15606=AXIS2_PLACEMENT_3D('',#24471,#17669,#17670);
#15607=AXIS2_PLACEMENT_3D('',#24474,#17671,#17672);
#15608=AXIS2_PLACEMENT_3D('',#24493,#17675,#17676);
#15609=AXIS2_PLACEMENT_3D('',#24495,#17677,#17678);
#15610=AXIS2_PLACEMENT_3D('',#24497,#17679,#17680);
#15611=AXIS2_PLACEMENT_3D('',#24498,#17681,#17682);
#15612=AXIS2_PLACEMENT_3D('',#24499,#17683,#17684);
#15613=AXIS2_PLACEMENT_3D('',#24500,#17685,#17686);
#15614=AXIS2_PLACEMENT_3D('',#24502,#17688,#17689);
#15615=AXIS2_PLACEMENT_3D('',#24521,#17692,#17693);
#15616=AXIS2_PLACEMENT_3D('',#24523,#17694,#17695);
#15617=AXIS2_PLACEMENT_3D('',#24525,#17697,#17698);
#15618=AXIS2_PLACEMENT_3D('',#24526,#17699,#17700);
#15619=AXIS2_PLACEMENT_3D('',#24527,#17701,#17702);
#15620=AXIS2_PLACEMENT_3D('',#24528,#17703,#17704);
#15621=AXIS2_PLACEMENT_3D('',#24545,#17706,#17707);
#15622=AXIS2_PLACEMENT_3D('',#24546,#17708,#17709);
#15623=AXIS2_PLACEMENT_3D('',#24547,#17710,#17711);
#15624=AXIS2_PLACEMENT_3D('',#24553,#17715,#17716);
#15625=AXIS2_PLACEMENT_3D('',#24554,#17717,#17718);
#15626=AXIS2_PLACEMENT_3D('',#24555,#17719,#17720);
#15627=AXIS2_PLACEMENT_3D('',#24556,#17721,#17722);
#15628=AXIS2_PLACEMENT_3D('',#24557,#17723,#17724);
#15629=AXIS2_PLACEMENT_3D('',#24558,#17725,#17726);
#15630=AXIS2_PLACEMENT_3D('',#24559,#17727,#17728);
#15631=AXIS2_PLACEMENT_3D('',#24561,#17729,#17730);
#15632=AXIS2_PLACEMENT_3D('',#24562,#17731,#17732);
#15633=AXIS2_PLACEMENT_3D('',#24563,#17733,#17734);
#15634=AXIS2_PLACEMENT_3D('',#24582,#17737,#17738);
#15635=AXIS2_PLACEMENT_3D('',#24585,#17740,#17741);
#15636=AXIS2_PLACEMENT_3D('',#24587,#17743,#17744);
#15637=AXIS2_PLACEMENT_3D('',#24588,#17745,#17746);
#15638=AXIS2_PLACEMENT_3D('',#24589,#17747,#17748);
#15639=AXIS2_PLACEMENT_3D('',#24590,#17749,#17750);
#15640=AXIS2_PLACEMENT_3D('',#24591,#17751,#17752);
#15641=AXIS2_PLACEMENT_3D('',#24610,#17755,#17756);
#15642=AXIS2_PLACEMENT_3D('',#24612,#17758,#17759);
#15643=AXIS2_PLACEMENT_3D('',#24614,#17761,#17762);
#15644=AXIS2_PLACEMENT_3D('',#24615,#17763,#17764);
#15645=AXIS2_PLACEMENT_3D('',#24617,#17765,#17766);
#15646=AXIS2_PLACEMENT_3D('',#24620,#17768,#17769);
#15647=AXIS2_PLACEMENT_3D('',#24622,#17770,#17771);
#15648=AXIS2_PLACEMENT_3D('',#24625,#17773,#17774);
#15649=AXIS2_PLACEMENT_3D('',#24627,#17775,#17776);
#15650=AXIS2_PLACEMENT_3D('',#24629,#17777,#17778);
#15651=AXIS2_PLACEMENT_3D('',#24631,#17779,#17780);
#15652=AXIS2_PLACEMENT_3D('',#24633,#17781,#17782);
#15653=AXIS2_PLACEMENT_3D('',#24635,#17783,#17784);
#15654=AXIS2_PLACEMENT_3D('',#24636,#17785,#17786);
#15655=AXIS2_PLACEMENT_3D('',#24638,#17787,#17788);
#15656=AXIS2_PLACEMENT_3D('',#24640,#17789,#17790);
#15657=AXIS2_PLACEMENT_3D('',#24641,#17791,#17792);
#15658=AXIS2_PLACEMENT_3D('',#24642,#17793,#17794);
#15659=AXIS2_PLACEMENT_3D('',#24645,#17796,#17797);
#15660=AXIS2_PLACEMENT_3D('',#24646,#17798,#17799);
#15661=AXIS2_PLACEMENT_3D('',#24648,#17800,#17801);
#15662=AXIS2_PLACEMENT_3D('',#24649,#17802,#17803);
#15663=AXIS2_PLACEMENT_3D('',#24650,#17804,#17805);
#15664=AXIS2_PLACEMENT_3D('',#24652,#17806,#17807);
#15665=AXIS2_PLACEMENT_3D('',#24654,#17809,#17810);
#15666=AXIS2_PLACEMENT_3D('',#24655,#17811,#17812);
#15667=AXIS2_PLACEMENT_3D('',#24765,#17813,#17814);
#15668=AXIS2_PLACEMENT_3D('',#25020,#17815,#17816);
#15669=AXIS2_PLACEMENT_3D('',#25077,#17817,#17818);
#15670=AXIS2_PLACEMENT_3D('',#25079,#17819,#17820);
#15671=AXIS2_PLACEMENT_3D('',#25080,#17821,#17822);
#15672=AXIS2_PLACEMENT_3D('',#25082,#17823,#17824);
#15673=AXIS2_PLACEMENT_3D('',#25098,#17825,#17826);
#15674=AXIS2_PLACEMENT_3D('',#25099,#17827,#17828);
#15675=AXIS2_PLACEMENT_3D('',#25101,#17829,#17830);
#15676=AXIS2_PLACEMENT_3D('',#25102,#17831,#17832);
#15677=AXIS2_PLACEMENT_3D('',#25104,#17833,#17834);
#15678=AXIS2_PLACEMENT_3D('',#25105,#17835,#17836);
#15679=AXIS2_PLACEMENT_3D('',#25129,#17837,#17838);
#15680=AXIS2_PLACEMENT_3D('',#25145,#17839,#17840);
#15681=AXIS2_PLACEMENT_3D('',#25146,#17841,#17842);
#15682=AXIS2_PLACEMENT_3D('',#25150,#17844,#17845);
#15683=AXIS2_PLACEMENT_3D('',#25153,#17847,#17848);
#15684=AXIS2_PLACEMENT_3D('',#25155,#17850,#17851);
#15685=AXIS2_PLACEMENT_3D('',#25173,#17852,#17853);
#15686=AXIS2_PLACEMENT_3D('',#25189,#17854,#17855);
#15687=AXIS2_PLACEMENT_3D('',#25190,#17856,#17857);
#15688=AXIS2_PLACEMENT_3D('',#25192,#17858,#17859);
#15689=AXIS2_PLACEMENT_3D('',#25194,#17860,#17861);
#15690=AXIS2_PLACEMENT_3D('',#25195,#17862,#17863);
#15691=AXIS2_PLACEMENT_3D('',#25197,#17864,#17865);
#15692=AXIS2_PLACEMENT_3D('',#25198,#17866,#17867);
#15693=AXIS2_PLACEMENT_3D('',#25216,#17868,#17869);
#15694=AXIS2_PLACEMENT_3D('',#25232,#17870,#17871);
#15695=AXIS2_PLACEMENT_3D('',#25233,#17872,#17873);
#15696=AXIS2_PLACEMENT_3D('',#25235,#17874,#17875);
#15697=AXIS2_PLACEMENT_3D('',#25237,#17876,#17877);
#15698=AXIS2_PLACEMENT_3D('',#25238,#17878,#17879);
#15699=AXIS2_PLACEMENT_3D('',#25240,#17880,#17881);
#15700=AXIS2_PLACEMENT_3D('',#25241,#17882,#17883);
#15701=AXIS2_PLACEMENT_3D('',#25243,#17884,#17885);
#15702=AXIS2_PLACEMENT_3D('',#25244,#17886,#17887);
#15703=AXIS2_PLACEMENT_3D('',#25246,#17889,#17890);
#15704=AXIS2_PLACEMENT_3D('',#25247,#17891,#17892);
#15705=AXIS2_PLACEMENT_3D('',#25248,#17893,#17894);
#15706=AXIS2_PLACEMENT_3D('',#25249,#17895,#17896);
#15707=AXIS2_PLACEMENT_3D('',#25252,#17898,#17899);
#15708=AXIS2_PLACEMENT_3D('',#25257,#17902,#17903);
#15709=AXIS2_PLACEMENT_3D('',#25259,#17905,#17906);
#15710=AXIS2_PLACEMENT_3D('',#25261,#17908,#17909);
#15711=AXIS2_PLACEMENT_3D('',#25263,#17910,#17911);
#15712=AXIS2_PLACEMENT_3D('',#25265,#17912,#17913);
#15713=AXIS2_PLACEMENT_3D('',#25266,#17914,#17915);
#15714=AXIS2_PLACEMENT_3D('',#25267,#17916,#17917);
#15715=AXIS2_PLACEMENT_3D('',#25269,#17918,#17919);
#15716=AXIS2_PLACEMENT_3D('',#25271,#17921,#17922);
#15717=AXIS2_PLACEMENT_3D('',#25273,#17923,#17924);
#15718=AXIS2_PLACEMENT_3D('',#25274,#17925,#17926);
#15719=AXIS2_PLACEMENT_3D('',#25275,#17927,#17928);
#15720=AXIS2_PLACEMENT_3D('',#25277,#17929,#17930);
#15721=AXIS2_PLACEMENT_3D('',#25278,#17931,#17932);
#15722=AXIS2_PLACEMENT_3D('',#25279,#17933,#17934);
#15723=AXIS2_PLACEMENT_3D('',#25281,#17935,#17936);
#15724=AXIS2_PLACEMENT_3D('',#25282,#17937,#17938);
#15725=AXIS2_PLACEMENT_3D('',#25283,#17939,#17940);
#15726=AXIS2_PLACEMENT_3D('',#25285,#17941,#17942);
#15727=AXIS2_PLACEMENT_3D('',#25286,#17943,#17944);
#15728=AXIS2_PLACEMENT_3D('',#25287,#17945,#17946);
#15729=AXIS2_PLACEMENT_3D('',#25290,#17949,#17950);
#15730=AXIS2_PLACEMENT_3D('',#25292,#17951,#17952);
#15731=AXIS2_PLACEMENT_3D('',#25295,#17955,#17956);
#15732=AXIS2_PLACEMENT_3D('',#25297,#17958,#17959);
#15733=AXIS2_PLACEMENT_3D('',#25299,#17961,#17962);
#15734=AXIS2_PLACEMENT_3D('',#25312,#17964,#17965);
#15735=AXIS2_PLACEMENT_3D('',#25314,#17967,#17968);
#15736=AXIS2_PLACEMENT_3D('',#25315,#17969,#17970);
#15737=AXIS2_PLACEMENT_3D('',#25330,#17971,#17972);
#15738=AXIS2_PLACEMENT_3D('',#25331,#17973,#17974);
#15739=AXIS2_PLACEMENT_3D('',#25332,#17975,#17976);
#15740=AXIS2_PLACEMENT_3D('',#25333,#17977,#17978);
#15741=AXIS2_PLACEMENT_3D('',#25335,#17980,#17981);
#15742=AXIS2_PLACEMENT_3D('',#25338,#17983,#17984);
#15743=AXIS2_PLACEMENT_3D('',#25339,#17985,#17986);
#15744=AXIS2_PLACEMENT_3D('',#25342,#17988,#17989);
#15745=AXIS2_PLACEMENT_3D('',#25343,#17990,#17991);
#15746=AXIS2_PLACEMENT_3D('',#25345,#17992,#17993);
#15747=AXIS2_PLACEMENT_3D('',#25346,#17994,#17995);
#15748=AXIS2_PLACEMENT_3D('',#25347,#17996,#17997);
#15749=AXIS2_PLACEMENT_3D('',#25348,#17998,#17999);
#15750=AXIS2_PLACEMENT_3D('',#25350,#18000,#18001);
#15751=AXIS2_PLACEMENT_3D('',#25351,#18002,#18003);
#15752=AXIS2_PLACEMENT_3D('',#25352,#18004,#18005);
#15753=AXIS2_PLACEMENT_3D('',#25353,#18006,#18007);
#15754=AXIS2_PLACEMENT_3D('',#25354,#18008,#18009);
#15755=AXIS2_PLACEMENT_3D('',#25355,#18010,#18011);
#15756=AXIS2_PLACEMENT_3D('',#25356,#18012,#18013);
#15757=AXIS2_PLACEMENT_3D('',#25357,#18014,#18015);
#15758=AXIS2_PLACEMENT_3D('',#25358,#18016,#18017);
#15759=AXIS2_PLACEMENT_3D('',#25359,#18018,#18019);
#15760=AXIS2_PLACEMENT_3D('',#25360,#18020,#18021);
#15761=AXIS2_PLACEMENT_3D('',#25361,#18022,#18023);
#15762=AXIS2_PLACEMENT_3D('',#25362,#18024,#18025);
#15763=AXIS2_PLACEMENT_3D('',#25363,#18026,#18027);
#15764=AXIS2_PLACEMENT_3D('',#25364,#18028,#18029);
#15765=AXIS2_PLACEMENT_3D('',#25365,#18030,#18031);
#15766=AXIS2_PLACEMENT_3D('',#25367,#18033,#18034);
#15767=AXIS2_PLACEMENT_3D('',#25368,#18035,#18036);
#15768=AXIS2_PLACEMENT_3D('',#25370,#18038,#18039);
#15769=AXIS2_PLACEMENT_3D('',#25371,#18040,#18041);
#15770=AXIS2_PLACEMENT_3D('',#25372,#18042,#18043);
#15771=AXIS2_PLACEMENT_3D('',#25373,#18044,#18045);
#15772=AXIS2_PLACEMENT_3D('',#25374,#18046,#18047);
#15773=AXIS2_PLACEMENT_3D('',#25375,#18048,#18049);
#15774=AXIS2_PLACEMENT_3D('',#25377,#18051,#18052);
#15775=AXIS2_PLACEMENT_3D('',#25379,#18054,#18055);
#15776=AXIS2_PLACEMENT_3D('',#25381,#18056,#18057);
#15777=AXIS2_PLACEMENT_3D('',#25383,#18059,#18060);
#15778=AXIS2_PLACEMENT_3D('',#25385,#18062,#18063);
#15779=AXIS2_PLACEMENT_3D('',#25387,#18065,#18066);
#15780=AXIS2_PLACEMENT_3D('',#25388,#18067,#18068);
#15781=AXIS2_PLACEMENT_3D('',#25389,#18069,#18070);
#15782=AXIS2_PLACEMENT_3D('',#25390,#18071,#18072);
#15783=AXIS2_PLACEMENT_3D('',#25391,#18073,#18074);
#15784=AXIS2_PLACEMENT_3D('',#25392,#18075,#18076);
#15785=AXIS2_PLACEMENT_3D('',#25393,#18077,#18078);
#15786=AXIS2_PLACEMENT_3D('',#25394,#18079,#18080);
#15787=AXIS2_PLACEMENT_3D('',#25395,#18081,#18082);
#15788=AXIS2_PLACEMENT_3D('',#25396,#18083,#18084);
#15789=AXIS2_PLACEMENT_3D('',#25397,#18085,#18086);
#15790=AXIS2_PLACEMENT_3D('',#25398,#18087,#18088);
#15791=AXIS2_PLACEMENT_3D('',#25399,#18089,#18090);
#15792=AXIS2_PLACEMENT_3D('',#25400,#18091,#18092);
#15793=AXIS2_PLACEMENT_3D('',#25403,#18094,#18095);
#15794=AXIS2_PLACEMENT_3D('',#25404,#18096,#18097);
#15795=AXIS2_PLACEMENT_3D('',#25406,#18098,#18099);
#15796=AXIS2_PLACEMENT_3D('',#25407,#18100,#18101);
#15797=AXIS2_PLACEMENT_3D('',#25409,#18103,#18104);
#15798=AXIS2_PLACEMENT_3D('',#25410,#18105,#18106);
#17363=DIRECTION('axis',(0.,0.,1.));
#17364=DIRECTION('refdir',(1.,0.,0.));
#17365=DIRECTION('center_axis',(-1.,0.,0.));
#17366=DIRECTION('ref_axis',(0.,-1.,0.));
#17367=DIRECTION('center_axis',(-1.,0.,0.));
#17368=DIRECTION('ref_axis',(0.,-1.,0.));
#17369=DIRECTION('',(0.707106781186552,-0.707106781186543,8.65956056235488E-17));
#17370=DIRECTION('center_axis',(1.,0.,0.));
#17371=DIRECTION('ref_axis',(0.,-1.,0.));
#17372=DIRECTION('center_axis',(1.,0.,0.));
#17373=DIRECTION('ref_axis',(0.,-1.,0.));
#17374=DIRECTION('center_axis',(1.,0.,0.));
#17375=DIRECTION('ref_axis',(0.,0.,-1.));
#17376=DIRECTION('center_axis',(1.,0.,0.));
#17377=DIRECTION('ref_axis',(0.,0.,-1.));
#17378=DIRECTION('center_axis',(1.,0.,0.));
#17379=DIRECTION('ref_axis',(0.,1.,0.));
#17380=DIRECTION('',(1.,0.,0.));
#17381=DIRECTION('center_axis',(1.,0.,0.));
#17382=DIRECTION('ref_axis',(0.,0.,-1.));
#17383=DIRECTION('center_axis',(0.,-1.,0.));
#17384=DIRECTION('ref_axis',(1.,0.,0.));
#17385=DIRECTION('center_axis',(0.,-1.,0.));
#17386=DIRECTION('ref_axis',(1.,0.,0.));
#17387=DIRECTION('',(0.707106781186554,0.707106781186541,8.65956056235501E-17));
#17388=DIRECTION('center_axis',(0.,1.,0.));
#17389=DIRECTION('ref_axis',(1.,0.,0.));
#17390=DIRECTION('center_axis',(0.,-1.,0.));
#17391=DIRECTION('ref_axis',(1.,0.,0.));
#17392=DIRECTION('center_axis',(0.,-1.,0.));
#17393=DIRECTION('ref_axis',(-1.,0.,0.));
#17394=DIRECTION('',(1.,0.,0.));
#17395=DIRECTION('center_axis',(0.,-1.,0.));
#17396=DIRECTION('ref_axis',(1.,0.,0.));
#17397=DIRECTION('',(0.,0.,1.));
#17398=DIRECTION('center_axis',(0.,-1.,0.));
#17399=DIRECTION('ref_axis',(1.,0.,0.));
#17400=DIRECTION('',(-1.,0.,0.));
#17401=DIRECTION('center_axis',(0.,-1.,0.));
#17402=DIRECTION('ref_axis',(-1.,0.,0.));
#17403=DIRECTION('',(0.,0.,-1.));
#17404=DIRECTION('center_axis',(0.,1.,0.));
#17405=DIRECTION('ref_axis',(1.,0.,0.));
#17406=DIRECTION('',(0.,1.,0.));
#17407=DIRECTION('center_axis',(0.,1.,0.));
#17408=DIRECTION('ref_axis',(1.,0.,0.));
#17409=DIRECTION('center_axis',(0.,-1.,0.));
#17410=DIRECTION('ref_axis',(-1.,0.,0.));
#17411=DIRECTION('',(-0.555969453910032,0.707106781186556,0.436918718206223));
#17412=DIRECTION('center_axis',(0.,1.,0.));
#17413=DIRECTION('ref_axis',(-1.,0.,0.));
#17414=DIRECTION('center_axis',(0.,1.,0.));
#17415=DIRECTION('ref_axis',(-1.,0.,0.));
#17416=DIRECTION('',(-0.450316983320678,-0.707106781186556,0.545173930533139));
#17417=DIRECTION('',(0.406052535411294,-0.675506402763447,0.615477406824692));
#17418=DIRECTION('',(0.406052535411299,0.675506402763456,-0.615477406824679));
#17419=DIRECTION('center_axis',(0.,-1.,0.));
#17420=DIRECTION('ref_axis',(1.,0.,0.));
#17421=DIRECTION('',(-0.450316983320678,0.707106781186556,-0.545173930533139));
#17422=DIRECTION('center_axis',(0.,1.,0.));
#17423=DIRECTION('ref_axis',(1.,0.,0.));
#17424=DIRECTION('',(0.555969453910031,-0.707106781186554,0.436918718206228));
#17425=DIRECTION('center_axis',(0.,-1.,0.));
#17426=DIRECTION('ref_axis',(1.,0.,0.));
#17427=DIRECTION('',(0.628668104787158,-0.674217950114304,-0.387564923292846));
#17428=DIRECTION('',(-0.628668104787152,0.674217950114311,-0.387564923292843));
#17429=DIRECTION('center_axis',(0.,-1.,0.));
#17430=DIRECTION('ref_axis',(1.,0.,0.));
#17431=DIRECTION('',(0.,0.,-1.));
#17432=DIRECTION('',(1.,0.,0.));
#17433=DIRECTION('center_axis',(0.,0.,1.));
#17434=DIRECTION('ref_axis',(0.707106781186538,-0.707106781186557,0.));
#17435=DIRECTION('',(0.,0.,-1.));
#17436=DIRECTION('center_axis',(0.,0.,-1.));
#17437=DIRECTION('ref_axis',(0.707106781186543,-0.707106781186552,0.));
#17438=DIRECTION('',(0.,0.,1.));
#17439=DIRECTION('center_axis',(0.,0.,1.));
#17440=DIRECTION('ref_axis',(0.707106781186543,-0.707106781186552,0.));
#17441=DIRECTION('center_axis',(0.,1.,0.));
#17442=DIRECTION('ref_axis',(1.,0.,0.));
#17443=DIRECTION('',(0.,1.,0.));
#17444=DIRECTION('center_axis',(0.,1.,0.));
#17445=DIRECTION('ref_axis',(1.,0.,0.));
#17446=DIRECTION('center_axis',(0.,-1.,0.));
#17447=DIRECTION('ref_axis',(1.,0.,0.));
#17448=DIRECTION('',(-0.450316983320678,0.707106781186556,-0.545173930533139));
#17449=DIRECTION('center_axis',(0.,1.,0.));
#17450=DIRECTION('ref_axis',(1.,0.,0.));
#17451=DIRECTION('',(-0.469605266894875,-0.707106781186553,-0.528650066967352));
#17452=DIRECTION('',(-0.52464839659846,-0.683785150909193,0.507131075110525));
#17453=DIRECTION('',(0.524648396598484,0.683785150909177,0.507131075110523));
#17454=DIRECTION('center_axis',(0.,-1.,0.));
#17455=DIRECTION('ref_axis',(-1.,0.,0.));
#17456=DIRECTION('',(0.469605266894875,0.707106781186553,-0.528650066967352));
#17457=DIRECTION('center_axis',(0.,1.,0.));
#17458=DIRECTION('ref_axis',(-1.,0.,0.));
#17459=DIRECTION('',(-0.450316983320678,-0.707106781186556,0.545173930533139));
#17460=DIRECTION('center_axis',(0.,-1.,0.));
#17461=DIRECTION('ref_axis',(-1.,0.,0.));
#17462=DIRECTION('',(0.406052535411297,-0.675506402763453,0.615477406824684));
#17463=DIRECTION('',(0.406052535411268,0.675506402763462,-0.615477406824693));
#17464=DIRECTION('center_axis',(0.,-1.,0.));
#17465=DIRECTION('ref_axis',(1.,0.,0.));
#17466=DIRECTION('',(1.,0.,0.));
#17467=DIRECTION('',(0.,0.,1.));
#17468=DIRECTION('center_axis',(1.,0.,0.));
#17469=DIRECTION('ref_axis',(0.,-0.707106781186549,0.707106781186546));
#17470=DIRECTION('center_axis',(-1.,0.,0.));
#17471=DIRECTION('ref_axis',(0.,-1.,0.));
#17472=DIRECTION('',(-1.,0.,0.));
#17473=DIRECTION('center_axis',(-1.,0.,0.));
#17474=DIRECTION('ref_axis',(0.,0.,1.));
#17475=DIRECTION('center_axis',(0.,1.,0.));
#17476=DIRECTION('ref_axis',(1.,0.,0.));
#17477=DIRECTION('',(0.,1.,0.));
#17478=DIRECTION('center_axis',(0.,1.,0.));
#17479=DIRECTION('ref_axis',(1.,0.,0.));
#17480=DIRECTION('center_axis',(0.,-1.,0.));
#17481=DIRECTION('ref_axis',(1.,0.,0.));
#17482=DIRECTION('',(-0.555969453910031,0.707106781186554,0.436918718206228));
#17483=DIRECTION('center_axis',(0.,1.,0.));
#17484=DIRECTION('ref_axis',(1.,0.,0.));
#17485=DIRECTION('',(0.450316983320677,-0.707106781186554,-0.545173930533143));
#17486=DIRECTION('center_axis',(0.,-1.,0.));
#17487=DIRECTION('ref_axis',(1.,0.,0.));
#17488=DIRECTION('',(-0.406052535411294,-0.675506402763435,-0.615477406824705));
#17489=DIRECTION('',(-0.406052535411254,0.675506402763442,0.615477406824724));
#17490=DIRECTION('center_axis',(0.,-1.,0.));
#17491=DIRECTION('ref_axis',(-1.,0.,0.));
#17492=DIRECTION('',(0.450316983320678,0.707106781186556,0.545173930533139));
#17493=DIRECTION('center_axis',(0.,1.,0.));
#17494=DIRECTION('ref_axis',(-1.,0.,0.));
#17495=DIRECTION('center_axis',(0.,1.,0.));
#17496=DIRECTION('ref_axis',(-1.,0.,0.));
#17497=DIRECTION('',(0.555969453910031,-0.707106781186554,0.436918718206228));
#17498=DIRECTION('',(0.628668104787149,-0.674217950114307,-0.387564923292854));
#17499=DIRECTION('',(-0.628668104787158,0.674217950114304,-0.387564923292846));
#17500=DIRECTION('center_axis',(0.,1.,0.));
#17501=DIRECTION('ref_axis',(1.,0.,0.));
#17502=DIRECTION('',(0.,1.,0.));
#17503=DIRECTION('center_axis',(0.,1.,0.));
#17504=DIRECTION('ref_axis',(1.,0.,0.));
#17505=DIRECTION('center_axis',(0.,-1.,0.));
#17506=DIRECTION('ref_axis',(1.,0.,0.));
#17507=DIRECTION('',(0.469605266894875,0.707106781186553,-0.528650066967352));
#17508=DIRECTION('center_axis',(0.,1.,0.));
#17509=DIRECTION('ref_axis',(1.,0.,0.));
#17510=DIRECTION('',(0.450316983320697,-0.707106781186546,-0.545173930533137));
#17511=DIRECTION('',(-0.406052535411294,-0.675506402763447,-0.615477406824692));
#17512=DIRECTION('',(-0.406052535411272,0.675506402763455,0.615477406824698));
#17513=DIRECTION('center_axis',(0.,-1.,0.));
#17514=DIRECTION('ref_axis',(-1.,0.,0.));
#17515=DIRECTION('',(0.450316983320697,0.707106781186546,0.545173930533137));
#17516=DIRECTION('center_axis',(0.,1.,0.));
#17517=DIRECTION('ref_axis',(-1.,0.,0.));
#17518=DIRECTION('',(-0.469605266894875,-0.707106781186553,-0.528650066967352));
#17519=DIRECTION('center_axis',(0.,-1.,0.));
#17520=DIRECTION('ref_axis',(-1.,0.,0.));
#17521=DIRECTION('',(-0.524648396598479,-0.683785150909184,0.507131075110518));
#17522=DIRECTION('',(0.524648396598465,0.683785150909186,0.50713107511053));
#17523=DIRECTION('center_axis',(0.,-1.,0.));
#17524=DIRECTION('ref_axis',(1.,0.,0.));
#17525=DIRECTION('',(0.,0.,1.));
#17526=DIRECTION('',(-1.,0.,0.));
#17527=DIRECTION('center_axis',(0.,0.,1.));
#17528=DIRECTION('ref_axis',(-0.707106781186544,-0.707106781186551,0.));
#17529=DIRECTION('center_axis',(0.,0.,1.));
#17530=DIRECTION('ref_axis',(0.,-1.,0.));
#17531=DIRECTION('',(0.,0.,-1.));
#17532=DIRECTION('center_axis',(0.,0.,-1.));
#17533=DIRECTION('ref_axis',(-1.,0.,0.));
#17534=DIRECTION('center_axis',(0.,1.,0.));
#17535=DIRECTION('ref_axis',(1.,0.,0.));
#17536=DIRECTION('',(0.,1.,0.));
#17537=DIRECTION('center_axis',(0.,1.,0.));
#17538=DIRECTION('ref_axis',(1.,0.,0.));
#17539=DIRECTION('',(-0.706933664902991,-0.171973946473105,-0.686053755300042));
#17540=DIRECTION('center_axis',(-1.,0.,0.));
#17541=DIRECTION('ref_axis',(0.,-0.946352857512202,0.323135063214268));
#17542=DIRECTION('center_axis',(1.,0.,0.));
#17543=DIRECTION('ref_axis',(0.,-0.946352857512203,0.323135063214268));
#17544=DIRECTION('',(0.707106781186544,0.186221003615294,0.682144953666387));
#17545=DIRECTION('center_axis',(-1.,0.,0.));
#17546=DIRECTION('ref_axis',(0.,-0.946352857512202,0.323135063214268));
#17547=DIRECTION('center_axis',(-1.,0.,0.));
#17548=DIRECTION('ref_axis',(0.,0.946352857512202,-0.323135063214268));
#17549=DIRECTION('',(-1.,0.,0.));
#17550=DIRECTION('center_axis',(-1.,0.,0.));
#17551=DIRECTION('ref_axis',(0.,0.946352857512202,-0.323135063214268));
#17552=DIRECTION('',(1.,0.,0.));
#17553=DIRECTION('',(0.706933664902985,0.171973946473104,-0.686053755300049));
#17554=DIRECTION('center_axis',(-1.,0.,0.));
#17555=DIRECTION('ref_axis',(0.,-0.946352857512202,-0.323135063214268));
#17556=DIRECTION('',(-0.707106781186544,-0.186221003615294,0.682144953666387));
#17557=DIRECTION('center_axis',(1.,0.,0.));
#17558=DIRECTION('ref_axis',(0.,-0.946352857512203,-0.323135063214268));
#17559=DIRECTION('center_axis',(-1.,0.,0.));
#17560=DIRECTION('ref_axis',(0.,-0.946352857512202,-0.323135063214268));
#17561=DIRECTION('center_axis',(-1.,0.,0.));
#17562=DIRECTION('ref_axis',(0.,0.660980889208583,-0.750402734603914));
#17563=DIRECTION('center_axis',(1.,0.,0.));
#17564=DIRECTION('ref_axis',(0.,0.707106781186548,-0.707106781186548));
#17565=DIRECTION('center_axis',(0.,-0.945990172710258,0.324195300915385));
#17566=DIRECTION('ref_axis',(1.,0.,0.));
#17567=DIRECTION('center_axis',(-1.,0.,0.));
#17568=DIRECTION('ref_axis',(0.,0.707106781186548,-0.707106781186548));
#17569=DIRECTION('center_axis',(1.,0.,0.));
#17570=DIRECTION('ref_axis',(0.,0.,-1.));
#17571=DIRECTION('center_axis',(1.,0.,0.));
#17572=DIRECTION('ref_axis',(0.,0.707106781186548,0.707106781186548));
#17573=DIRECTION('center_axis',(-1.,0.,0.));
#17574=DIRECTION('ref_axis',(0.,-0.178029704061997,-0.984025113740294));
#17575=DIRECTION('',(0.,-1.,0.));
#17576=DIRECTION('center_axis',(-1.,0.,0.));
#17577=DIRECTION('ref_axis',(0.,0.178029704061997,-0.984025113740294));
#17578=DIRECTION('center_axis',(1.,0.,0.));
#17579=DIRECTION('ref_axis',(0.,-0.707106781186547,0.707106781186548));
#17580=DIRECTION('center_axis',(-1.,0.,0.));
#17581=DIRECTION('ref_axis',(0.,0.939379515438772,-0.342879171099701));
#17582=DIRECTION('',(0.,-1.,0.));
#17583=DIRECTION('',(0.,0.,-1.));
#17584=DIRECTION('',(0.,1.,0.));
#17585=DIRECTION('center_axis',(-1.,0.,0.));
#17586=DIRECTION('ref_axis',(0.,0.939379515438772,0.342879171099701));
#17587=DIRECTION('center_axis',(1.,0.,0.));
#17588=DIRECTION('ref_axis',(0.,-0.707106781186548,-0.707106781186547));
#17589=DIRECTION('center_axis',(-1.,0.,0.));
#17590=DIRECTION('ref_axis',(0.,0.326047170834313,0.945353501284541));
#17591=DIRECTION('',(0.,1.,0.));
#17592=DIRECTION('center_axis',(-1.,0.,0.));
#17593=DIRECTION('ref_axis',(0.,-0.326047170834313,0.945353501284541));
#17594=DIRECTION('',(0.,1.,0.));
#17595=DIRECTION('',(0.,1.,0.));
#17596=DIRECTION('center_axis',(0.,1.,0.));
#17597=DIRECTION('ref_axis',(1.,0.,0.));
#17598=DIRECTION('center_axis',(0.,1.,0.));
#17599=DIRECTION('ref_axis',(1.,0.,0.));
#17600=DIRECTION('',(0.707106781186554,-0.707106781186541,-8.65956056235501E-17));
#17601=DIRECTION('center_axis',(0.,-1.,0.));
#17602=DIRECTION('ref_axis',(1.,0.,0.));
#17603=DIRECTION('center_axis',(0.,1.,0.));
#17604=DIRECTION('ref_axis',(-1.,0.,0.));
#17605=DIRECTION('',(0.,0.,-1.));
#17606=DIRECTION('',(-1.,0.,0.));
#17607=DIRECTION('',(0.,0.,1.));
#17608=DIRECTION('',(1.,0.,0.));
#17609=DIRECTION('center_axis',(0.,1.,0.));
#17610=DIRECTION('ref_axis',(1.,0.,0.));
#17611=DIRECTION('center_axis',(0.,1.,0.));
#17612=DIRECTION('ref_axis',(1.,0.,0.));
#17613=DIRECTION('center_axis',(0.,1.,0.));
#17614=DIRECTION('ref_axis',(1.,0.,0.));
#17615=DIRECTION('center_axis',(0.,1.,0.));
#17616=DIRECTION('ref_axis',(1.,0.,0.));
#17617=DIRECTION('center_axis',(0.,-1.,0.));
#17618=DIRECTION('ref_axis',(1.,0.,0.));
#17619=DIRECTION('',(0.,-1.,0.));
#17620=DIRECTION('center_axis',(0.,-1.,0.));
#17621=DIRECTION('ref_axis',(1.,0.,0.));
#17622=DIRECTION('center_axis',(0.,1.,0.));
#17623=DIRECTION('ref_axis',(1.,0.,0.));
#17624=DIRECTION('',(0.707106781186554,-0.707106781186541,-8.65956056235501E-17));
#17625=DIRECTION('center_axis',(0.,-1.,0.));
#17626=DIRECTION('ref_axis',(1.,0.,0.));
#17627=DIRECTION('center_axis',(0.,-1.,0.));
#17628=DIRECTION('ref_axis',(1.,0.,0.));
#17629=DIRECTION('',(0.,-1.,0.));
#17630=DIRECTION('center_axis',(0.,-1.,0.));
#17631=DIRECTION('ref_axis',(1.,0.,0.));
#17632=DIRECTION('center_axis',(0.,1.,0.));
#17633=DIRECTION('ref_axis',(1.,0.,0.));
#17634=DIRECTION('',(0.707106781186554,-0.707106781186541,-8.65956056235501E-17));
#17635=DIRECTION('center_axis',(0.,-1.,0.));
#17636=DIRECTION('ref_axis',(1.,0.,0.));
#17637=DIRECTION('center_axis',(0.,-1.,0.));
#17638=DIRECTION('ref_axis',(1.,0.,0.));
#17639=DIRECTION('',(0.,-1.,0.));
#17640=DIRECTION('center_axis',(0.,-1.,0.));
#17641=DIRECTION('ref_axis',(1.,0.,0.));
#17642=DIRECTION('center_axis',(0.,1.,0.));
#17643=DIRECTION('ref_axis',(1.,0.,0.));
#17644=DIRECTION('',(0.707106781186554,-0.707106781186541,-8.65956056235501E-17));
#17645=DIRECTION('center_axis',(0.,-1.,0.));
#17646=DIRECTION('ref_axis',(1.,0.,0.));
#17647=DIRECTION('center_axis',(0.,-1.,0.));
#17648=DIRECTION('ref_axis',(1.,0.,0.));
#17649=DIRECTION('',(0.,-1.,0.));
#17650=DIRECTION('center_axis',(0.,-1.,0.));
#17651=DIRECTION('ref_axis',(1.,0.,0.));
#17652=DIRECTION('center_axis',(0.,1.,0.));
#17653=DIRECTION('ref_axis',(1.,0.,0.));
#17654=DIRECTION('',(0.707106781186554,-0.707106781186541,-8.65956056235501E-17));
#17655=DIRECTION('center_axis',(0.,-1.,0.));
#17656=DIRECTION('ref_axis',(1.,0.,0.));
#17657=DIRECTION('center_axis',(0.,-1.,0.));
#17658=DIRECTION('ref_axis',(1.,0.,0.));
#17659=DIRECTION('',(0.,-1.,0.));
#17660=DIRECTION('center_axis',(0.,-1.,0.));
#17661=DIRECTION('ref_axis',(1.,0.,0.));
#17662=DIRECTION('center_axis',(0.,1.,0.));
#17663=DIRECTION('ref_axis',(0.718378767037319,0.,-0.695652173913042));
#17664=DIRECTION('center_axis',(1.,0.,0.));
#17665=DIRECTION('ref_axis',(0.,0.,-1.));
#17666=DIRECTION('center_axis',(1.,0.,0.));
#17667=DIRECTION('ref_axis',(0.,0.,-1.));
#17668=DIRECTION('',(1.,0.,0.));
#17669=DIRECTION('center_axis',(0.,-1.,0.));
#17670=DIRECTION('ref_axis',(-0.707106781186552,0.,-0.707106781186543));
#17671=DIRECTION('center_axis',(0.,-1.,0.));
#17672=DIRECTION('ref_axis',(-1.,0.,0.));
#17673=DIRECTION('',(0.,-1.,0.));
#17674=DIRECTION('',(0.,1.,0.));
#17675=DIRECTION('center_axis',(-0.408248290463861,-0.816496580927726,0.408248290463865));
#17676=DIRECTION('ref_axis',(-0.577350269189623,0.577350269189627,0.577350269189627));
#17677=DIRECTION('center_axis',(-1.,0.,0.));
#17678=DIRECTION('ref_axis',(0.,1.,0.));
#17679=DIRECTION('center_axis',(0.,0.,1.));
#17680=DIRECTION('ref_axis',(-1.,0.,0.));
#17681=DIRECTION('center_axis',(0.,1.,0.));
#17682=DIRECTION('ref_axis',(0.,0.,1.));
#17683=DIRECTION('center_axis',(0.,0.,1.));
#17684=DIRECTION('ref_axis',(-0.707106781186544,0.707106781186551,0.));
#17685=DIRECTION('center_axis',(0.,0.,1.));
#17686=DIRECTION('ref_axis',(0.,1.,0.));
#17687=DIRECTION('',(0.,0.,1.));
#17688=DIRECTION('center_axis',(0.,-1.,0.));
#17689=DIRECTION('ref_axis',(-0.707106781186546,0.,0.707106781186549));
#17690=DIRECTION('',(0.,1.,0.));
#17691=DIRECTION('',(0.,-1.,0.));
#17692=DIRECTION('center_axis',(-1.,0.,0.));
#17693=DIRECTION('ref_axis',(0.,0.707106781186549,0.707106781186546));
#17694=DIRECTION('center_axis',(-1.,0.,0.));
#17695=DIRECTION('ref_axis',(0.,0.,1.));
#17696=DIRECTION('',(1.,0.,0.));
#17697=DIRECTION('center_axis',(0.40824829046386,-0.40824829046386,-0.816496580927729));
#17698=DIRECTION('ref_axis',(-0.577350269189629,0.577350269189625,-0.577350269189623));
#17699=DIRECTION('center_axis',(-1.,0.,0.));
#17700=DIRECTION('ref_axis',(0.,0.70710678118655,-0.707106781186545));
#17701=DIRECTION('center_axis',(0.,1.,0.));
#17702=DIRECTION('ref_axis',(0.70710678118654,0.,0.707106781186555));
#17703=DIRECTION('center_axis',(0.,-1.,0.));
#17704=DIRECTION('ref_axis',(1.,0.,-2.22044604925032E-15));
#17705=DIRECTION('',(0.,-1.,0.));
#17706=DIRECTION('center_axis',(0.408248290463861,0.408248290463857,-0.81649658092773));
#17707=DIRECTION('ref_axis',(0.577350269189634,0.577350269189623,0.57735026918962));
#17708=DIRECTION('center_axis',(0.,0.,1.));
#17709=DIRECTION('ref_axis',(0.707106781186548,0.707106781186548,0.));
#17710=DIRECTION('center_axis',(0.,0.,1.));
#17711=DIRECTION('ref_axis',(1.,0.,0.));
#17712=DIRECTION('',(-1.,0.,0.));
#17713=DIRECTION('',(0.,1.,0.));
#17714=DIRECTION('',(1.,0.,0.));
#17715=DIRECTION('center_axis',(-1.,0.,0.));
#17716=DIRECTION('ref_axis',(0.,0.707106781186549,-0.707106781186546));
#17717=DIRECTION('center_axis',(-1.,0.,0.));
#17718=DIRECTION('ref_axis',(0.,1.,0.));
#17719=DIRECTION('center_axis',(0.,0.,1.));
#17720=DIRECTION('ref_axis',(0.707106781186551,0.707106781186544,0.));
#17721=DIRECTION('center_axis',(0.,0.,-1.));
#17722=DIRECTION('ref_axis',(0.707106781186548,0.707106781186548,0.));
#17723=DIRECTION('center_axis',(0.408248290463865,-0.816496580927724,-0.408248290463865));
#17724=DIRECTION('ref_axis',(-0.577350269189621,-0.577350269189628,0.577350269189628));
#17725=DIRECTION('center_axis',(0.,-1.,0.));
#17726=DIRECTION('ref_axis',(-1.,0.,0.));
#17727=DIRECTION('center_axis',(0.408248290463873,0.408248290463858,-0.816496580927724));
#17728=DIRECTION('ref_axis',(-0.577350269189634,-0.57735026918962,-0.577350269189623));
#17729=DIRECTION('center_axis',(-4.4408920985006E-15,-1.,0.));
#17730=DIRECTION('ref_axis',(0.,0.,-1.));
#17731=DIRECTION('center_axis',(-1.,0.,-8.88178419700124E-15));
#17732=DIRECTION('ref_axis',(0.,-1.,0.));
#17733=DIRECTION('center_axis',(0.,-1.,0.));
#17734=DIRECTION('ref_axis',(-0.707106781186554,0.,-0.707106781186541));
#17735=DIRECTION('',(0.,-1.,0.));
#17736=DIRECTION('',(0.,1.,0.));
#17737=DIRECTION('center_axis',(1.,0.,0.));
#17738=DIRECTION('ref_axis',(0.,-0.707106781186548,-0.707106781186548));
#17739=DIRECTION('',(1.,0.,0.));
#17740=DIRECTION('center_axis',(-1.,1.77635683940026E-14,0.));
#17741=DIRECTION('ref_axis',(0.,0.,-1.));
#17742=DIRECTION('',(-1.,0.,0.));
#17743=DIRECTION('center_axis',(-0.816496580927736,-0.408248290463854,-0.408248290463854));
#17744=DIRECTION('ref_axis',(0.577350269189608,-0.577350269189637,-0.577350269189633));
#17745=DIRECTION('center_axis',(0.,-1.,0.));
#17746=DIRECTION('ref_axis',(0.707106781186543,0.,-0.707106781186552));
#17747=DIRECTION('center_axis',(-0.81649658092773,-0.408248290463858,0.408248290463861));
#17748=DIRECTION('ref_axis',(0.577350269189622,-0.577350269189629,0.577350269189626));
#17749=DIRECTION('center_axis',(0.,-1.,0.));
#17750=DIRECTION('ref_axis',(0.707106781186543,0.,0.707106781186552));
#17751=DIRECTION('center_axis',(0.,-1.,0.));
#17752=DIRECTION('ref_axis',(-0.707106781186548,0.,0.707106781186548));
#17753=DIRECTION('',(0.,-1.,0.));
#17754=DIRECTION('',(0.,1.,0.));
#17755=DIRECTION('center_axis',(0.,1.,0.));
#17756=DIRECTION('ref_axis',(0.707106781186541,0.,-0.707106781186554));
#17757=DIRECTION('',(0.,1.,0.));
#17758=DIRECTION('center_axis',(0.,0.,1.));
#17759=DIRECTION('ref_axis',(1.,0.,0.));
#17760=DIRECTION('',(-1.,0.,0.));
#17761=DIRECTION('center_axis',(0.,-1.,0.));
#17762=DIRECTION('ref_axis',(1.,0.,0.));
#17763=DIRECTION('center_axis',(1.,0.,0.));
#17764=DIRECTION('ref_axis',(0.,0.,-1.));
#17765=DIRECTION('center_axis',(1.,0.,0.));
#17766=DIRECTION('ref_axis',(0.,0.694365074829414,-0.719622917128924));
#17767=DIRECTION('',(0.,1.,0.));
#17768=DIRECTION('center_axis',(1.,0.,0.));
#17769=DIRECTION('ref_axis',(0.,-0.566946709513841,-0.823754471047914));
#17770=DIRECTION('center_axis',(1.,0.,0.));
#17771=DIRECTION('ref_axis',(0.,-0.566946709513841,0.823754471047914));
#17772=DIRECTION('',(0.,-1.,0.));
#17773=DIRECTION('center_axis',(1.,0.,0.));
#17774=DIRECTION('ref_axis',(0.,0.694365074829414,0.719622917128924));
#17775=DIRECTION('center_axis',(-1.,0.,0.));
#17776=DIRECTION('ref_axis',(0.,1.,0.));
#17777=DIRECTION('center_axis',(1.,0.,0.));
#17778=DIRECTION('ref_axis',(0.,0.,-1.));
#17779=DIRECTION('center_axis',(1.,0.,0.));
#17780=DIRECTION('ref_axis',(0.,0.,-1.));
#17781=DIRECTION('center_axis',(1.,0.,0.));
#17782=DIRECTION('ref_axis',(0.,0.,-1.));
#17783=DIRECTION('center_axis',(1.,0.,0.));
#17784=DIRECTION('ref_axis',(0.,0.,-1.));
#17785=DIRECTION('center_axis',(1.,0.,0.));
#17786=DIRECTION('ref_axis',(0.,0.,-1.));
#17787=DIRECTION('center_axis',(0.,-1.,-1.22464679914735E-16));
#17788=DIRECTION('ref_axis',(0.,-1.22464679914735E-16,1.));
#17789=DIRECTION('center_axis',(1.,0.,0.));
#17790=DIRECTION('ref_axis',(0.,1.,0.));
#17791=DIRECTION('center_axis',(1.,0.,0.));
#17792=DIRECTION('ref_axis',(0.,1.,0.));
#17793=DIRECTION('center_axis',(1.,0.,0.));
#17794=DIRECTION('ref_axis',(0.,1.,0.));
#17795=DIRECTION('',(1.,0.,0.));
#17796=DIRECTION('center_axis',(1.,0.,0.));
#17797=DIRECTION('ref_axis',(0.,0.,-1.));
#17798=DIRECTION('center_axis',(1.,0.,0.));
#17799=DIRECTION('ref_axis',(0.,0.,-1.));
#17800=DIRECTION('center_axis',(0.,-1.,0.));
#17801=DIRECTION('ref_axis',(-1.,0.,0.));
#17802=DIRECTION('center_axis',(-1.,0.,0.));
#17803=DIRECTION('ref_axis',(0.,-0.566946709513841,-0.823754471047914));
#17804=DIRECTION('center_axis',(0.,1.,0.));
#17805=DIRECTION('ref_axis',(-0.707106781186544,0.,-0.707106781186551));
#17806=DIRECTION('center_axis',(0.,-1.,2.22044604925031E-15));
#17807=DIRECTION('ref_axis',(-1.,0.,0.));
#17808=DIRECTION('',(0.,-1.,0.));
#17809=DIRECTION('center_axis',(1.,0.,0.));
#17810=DIRECTION('ref_axis',(0.,0.,-1.));
#17811=DIRECTION('center_axis',(-1.,0.,0.));
#17812=DIRECTION('ref_axis',(0.,0.694365074829414,-0.719622917128924));
#17813=DIRECTION('center_axis',(0.,-1.,1.63845976266357E-14));
#17814=DIRECTION('ref_axis',(0.316350739523702,1.55431223447523E-14,0.948642298025345));
#17815=DIRECTION('center_axis',(0.,-1.304735096307E-15,1.));
#17816=DIRECTION('ref_axis',(-1.,0.,0.));
#17817=DIRECTION('center_axis',(1.,0.,0.));
#17818=DIRECTION('ref_axis',(0.,0.,-1.));
#17819=DIRECTION('center_axis',(1.,0.,0.));
#17820=DIRECTION('ref_axis',(0.,0.,-1.));
#17821=DIRECTION('center_axis',(1.,0.,0.));
#17822=DIRECTION('ref_axis',(0.,0.,-1.));
#17823=DIRECTION('center_axis',(1.,0.,0.));
#17824=DIRECTION('ref_axis',(0.,-0.704542565014449,-0.709661732153327));
#17825=DIRECTION('center_axis',(-1.,0.,0.));
#17826=DIRECTION('ref_axis',(0.,-0.704542565014449,-0.709661732153327));
#17827=DIRECTION('center_axis',(1.,0.,0.));
#17828=DIRECTION('ref_axis',(0.,0.,-1.));
#17829=DIRECTION('center_axis',(-1.,0.,0.));
#17830=DIRECTION('ref_axis',(0.,-0.999903350347485,0.0139028761007986));
#17831=DIRECTION('center_axis',(-1.,0.,0.));
#17832=DIRECTION('ref_axis',(0.,0.,-1.));
#17833=DIRECTION('center_axis',(-1.,0.,0.));
#17834=DIRECTION('ref_axis',(0.,0.,-1.));
#17835=DIRECTION('center_axis',(1.,0.,0.));
#17836=DIRECTION('ref_axis',(0.,0.,-1.));
#17837=DIRECTION('center_axis',(-1.,0.,0.));
#17838=DIRECTION('ref_axis',(0.,-0.704542565014449,0.709661732153327));
#17839=DIRECTION('center_axis',(1.,0.,0.));
#17840=DIRECTION('ref_axis',(0.,-0.704542565014449,0.709661732153327));
#17841=DIRECTION('center_axis',(1.,0.,0.));
#17842=DIRECTION('ref_axis',(0.,-1.58603289232165E-16,1.));
#17843=DIRECTION('',(-1.,0.,0.));
#17844=DIRECTION('center_axis',(1.,0.,0.));
#17845=DIRECTION('ref_axis',(0.,-0.326047170834313,0.945353501284541));
#17846=DIRECTION('',(1.,0.,0.));
#17847=DIRECTION('center_axis',(-1.,0.,0.));
#17848=DIRECTION('ref_axis',(0.,-0.566946709513841,0.823754471047914));
#17849=DIRECTION('',(1.,0.,0.));
#17850=DIRECTION('center_axis',(-1.,0.,0.));
#17851=DIRECTION('ref_axis',(0.,0.,1.));
#17852=DIRECTION('center_axis',(-1.,0.,0.));
#17853=DIRECTION('ref_axis',(0.,0.707106781186547,-0.707106781186548));
#17854=DIRECTION('center_axis',(1.,0.,0.));
#17855=DIRECTION('ref_axis',(0.,0.707106781186547,-0.707106781186548));
#17856=DIRECTION('center_axis',(1.,0.,0.));
#17857=DIRECTION('ref_axis',(0.,0.,-1.));
#17858=DIRECTION('center_axis',(-1.,0.,0.));
#17859=DIRECTION('ref_axis',(0.,-0.0139028761007986,-0.999903350347485));
#17860=DIRECTION('center_axis',(-1.,0.,0.));
#17861=DIRECTION('ref_axis',(0.,0.,-1.));
#17862=DIRECTION('center_axis',(-1.,0.,0.));
#17863=DIRECTION('ref_axis',(0.,0.999903350347485,0.0139028761007986));
#17864=DIRECTION('center_axis',(-1.,0.,0.));
#17865=DIRECTION('ref_axis',(0.,0.,-1.));
#17866=DIRECTION('center_axis',(-1.,0.,0.));
#17867=DIRECTION('ref_axis',(0.,0.,1.));
#17868=DIRECTION('center_axis',(-1.,0.,0.));
#17869=DIRECTION('ref_axis',(0.,0.707106781186548,0.707106781186547));
#17870=DIRECTION('center_axis',(1.,0.,0.));
#17871=DIRECTION('ref_axis',(0.,0.707106781186548,0.707106781186547));
#17872=DIRECTION('center_axis',(1.,0.,0.));
#17873=DIRECTION('ref_axis',(0.,0.,-1.));
#17874=DIRECTION('center_axis',(-1.,0.,0.));
#17875=DIRECTION('ref_axis',(0.,0.999903350347485,-0.0139028761007986));
#17876=DIRECTION('center_axis',(-1.,0.,0.));
#17877=DIRECTION('ref_axis',(0.,0.,-1.));
#17878=DIRECTION('center_axis',(-1.,0.,0.));
#17879=DIRECTION('ref_axis',(0.,-0.0139028761007986,0.999903350347485));
#17880=DIRECTION('center_axis',(-1.,0.,0.));
#17881=DIRECTION('ref_axis',(0.,0.,-1.));
#17882=DIRECTION('center_axis',(0.,-1.,0.));
#17883=DIRECTION('ref_axis',(-0.707106781186544,0.,0.707106781186551));
#17884=DIRECTION('center_axis',(0.,-1.,0.));
#17885=DIRECTION('ref_axis',(0.,0.,1.));
#17886=DIRECTION('center_axis',(0.,1.,-2.22044604925031E-15));
#17887=DIRECTION('ref_axis',(-1.,0.,0.));
#17888=DIRECTION('',(0.,1.,0.));
#17889=DIRECTION('center_axis',(1.,0.,0.));
#17890=DIRECTION('ref_axis',(0.,0.,-1.));
#17891=DIRECTION('center_axis',(1.,0.,0.));
#17892=DIRECTION('ref_axis',(0.,0.,-1.));
#17893=DIRECTION('center_axis',(-1.,0.,0.));
#17894=DIRECTION('ref_axis',(0.,0.694365074829414,0.719622917128924));
#17895=DIRECTION('center_axis',(1.,0.,0.));
#17896=DIRECTION('ref_axis',(0.,1.,1.58603289232165E-16));
#17897=DIRECTION('',(-1.,0.,0.));
#17898=DIRECTION('center_axis',(1.,0.,0.));
#17899=DIRECTION('ref_axis',(0.,0.939379515438772,0.342879171099701));
#17900=DIRECTION('',(-1.,0.,0.));
#17901=DIRECTION('',(1.,0.,0.));
#17902=DIRECTION('center_axis',(1.,0.,0.));
#17903=DIRECTION('ref_axis',(0.,0.326047170834313,0.945353501284541));
#17904=DIRECTION('',(1.,0.,0.));
#17905=DIRECTION('center_axis',(0.,0.,1.));
#17906=DIRECTION('ref_axis',(0.,-1.,0.));
#17907=DIRECTION('',(0.,-1.,0.));
#17908=DIRECTION('center_axis',(1.,0.,0.));
#17909=DIRECTION('ref_axis',(0.,0.,-1.));
#17910=DIRECTION('center_axis',(0.,-1.,0.));
#17911=DIRECTION('ref_axis',(0.,0.,-1.));
#17912=DIRECTION('center_axis',(-1.55596157992435E-15,0.936610848943197,
-0.35037139957751));
#17913=DIRECTION('ref_axis',(1.,0.,-4.44089209850056E-15));
#17914=DIRECTION('center_axis',(1.,0.,0.));
#17915=DIRECTION('ref_axis',(0.,-0.178029704061997,-0.984025113740294));
#17916=DIRECTION('center_axis',(0.,1.,0.));
#17917=DIRECTION('ref_axis',(0.707106781186538,0.,-0.707106781186557));
#17918=DIRECTION('center_axis',(0.,-1.,2.22044604925031E-15));
#17919=DIRECTION('ref_axis',(0.,-2.22044604925031E-15,-1.));
#17920=DIRECTION('',(0.,1.,0.));
#17921=DIRECTION('center_axis',(1.,0.,0.));
#17922=DIRECTION('ref_axis',(0.,0.,-1.));
#17923=DIRECTION('center_axis',(2.60342613851738E-15,-0.936610848943196,
-0.350371399577514));
#17924=DIRECTION('ref_axis',(0.,0.350371399577514,-0.936610848943196));
#17925=DIRECTION('center_axis',(1.,0.,0.));
#17926=DIRECTION('ref_axis',(0.,0.178029704061997,-0.984025113740294));
#17927=DIRECTION('center_axis',(0.,0.,1.));
#17928=DIRECTION('ref_axis',(1.,0.,0.));
#17929=DIRECTION('center_axis',(1.,0.,0.));
#17930=DIRECTION('ref_axis',(0.,0.999903350347485,0.0139028761007998));
#17931=DIRECTION('center_axis',(0.,0.945990172710257,-0.324195300915386));
#17932=DIRECTION('ref_axis',(0.,-0.324195300915386,-0.945990172710257));
#17933=DIRECTION('center_axis',(0.,0.,1.));
#17934=DIRECTION('ref_axis',(1.,0.,0.));
#17935=DIRECTION('center_axis',(0.,-0.945990172710257,-0.324195300915386));
#17936=DIRECTION('ref_axis',(0.,0.324195300915386,-0.945990172710257));
#17937=DIRECTION('center_axis',(1.,0.,0.));
#17938=DIRECTION('ref_axis',(0.,-0.999903350347485,0.0139028761007998));
#17939=DIRECTION('center_axis',(-1.,0.,0.));
#17940=DIRECTION('ref_axis',(0.,0.,1.));
#17941=DIRECTION('center_axis',(-1.,0.,0.));
#17942=DIRECTION('ref_axis',(0.,-0.707106781186547,0.707106781186548));
#17943=DIRECTION('center_axis',(0.,0.324195300915385,-0.945990172710258));
#17944=DIRECTION('ref_axis',(0.,-0.945990172710258,-0.324195300915385));
#17945=DIRECTION('center_axis',(1.,0.,0.));
#17946=DIRECTION('ref_axis',(0.,0.999903350347485,0.0139028761007986));
#17947=DIRECTION('',(-1.,0.,0.));
#17948=DIRECTION('',(1.,0.,0.));
#17949=DIRECTION('center_axis',(1.,0.,0.));
#17950=DIRECTION('ref_axis',(0.,1.58603289232165E-16,-1.));
#17951=DIRECTION('center_axis',(1.,0.,0.));
#17952=DIRECTION('ref_axis',(0.,0.939379515438772,-0.342879171099701));
#17953=DIRECTION('',(1.,0.,0.));
#17954=DIRECTION('',(1.,0.,0.));
#17955=DIRECTION('center_axis',(0.,0.,-1.));
#17956=DIRECTION('ref_axis',(0.,1.,0.));
#17957=DIRECTION('',(1.,0.,0.));
#17958=DIRECTION('center_axis',(1.,0.,0.));
#17959=DIRECTION('ref_axis',(0.,-1.,-1.58603289232165E-16));
#17960=DIRECTION('',(1.,0.,0.));
#17961=DIRECTION('center_axis',(0.,1.,0.));
#17962=DIRECTION('ref_axis',(0.707106781186541,0.,0.707106781186554));
#17963=DIRECTION('',(0.,-1.,0.));
#17964=DIRECTION('center_axis',(0.,0.,1.));
#17965=DIRECTION('ref_axis',(1.,0.,0.));
#17966=DIRECTION('',(1.,0.,0.));
#17967=DIRECTION('center_axis',(0.,1.,0.));
#17968=DIRECTION('ref_axis',(0.70710678118654,0.,-0.707106781186555));
#17969=DIRECTION('center_axis',(0.,-1.,0.));
#17970=DIRECTION('ref_axis',(0.,0.,-1.));
#17971=DIRECTION('center_axis',(-0.408248290463861,-0.408248290463847,-0.816496580927735));
#17972=DIRECTION('ref_axis',(0.577350269189648,0.577350269189616,-0.577350269189614));
#17973=DIRECTION('center_axis',(-1.,0.,0.));
#17974=DIRECTION('ref_axis',(0.,0.,1.));
#17975=DIRECTION('center_axis',(-1.,0.,0.));
#17976=DIRECTION('ref_axis',(0.,0.707106781186548,0.707106781186548));
#17977=DIRECTION('center_axis',(-1.,0.,0.));
#17978=DIRECTION('ref_axis',(0.,-0.999903350347485,0.0139028761007986));
#17979=DIRECTION('',(-1.,0.,0.));
#17980=DIRECTION('center_axis',(1.,0.,0.));
#17981=DIRECTION('ref_axis',(0.,0.946352857512202,0.323135063214268));
#17982=DIRECTION('',(-1.,0.,0.));
#17983=DIRECTION('center_axis',(-1.,0.,0.));
#17984=DIRECTION('ref_axis',(0.,0.946352857512202,0.323135063214268));
#17985=DIRECTION('center_axis',(-1.,0.,0.));
#17986=DIRECTION('ref_axis',(0.,0.,-1.));
#17987=DIRECTION('',(1.,0.,0.));
#17988=DIRECTION('center_axis',(-1.,0.,0.));
#17989=DIRECTION('ref_axis',(0.,0.,-1.));
#17990=DIRECTION('center_axis',(0.559184554883702,-0.00524477298579031,
-0.829026613526878));
#17991=DIRECTION('ref_axis',(0.828990150486439,-0.00777536702111098,0.559209150554744));
#17992=DIRECTION('center_axis',(1.,0.,0.));
#17993=DIRECTION('ref_axis',(0.,-0.945990172710258,0.324195300915385));
#17994=DIRECTION('center_axis',(0.,0.324195300915381,0.945990172710259));
#17995=DIRECTION('ref_axis',(1.,0.,0.));
#17996=DIRECTION('center_axis',(-4.15938771844182E-15,-0.350371399577514,
0.936610848943196));
#17997=DIRECTION('ref_axis',(0.,0.936610848943196,0.350371399577514));
#17998=DIRECTION('center_axis',(0.,0.,1.));
#17999=DIRECTION('ref_axis',(1.,0.,0.));
#18000=DIRECTION('center_axis',(1.,0.,0.));
#18001=DIRECTION('ref_axis',(0.,0.350371399577514,0.936610848943196));
#18002=DIRECTION('center_axis',(0.,0.936610848943196,-0.350371399577514));
#18003=DIRECTION('ref_axis',(1.,0.,0.));
#18004=DIRECTION('center_axis',(0.,0.945990172710258,0.324195300915385));
#18005=DIRECTION('ref_axis',(0.,0.324195300915385,-0.945990172710258));
#18006=DIRECTION('center_axis',(0.,0.,1.));
#18007=DIRECTION('ref_axis',(1.,0.,0.));
#18008=DIRECTION('center_axis',(1.,0.,0.));
#18009=DIRECTION('ref_axis',(0.,-0.324195300915385,-0.945990172710258));
#18010=DIRECTION('center_axis',(0.,-0.936610848943197,-0.35037139957751));
#18011=DIRECTION('ref_axis',(0.,-0.35037139957751,0.936610848943197));
#18012=DIRECTION('center_axis',(1.,0.,0.));
#18013=DIRECTION('ref_axis',(0.,0.,-1.));
#18014=DIRECTION('center_axis',(0.,1.,-2.22044604925031E-15));
#18015=DIRECTION('ref_axis',(0.,2.22044604925031E-15,1.));
#18016=DIRECTION('center_axis',(0.,-1.,0.));
#18017=DIRECTION('ref_axis',(0.707106781186538,0.,0.707106781186557));
#18018=DIRECTION('center_axis',(0.,1.,-2.22044604925031E-15));
#18019=DIRECTION('ref_axis',(0.,2.22044604925031E-15,1.));
#18020=DIRECTION('center_axis',(1.,0.,0.));
#18021=DIRECTION('ref_axis',(0.,0.,-1.));
#18022=DIRECTION('center_axis',(1.,0.,0.));
#18023=DIRECTION('ref_axis',(0.,-0.999903350347485,-0.0139028761007986));
#18024=DIRECTION('center_axis',(-1.,0.,0.));
#18025=DIRECTION('ref_axis',(0.,-0.999903350347485,-0.0139028761007986));
#18026=DIRECTION('center_axis',(-1.,0.,0.));
#18027=DIRECTION('ref_axis',(0.,-0.707106781186548,-0.707106781186548));
#18028=DIRECTION('center_axis',(-1.,0.,0.));
#18029=DIRECTION('ref_axis',(0.,-0.707106781186548,-0.707106781186547));
#18030=DIRECTION('center_axis',(-1.,0.,0.));
#18031=DIRECTION('ref_axis',(0.,0.999903350347485,-0.0139028761007986));
#18032=DIRECTION('',(-1.,0.,0.));
#18033=DIRECTION('center_axis',(1.,0.,0.));
#18034=DIRECTION('ref_axis',(0.,0.,-1.));
#18035=DIRECTION('center_axis',(1.,0.,0.));
#18036=DIRECTION('ref_axis',(0.,-0.0139028761007986,0.999903350347485));
#18037=DIRECTION('',(1.,0.,0.));
#18038=DIRECTION('center_axis',(-1.,0.,0.));
#18039=DIRECTION('ref_axis',(0.,0.,-1.));
#18040=DIRECTION('center_axis',(-0.559184554883714,0.00524477298580095,
-0.82902661352687));
#18041=DIRECTION('ref_axis',(0.828990150486434,-0.0077753670211287,-0.559209150554751));
#18042=DIRECTION('center_axis',(1.,0.,0.));
#18043=DIRECTION('ref_axis',(0.,0.936610848943196,-0.350371399577514));
#18044=DIRECTION('center_axis',(0.,-0.350371399577516,-0.936610848943195));
#18045=DIRECTION('ref_axis',(1.,0.,0.));
#18046=DIRECTION('center_axis',(1.,0.,0.));
#18047=DIRECTION('ref_axis',(0.,0.,-1.));
#18048=DIRECTION('center_axis',(-1.,0.,0.));
#18049=DIRECTION('ref_axis',(0.,-0.0139028761007986,-0.999903350347485));
#18050=DIRECTION('',(-1.,0.,0.));
#18051=DIRECTION('center_axis',(-1.,0.,0.));
#18052=DIRECTION('ref_axis',(0.,0.,-1.));
#18053=DIRECTION('',(-1.,0.,0.));
#18054=DIRECTION('center_axis',(-1.,0.,0.));
#18055=DIRECTION('ref_axis',(0.,0.,-1.));
#18056=DIRECTION('center_axis',(-1.,0.,0.));
#18057=DIRECTION('ref_axis',(0.,0.,-1.));
#18058=DIRECTION('',(-1.,0.,0.));
#18059=DIRECTION('center_axis',(-1.,0.,0.));
#18060=DIRECTION('ref_axis',(0.,0.,-1.));
#18061=DIRECTION('',(-1.,0.,0.));
#18062=DIRECTION('center_axis',(-1.,0.,0.));
#18063=DIRECTION('ref_axis',(0.,0.,-1.));
#18064=DIRECTION('',(-1.,0.,0.));
#18065=DIRECTION('center_axis',(-1.,0.,0.));
#18066=DIRECTION('ref_axis',(0.,-0.707106781186548,0.707106781186547));
#18067=DIRECTION('center_axis',(1.,0.,0.));
#18068=DIRECTION('ref_axis',(0.,0.,-1.));
#18069=DIRECTION('center_axis',(-1.,0.,0.));
#18070=DIRECTION('ref_axis',(0.,0.706710494065816,0.707502846338621));
#18071=DIRECTION('center_axis',(0.,1.,0.));
#18072=DIRECTION('ref_axis',(1.,0.,0.));
#18073=DIRECTION('center_axis',(0.,1.,0.));
#18074=DIRECTION('ref_axis',(1.,0.,0.));
#18075=DIRECTION('center_axis',(0.,1.,0.));
#18076=DIRECTION('ref_axis',(1.,0.,0.));
#18077=DIRECTION('center_axis',(0.,1.,0.));
#18078=DIRECTION('ref_axis',(1.,0.,0.));
#18079=DIRECTION('center_axis',(0.,1.,0.));
#18080=DIRECTION('ref_axis',(1.,0.,0.));
#18081=DIRECTION('center_axis',(0.,1.,0.));
#18082=DIRECTION('ref_axis',(1.,0.,0.));
#18083=DIRECTION('center_axis',(0.,1.,0.));
#18084=DIRECTION('ref_axis',(1.,0.,0.));
#18085=DIRECTION('center_axis',(0.,1.,0.));
#18086=DIRECTION('ref_axis',(1.,0.,0.));
#18087=DIRECTION('center_axis',(0.,1.,0.));
#18088=DIRECTION('ref_axis',(1.,0.,0.));
#18089=DIRECTION('center_axis',(0.,1.,0.));
#18090=DIRECTION('ref_axis',(1.,0.,0.));
#18091=DIRECTION('center_axis',(1.,0.,0.));
#18092=DIRECTION('ref_axis',(0.,1.,0.));
#18093=DIRECTION('',(1.,0.,0.));
#18094=DIRECTION('center_axis',(1.,0.,0.));
#18095=DIRECTION('ref_axis',(0.,0.,-1.));
#18096=DIRECTION('center_axis',(1.,0.,0.));
#18097=DIRECTION('ref_axis',(0.,0.,-1.));
#18098=DIRECTION('center_axis',(1.,0.,0.));
#18099=DIRECTION('ref_axis',(0.,0.,-1.));
#18100=DIRECTION('center_axis',(1.,0.,0.));
#18101=DIRECTION('ref_axis',(0.,1.,0.));
#18102=DIRECTION('',(1.,0.,0.));
#18103=DIRECTION('center_axis',(1.,0.,0.));
#18104=DIRECTION('ref_axis',(0.,0.,-1.));
#18105=DIRECTION('center_axis',(0.,0.,1.));
#18106=DIRECTION('ref_axis',(1.,0.,0.));
#22626=CARTESIAN_POINT('',(0.,0.,0.));
#22627=CARTESIAN_POINT('Origin',(151.05,0.,0.));
#22628=CARTESIAN_POINT('',(150.8,13.5,-1.65327317884893E-15));
#22629=CARTESIAN_POINT('Origin',(150.8,0.,0.));
#22630=CARTESIAN_POINT('',(151.3,13.,1.59204083889156E-15));
#22631=CARTESIAN_POINT('',(151.05,13.25,-1.62265700887024E-15));
#22632=CARTESIAN_POINT('',(151.3,-13.,-1.59204083889156E-15));
#22633=CARTESIAN_POINT('Origin',(151.3,0.,0.));
#22634=CARTESIAN_POINT('Origin',(151.3,0.,0.));
#22635=CARTESIAN_POINT('Origin',(150.8,13.,0.));
#22636=CARTESIAN_POINT('',(150.8,-16.505,-2.02127954199271E-15));
#22637=CARTESIAN_POINT('Origin',(150.8,0.,0.));
#22638=CARTESIAN_POINT('Origin',(152.8,0.,0.));
#22639=CARTESIAN_POINT('',(154.8,-13.,-1.59204083889156E-15));
#22640=CARTESIAN_POINT('',(152.8,-13.,-1.59204083889156E-15));
#22641=CARTESIAN_POINT('Origin',(154.8,0.,0.));
#22642=CARTESIAN_POINT('Origin',(150.,-79.75,0.));
#22643=CARTESIAN_POINT('',(130.5,-80.,-2.38806125833734E-15));
#22644=CARTESIAN_POINT('Origin',(150.,-80.,0.));
#22645=CARTESIAN_POINT('',(131.,-79.5,2.32682891837997E-15));
#22646=CARTESIAN_POINT('',(130.75,-79.75,-2.35744508835865E-15));
#22647=CARTESIAN_POINT('Origin',(150.,-79.5,0.));
#22648=CARTESIAN_POINT('Origin',(125.8,-80.,-42.));
#22649=CARTESIAN_POINT('',(163.678669277077,-80.,40.));
#22650=CARTESIAN_POINT('',(173.,-80.,30.9027787310304));
#22651=CARTESIAN_POINT('Origin',(167.85,-80.,34.95));
#22652=CARTESIAN_POINT('',(136.321330722923,-80.,40.));
#22653=CARTESIAN_POINT('',(138.1,-80.,40.));
#22654=CARTESIAN_POINT('',(127.8,-80.,30.0530621813219));
#22655=CARTESIAN_POINT('Origin',(132.15,-80.,34.95));
#22656=CARTESIAN_POINT('',(127.8,-80.,-30.0530621813219));
#22657=CARTESIAN_POINT('',(127.8,-80.,-21.));
#22658=CARTESIAN_POINT('',(136.321330722923,-80.,-40.));
#22659=CARTESIAN_POINT('Origin',(132.15,-80.,-34.95));
#22660=CARTESIAN_POINT('',(163.678669277077,-80.,-40.));
#22661=CARTESIAN_POINT('',(138.1,-80.,-40.));
#22662=CARTESIAN_POINT('',(173.,-80.,-30.9027787310304));
#22663=CARTESIAN_POINT('Origin',(167.85,-80.,-34.95));
#22664=CARTESIAN_POINT('',(173.,-80.,-21.));
#22665=CARTESIAN_POINT('Origin',(150.,-80.,0.));
#22666=CARTESIAN_POINT('',(131.0005787145,-35.9988802797138,0.000387228748759416));
#22667=CARTESIAN_POINT('',(131.,-80.,2.32682891837997E-15));
#22668=CARTESIAN_POINT('',(131.,-20.,2.32682891837997E-15));
#22669=CARTESIAN_POINT('Ctrl Pts',(131.,-20.,3.7470027081099E-15));
#22670=CARTESIAN_POINT('Ctrl Pts',(131.,-20.,0.861580403347818));
#22671=CARTESIAN_POINT('Ctrl Pts',(131.062882219654,-20.177547250434,1.72325967716755));
#22672=CARTESIAN_POINT('Ctrl Pts',(131.166407061299,-20.4957587354358,2.50630832645151));
#22673=CARTESIAN_POINT('Ctrl Pts',(131.269931902945,-20.8139702204376,3.28935697573546));
#22674=CARTESIAN_POINT('Ctrl Pts',(131.414099366581,-21.2728459400074,3.99377500048364));
#22675=CARTESIAN_POINT('Ctrl Pts',(131.566890134667,-21.8297157892228,4.60514959406471));
#22676=CARTESIAN_POINT('Ctrl Pts',(131.719680902753,-22.3865856384382,5.21652418764578));
#22677=CARTESIAN_POINT('Ctrl Pts',(131.881094975289,-23.0414496172992,5.73485535005976));
#22678=CARTESIAN_POINT('Ctrl Pts',(132.022932148162,-23.7812715599426,6.14978270902572));
#22679=CARTESIAN_POINT('Ctrl Pts',(132.164769321036,-24.521093502586,6.5647100679917));
#22680=CARTESIAN_POINT('Ctrl Pts',(132.287029594247,-25.3458734090118,6.87623362350966));
#22681=CARTESIAN_POINT('Ctrl Pts',(132.359109453404,-26.218038076651,7.05638957039791));
#22682=CARTESIAN_POINT('Ctrl Pts',(132.407162692842,-26.7994811884105,7.17649353499007));
#22683=CARTESIAN_POINT('Ctrl Pts',(132.432913526034,-27.4019841940426,7.23821189574679));
#22684=CARTESIAN_POINT('Ctrl Pts',(132.432837348447,-28.0029670680466,7.23818290361787));
#22685=CARTESIAN_POINT('Ctrl Pts',(132.432761170859,-28.6039499420506,7.23815391148896));
#22686=CARTESIAN_POINT('Ctrl Pts',(132.406857982492,-29.2034126844264,7.17637756647439));
#22687=CARTESIAN_POINT('Ctrl Pts',(132.358699643159,-29.7840623655322,7.05586397232987));
#22688=CARTESIAN_POINT('Ctrl Pts',(132.310541303825,-30.3647120466379,6.93535037818535));
#22689=CARTESIAN_POINT('Ctrl Pts',(132.240127813526,-30.9265486664736,6.75609953491087));
#22690=CARTESIAN_POINT('Ctrl Pts',(132.156532403699,-31.4546224725911,6.52774573987559));
#22691=CARTESIAN_POINT('Ctrl Pts',(131.989341584043,-32.5107700848262,6.07103814980503));
#22692=CARTESIAN_POINT('Ctrl Pts',(131.769423086272,-33.4318664421888,5.41791875269127));
#22693=CARTESIAN_POINT('Ctrl Pts',(131.5661054454,-34.1731638593317,4.60441612118007));
#22694=CARTESIAN_POINT('Ctrl Pts',(131.464446624964,-34.5438125679032,4.19766480542447));
#22695=CARTESIAN_POINT('Ctrl Pts',(131.366938018753,-34.8695115414198,3.75081768106951));
#22696=CARTESIAN_POINT('Ctrl Pts',(131.282292361583,-35.1407839851041,3.2643108477403));
#22697=CARTESIAN_POINT('Ctrl Pts',(131.155323875828,-35.5476926506305,2.5345505977465));
#22698=CARTESIAN_POINT('Ctrl Pts',(131.057297025417,-35.8321416240344,1.71555600256064));
#22699=CARTESIAN_POINT('Ctrl Pts',(131.019156861914,-35.9439288801667,0.861916886569704));
#22700=CARTESIAN_POINT('Ctrl Pts',(131.006445419458,-35.9811855970535,0.577414055312998));
#22701=CARTESIAN_POINT('Ctrl Pts',(131.000386017092,-35.9992635494311,0.289063010818519));
#22702=CARTESIAN_POINT('Ctrl Pts',(131.000681403705,-35.9986815924753,0.000455940025769347));
#22703=CARTESIAN_POINT('Origin',(150.,-20.,0.));
#22704=CARTESIAN_POINT('',(132.432701479047,-28.,-7.23809523809524));
#22705=CARTESIAN_POINT('Ctrl Pts',(132.432701479047,-28.,-7.23809523809524));
#22706=CARTESIAN_POINT('Ctrl Pts',(132.432701479047,-26.8009816752416,-7.23809523809524));
#22707=CARTESIAN_POINT('Ctrl Pts',(132.321869554036,-25.6008229172718,-6.98274855048125));
#22708=CARTESIAN_POINT('Ctrl Pts',(132.155628452105,-24.545670137385,-6.52703527428346));
#22709=CARTESIAN_POINT('Ctrl Pts',(132.07250790114,-24.0180937474416,-6.29917863618456));
#22710=CARTESIAN_POINT('Ctrl Pts',(131.975535055945,-23.5267688520189,-6.02123035093972));
#22711=CARTESIAN_POINT('Ctrl Pts',(131.874197516921,-23.0724682732237,-5.69922103670885));
#22712=CARTESIAN_POINT('Ctrl Pts',(131.671522438873,-22.1638671156332,-5.05520240824711));
#22713=CARTESIAN_POINT('Ctrl Pts',(131.451388585508,-21.4033632245524,-4.23493966384127));
#22714=CARTESIAN_POINT('Ctrl Pts',(131.282228165024,-20.8608983376114,-3.26382017119042));
#22715=CARTESIAN_POINT('Ctrl Pts',(131.197647954782,-20.5896658941409,-2.778260424865));
#22716=CARTESIAN_POINT('Ctrl Pts',(131.12581110276,-20.3729432017053,-2.25498649147832));
#22717=CARTESIAN_POINT('Ctrl Pts',(131.076399114064,-20.22552672817,-1.7039165396102));
#22718=CARTESIAN_POINT('Ctrl Pts',(131.026987125369,-20.0781102546348,-1.15284658774209));
#22719=CARTESIAN_POINT('Ctrl Pts',(131.,-20.,-0.573980617392535));
#22720=CARTESIAN_POINT('Ctrl Pts',(131.,-20.,3.88578058618805E-15));
#22721=CARTESIAN_POINT('Ctrl Pts',(131.000681403705,-35.9986815924753,0.000455940025769347));
#22722=CARTESIAN_POINT('Ctrl Pts',(131.001272312551,-35.9975174113732,-0.57689070813748));
#22723=CARTESIAN_POINT('Ctrl Pts',(131.027294049206,-35.9216793201183,-1.15526193173957));
#22724=CARTESIAN_POINT('Ctrl Pts',(131.076366966692,-35.7753210194057,-1.70590043958833));
#22725=CARTESIAN_POINT('Ctrl Pts',(131.14997071157,-35.5558003636517,-2.53179501295942));
#22726=CARTESIAN_POINT('Ctrl Pts',(131.27543167792,-35.1776335132831,-3.29530052290559));
#22727=CARTESIAN_POINT('Ctrl Pts',(131.418812458471,-34.6912990154186,-3.96691479885595));
#22728=CARTESIAN_POINT('Ctrl Pts',(131.562193239021,-34.2049645175541,-4.63852907480631));
#22729=CARTESIAN_POINT('Ctrl Pts',(131.723493833771,-33.6104623721938,-5.21825211676085));
#22730=CARTESIAN_POINT('Ctrl Pts',(131.875295509315,-32.9286711143801,-5.70073440851176));
#22731=CARTESIAN_POINT('Ctrl Pts',(132.027097184859,-32.2468798565664,-6.18321670026267));
#22732=CARTESIAN_POINT('Ctrl Pts',(132.169399941196,-31.4777994862994,-6.56845824180994));
#22733=CARTESIAN_POINT('Ctrl Pts',(132.270801014743,-30.6410546041911,-6.83217787626808));
#22734=CARTESIAN_POINT('Ctrl Pts',(132.37220208829,-29.8043097220827,-7.09589751072622));
#22735=CARTESIAN_POINT('Ctrl Pts',(132.432701479047,-28.899900328133,-7.23809523809524));
#22736=CARTESIAN_POINT('Ctrl Pts',(132.432701479047,-28.,-7.23809523809524));
#22737=CARTESIAN_POINT('Origin',(167.85,-79.75,34.95));
#22738=CARTESIAN_POINT('',(172.606870229008,-79.5,31.2117269195014));
#22739=CARTESIAN_POINT('',(173.,-80.,30.9027787310304));
#22740=CARTESIAN_POINT('',(161.8,-79.5,34.95));
#22741=CARTESIAN_POINT('Origin',(167.85,-79.5,34.95));
#22742=CARTESIAN_POINT('',(163.997091469667,-79.5,39.6145038167939));
#22743=CARTESIAN_POINT('Origin',(167.85,-79.5,34.95));
#22744=CARTESIAN_POINT('',(163.997091469667,-79.5,39.6145038167939));
#22745=CARTESIAN_POINT('Ctrl Pts',(164.24404266268,-79.9563089001744,40.4157589290663));
#22746=CARTESIAN_POINT('Ctrl Pts',(164.904763645791,-79.8656939616692,40.8421377709704));
#22747=CARTESIAN_POINT('Ctrl Pts',(165.655411043149,-79.6645622818713,41.125231372512));
#22748=CARTESIAN_POINT('Ctrl Pts',(166.910806630347,-79.4726177418242,41.3575474685077));
#22749=CARTESIAN_POINT('Ctrl Pts',(167.383432581128,-79.4297585902001,41.3983432821216));
#22750=CARTESIAN_POINT('Ctrl Pts',(168.316607594627,-79.4297719859887,41.3983383325715));
#22751=CARTESIAN_POINT('Ctrl Pts',(168.789318171633,-79.4725073961984,41.3576005032552));
#22752=CARTESIAN_POINT('Ctrl Pts',(169.704749159241,-79.6127601152316,41.1880395507574));
#22753=CARTESIAN_POINT('Ctrl Pts',(170.148057043937,-79.7078125846233,41.0590527875963));
#22754=CARTESIAN_POINT('Ctrl Pts',(170.877230469463,-79.8584385725448,40.7532327062643));
#22755=CARTESIAN_POINT('Ctrl Pts',(171.174525863015,-79.9177118275984,40.5973733005739));
#22756=CARTESIAN_POINT('Ctrl Pts',(171.45595733732,-79.9563089001744,40.4157589290663));
#22757=CARTESIAN_POINT('Ctrl Pts',(164.335473025189,-79.8042059334496,40.2771726193775));
#22758=CARTESIAN_POINT('Ctrl Pts',(164.963791192797,-79.7444108109014,40.6856055602962));
#22759=CARTESIAN_POINT('Ctrl Pts',(165.692867363639,-79.5716062994587,40.9777503392776));
#22760=CARTESIAN_POINT('Ctrl Pts',(166.924310432838,-79.4023046236385,41.221432574236));
#22761=CARTESIAN_POINT('Ctrl Pts',(167.390074212417,-79.3638725077551,41.2656132269326));
#22762=CARTESIAN_POINT('Ctrl Pts',(168.309961128106,-79.3638053779168,41.2655672039703));
#22763=CARTESIAN_POINT('Ctrl Pts',(168.775837059739,-79.4023115203605,41.2215445949071));
#22764=CARTESIAN_POINT('Ctrl Pts',(169.673734069797,-79.5257582939345,41.0435505178947));
#22765=CARTESIAN_POINT('Ctrl Pts',(170.106291243202,-79.608279307568,40.9099902338759));
#22766=CARTESIAN_POINT('Ctrl Pts',(170.811431283447,-79.7321249167481,40.6042203974311));
#22767=CARTESIAN_POINT('Ctrl Pts',(171.096853767376,-79.7785267521022,40.4510918365167));
#22768=CARTESIAN_POINT('Ctrl Pts',(171.364526974811,-79.8042059334496,40.2771726193775));
#22769=CARTESIAN_POINT('Ctrl Pts',(164.426903387699,-79.6521029667248,40.1385863096888));
#22770=CARTESIAN_POINT('Ctrl Pts',(165.023200759689,-79.6212831507678,40.5285536883552));
#22771=CARTESIAN_POINT('Ctrl Pts',(165.730469399245,-79.4781267398763,40.8301615232528));
#22772=CARTESIAN_POINT('Ctrl Pts',(166.937783093536,-79.331961481472,41.0852871258424));
#22773=CARTESIAN_POINT('Ctrl Pts',(167.396796517454,-79.2976945980757,41.1327758447739));
#22774=CARTESIAN_POINT('Ctrl Pts',(168.30327953742,-79.2977749929233,41.1328046840522));
#22775=CARTESIAN_POINT('Ctrl Pts',(168.762383358537,-79.3319478756572,41.0853222698221));
#22776=CARTESIAN_POINT('Ctrl Pts',(169.642709147199,-79.4386930097327,40.8991599406581));
#22777=CARTESIAN_POINT('Ctrl Pts',(170.064506615137,-79.5085963881185,40.7608067238982));
#22778=CARTESIAN_POINT('Ctrl Pts',(170.745644981025,-79.6058293970024,40.4552714635503));
#22779=CARTESIAN_POINT('Ctrl Pts',(171.019149702356,-79.6391850754963,40.3047425325162));
#22780=CARTESIAN_POINT('Ctrl Pts',(171.273096612301,-79.6521029667248,40.1385863096887));
#22781=CARTESIAN_POINT('Ctrl Pts',(164.518333750208,-79.5,40.));
#22782=CARTESIAN_POINT('Ctrl Pts',(165.082228306696,-79.5,40.372021477681));
#22783=CARTESIAN_POINT('Ctrl Pts',(165.767925719736,-79.3851707574638,40.6826804900184));
#22784=CARTESIAN_POINT('Ctrl Pts',(166.951286896027,-79.2616483632863,40.9491722315706));
#22785=CARTESIAN_POINT('Ctrl Pts',(167.403438148744,-79.2318085156308,41.000045789585));
#22786=CARTESIAN_POINT('Ctrl Pts',(168.296633070899,-79.2318083848514,41.000033555451));
#22787=CARTESIAN_POINT('Ctrl Pts',(168.748902246643,-79.2617519998194,40.9492663614741));
#22788=CARTESIAN_POINT('Ctrl Pts',(169.611694057755,-79.3516911884357,40.7546709077954));
#22789=CARTESIAN_POINT('Ctrl Pts',(170.022740814401,-79.4090631110633,40.6117441701778));
#22790=CARTESIAN_POINT('Ctrl Pts',(170.679845795009,-79.4795157412057,40.3062591547171));
#22791=CARTESIAN_POINT('Ctrl Pts',(170.941477606716,-79.5,40.1584610684589));
#22792=CARTESIAN_POINT('Ctrl Pts',(171.181666249792,-79.5,40.));
#22793=CARTESIAN_POINT('',(171.181666249792,-79.5,40.));
#22794=CARTESIAN_POINT('',(171.45595733732,-79.9563089001744,40.4157589290663));
#22795=CARTESIAN_POINT('',(171.181666249792,-79.5,40.));
#22796=CARTESIAN_POINT('',(164.24404266268,-79.9563089001744,40.4157589290663));
#22797=CARTESIAN_POINT('Ctrl Pts',(171.45595733732,-79.9563089001744,40.4157589290663));
#22798=CARTESIAN_POINT('Ctrl Pts',(171.174525863015,-79.9177118275984,40.5973733005739));
#22799=CARTESIAN_POINT('Ctrl Pts',(170.877230469463,-79.8584385725448,40.7532327062643));
#22800=CARTESIAN_POINT('Ctrl Pts',(170.148057043937,-79.7078125846233,41.0590527875963));
#22801=CARTESIAN_POINT('Ctrl Pts',(169.704749159241,-79.6127601152316,41.1880395507574));
#22802=CARTESIAN_POINT('Ctrl Pts',(168.789318171633,-79.4725073961984,41.3576005032552));
#22803=CARTESIAN_POINT('Ctrl Pts',(168.316607594627,-79.4297719859887,41.3983383325715));
#22804=CARTESIAN_POINT('Ctrl Pts',(167.383432581128,-79.4297585902001,41.3983432821216));
#22805=CARTESIAN_POINT('Ctrl Pts',(166.910806630347,-79.4726177418242,41.3575474685077));
#22806=CARTESIAN_POINT('Ctrl Pts',(165.655411043149,-79.6645622818713,41.125231372512));
#22807=CARTESIAN_POINT('Ctrl Pts',(164.904763645791,-79.8656939616692,40.8421377709704));
#22808=CARTESIAN_POINT('Ctrl Pts',(164.24404266268,-79.9563089001744,40.4157589290663));
#22809=CARTESIAN_POINT('',(164.518333750208,-79.5,40.));
#22810=CARTESIAN_POINT('',(164.24404266268,-79.9563089001744,40.4157589290663));
#22811=CARTESIAN_POINT('Ctrl Pts',(164.518333750208,-79.5,40.));
#22812=CARTESIAN_POINT('Ctrl Pts',(165.082228306696,-79.5,40.372021477681));
#22813=CARTESIAN_POINT('Ctrl Pts',(165.767925719736,-79.3851707574638,40.6826804900184));
#22814=CARTESIAN_POINT('Ctrl Pts',(166.951286896027,-79.2616483632863,40.9491722315706));
#22815=CARTESIAN_POINT('Ctrl Pts',(167.403438148744,-79.2318085156308,41.000045789585));
#22816=CARTESIAN_POINT('Ctrl Pts',(168.296633070899,-79.2318083848514,41.000033555451));
#22817=CARTESIAN_POINT('Ctrl Pts',(168.748902246643,-79.2617519998194,40.9492663614741));
#22818=CARTESIAN_POINT('Ctrl Pts',(169.611694057755,-79.3516911884357,40.7546709077954));
#22819=CARTESIAN_POINT('Ctrl Pts',(170.022740814401,-79.4090631110633,40.6117441701778));
#22820=CARTESIAN_POINT('Ctrl Pts',(170.679845795009,-79.4795157412057,40.3062591547171));
#22821=CARTESIAN_POINT('Ctrl Pts',(170.941477606716,-79.5,40.1584610684589));
#22822=CARTESIAN_POINT('Ctrl Pts',(171.181666249792,-79.5,40.));
#22823=CARTESIAN_POINT('Ctrl Pts',(163.678669277077,-80.,40.));
#22824=CARTESIAN_POINT('Ctrl Pts',(163.859138387108,-80.,40.1490685828142));
#22825=CARTESIAN_POINT('Ctrl Pts',(164.047413162951,-79.9832757598348,40.2888692728855));
#22826=CARTESIAN_POINT('Ctrl Pts',(164.24404266268,-79.9563089001744,40.4157589290663));
#22827=CARTESIAN_POINT('Ctrl Pts',(163.78481000794,-79.8333333333333,39.8715012722646));
#22828=CARTESIAN_POINT('Ctrl Pts',(163.960687028658,-79.8333333333333,40.0167767613686));
#22829=CARTESIAN_POINT('Ctrl Pts',(164.144230322027,-79.8221838398898,40.152892198886));
#22830=CARTESIAN_POINT('Ctrl Pts',(164.335473025189,-79.8042059334496,40.2771726193775));
#22831=CARTESIAN_POINT('Ctrl Pts',(163.890950738804,-79.6666666666667,39.7430025445293));
#22832=CARTESIAN_POINT('Ctrl Pts',(164.062235670207,-79.6666666666667,39.8844849399229));
#22833=CARTESIAN_POINT('Ctrl Pts',(164.241047481102,-79.6610919199449,40.0169151248864));
#22834=CARTESIAN_POINT('Ctrl Pts',(164.426903387699,-79.6521029667248,40.1385863096888));
#22835=CARTESIAN_POINT('Ctrl Pts',(163.997091469667,-79.5,39.6145038167939));
#22836=CARTESIAN_POINT('Ctrl Pts',(164.163784311757,-79.5,39.7521931184773));
#22837=CARTESIAN_POINT('Ctrl Pts',(164.337864640177,-79.5,39.8809380508869));
#22838=CARTESIAN_POINT('Ctrl Pts',(164.518333750208,-79.5,40.));
#22839=CARTESIAN_POINT('Ctrl Pts',(164.24404266268,-79.9563089001744,40.4157589290663));
#22840=CARTESIAN_POINT('Ctrl Pts',(164.047413162951,-79.9832757598348,40.2888692728855));
#22841=CARTESIAN_POINT('Ctrl Pts',(163.859138387108,-80.,40.1490685828142));
#22842=CARTESIAN_POINT('Ctrl Pts',(163.678669277077,-80.,40.));
#22843=CARTESIAN_POINT('Ctrl Pts',(163.997091469667,-79.5,39.6145038167939));
#22844=CARTESIAN_POINT('Ctrl Pts',(164.163784311757,-79.5,39.7521931184773));
#22845=CARTESIAN_POINT('Ctrl Pts',(164.337864640177,-79.5,39.8809380508869));
#22846=CARTESIAN_POINT('Ctrl Pts',(164.518333750208,-79.5,40.));
#22847=CARTESIAN_POINT('Origin',(167.85,-79.75,34.95));
#22848=CARTESIAN_POINT('',(172.021330722923,-80.,40.));
#22849=CARTESIAN_POINT('',(171.702908530333,-79.5,39.6145038167939));
#22850=CARTESIAN_POINT('',(172.021330722923,-80.,40.));
#22851=CARTESIAN_POINT('',(172.606870229008,-79.5,38.6882730804986));
#22852=CARTESIAN_POINT('Origin',(167.85,-79.5,34.95));
#22853=CARTESIAN_POINT('',(173.,-80.,38.9972212689696));
#22854=CARTESIAN_POINT('',(172.606870229008,-79.5,38.6882730804986));
#22855=CARTESIAN_POINT('Origin',(167.85,-80.,34.95));
#22856=CARTESIAN_POINT('Ctrl Pts',(171.45595733732,-79.9563089001744,40.4157589290663));
#22857=CARTESIAN_POINT('Ctrl Pts',(171.652586837049,-79.9832757598348,40.2888692728855));
#22858=CARTESIAN_POINT('Ctrl Pts',(171.840861612892,-80.,40.1490685828142));
#22859=CARTESIAN_POINT('Ctrl Pts',(172.021330722923,-80.,40.));
#22860=CARTESIAN_POINT('Ctrl Pts',(171.364526974811,-79.8042059334496,40.2771726193775));
#22861=CARTESIAN_POINT('Ctrl Pts',(171.555769677973,-79.8221838398898,40.152892198886));
#22862=CARTESIAN_POINT('Ctrl Pts',(171.739312971342,-79.8333333333333,40.0167767613686));
#22863=CARTESIAN_POINT('Ctrl Pts',(171.91518999206,-79.8333333333333,39.8715012722646));
#22864=CARTESIAN_POINT('Ctrl Pts',(171.273096612301,-79.6521029667248,40.1385863096888));
#22865=CARTESIAN_POINT('Ctrl Pts',(171.458952518898,-79.6610919199449,40.0169151248864));
#22866=CARTESIAN_POINT('Ctrl Pts',(171.637764329793,-79.6666666666667,39.8844849399229));
#22867=CARTESIAN_POINT('Ctrl Pts',(171.809049261196,-79.6666666666667,39.7430025445293));
#22868=CARTESIAN_POINT('Ctrl Pts',(171.181666249792,-79.5,40.));
#22869=CARTESIAN_POINT('Ctrl Pts',(171.362135359823,-79.5,39.8809380508869));
#22870=CARTESIAN_POINT('Ctrl Pts',(171.536215688243,-79.5,39.7521931184773));
#22871=CARTESIAN_POINT('Ctrl Pts',(171.702908530333,-79.5,39.6145038167939));
#22872=CARTESIAN_POINT('Ctrl Pts',(172.021330722923,-80.,40.));
#22873=CARTESIAN_POINT('Ctrl Pts',(171.840861612892,-80.,40.1490685828142));
#22874=CARTESIAN_POINT('Ctrl Pts',(171.652586837049,-79.9832757598348,40.2888692728855));
#22875=CARTESIAN_POINT('Ctrl Pts',(171.45595733732,-79.9563089001744,40.4157589290663));
#22876=CARTESIAN_POINT('Ctrl Pts',(171.181666249792,-79.5,40.));
#22877=CARTESIAN_POINT('Ctrl Pts',(171.362135359823,-79.5,39.8809380508869));
#22878=CARTESIAN_POINT('Ctrl Pts',(171.536215688243,-79.5,39.7521931184773));
#22879=CARTESIAN_POINT('Ctrl Pts',(171.702908530333,-79.5,39.6145038167939));
#22880=CARTESIAN_POINT('Ctrl Pts',(173.423859320912,-79.9545698442563,38.3862048013962));
#22881=CARTESIAN_POINT('Ctrl Pts',(173.637590761883,-79.9082209948182,38.031453352118));
#22882=CARTESIAN_POINT('Ctrl Pts',(174.161182840155,-79.6758255748561,36.8926040756434));
#22883=CARTESIAN_POINT('Ctrl Pts',(174.450714954638,-79.3629293846521,34.7340491444972));
#22884=CARTESIAN_POINT('Ctrl Pts',(174.12628339776,-79.6894007116804,33.0353820059301));
#22885=CARTESIAN_POINT('Ctrl Pts',(173.695468913621,-79.8788938435096,32.0051494847125));
#22886=CARTESIAN_POINT('Ctrl Pts',(173.568618196577,-79.9231780784845,31.7540659828401));
#22887=CARTESIAN_POINT('Ctrl Pts',(173.423859320912,-79.9545698442563,31.5137951986038));
#22888=CARTESIAN_POINT('Ctrl Pts',(173.282572880608,-79.8030465628375,38.2991037253566));
#22889=CARTESIAN_POINT('Ctrl Pts',(173.486921961723,-79.7720130814336,37.9606510628592));
#22890=CARTESIAN_POINT('Ctrl Pts',(174.009109978221,-79.5855452720181,36.8638359099341));
#22891=CARTESIAN_POINT('Ctrl Pts',(174.323939769628,-79.3038896735438,34.736501924795));
#22892=CARTESIAN_POINT('Ctrl Pts',(173.974333222952,-79.596158192733,33.0659783751474));
#22893=CARTESIAN_POINT('Ctrl Pts',(173.545800607626,-79.7480856679502,32.071313990426));
#22894=CARTESIAN_POINT('Ctrl Pts',(173.421574808057,-79.7822166975021,31.8298143240271));
#22895=CARTESIAN_POINT('Ctrl Pts',(173.282572880608,-79.8030465628375,31.6008962746433));
#22896=CARTESIAN_POINT('Ctrl Pts',(173.141286440304,-79.6515232814188,38.2120026493171));
#22897=CARTESIAN_POINT('Ctrl Pts',(173.338735235185,-79.6362079133846,37.8906417628064));
#22898=CARTESIAN_POINT('Ctrl Pts',(173.855318098134,-79.494523230808,36.8350822467445));
#22899=CARTESIAN_POINT('Ctrl Pts',(174.198332784239,-79.2449563760689,34.739214009455));
#22900=CARTESIAN_POINT('Ctrl Pts',(173.821676532788,-79.5015464237554,33.0986369664091));
#22901=CARTESIAN_POINT('Ctrl Pts',(173.396335027929,-79.6176373358252,32.1369290213944));
#22902=CARTESIAN_POINT('Ctrl Pts',(173.27441952729,-79.6409613809824,31.9059666056146));
#22903=CARTESIAN_POINT('Ctrl Pts',(173.141286440304,-79.6515232814188,31.6879973506829));
#22904=CARTESIAN_POINT('Ctrl Pts',(173.,-79.5,38.1249015732775));
#22905=CARTESIAN_POINT('Ctrl Pts',(173.188066435025,-79.5,37.8198394735476));
#22906=CARTESIAN_POINT('Ctrl Pts',(173.703245236199,-79.4042429279699,36.8063140810353));
#22907=CARTESIAN_POINT('Ctrl Pts',(174.071557599229,-79.1859166649607,34.7416667897528));
#22908=CARTESIAN_POINT('Ctrl Pts',(173.669726357979,-79.408303904808,33.1292333356263));
#22909=CARTESIAN_POINT('Ctrl Pts',(173.246666721935,-79.4868291602657,32.2030935271079));
#22910=CARTESIAN_POINT('Ctrl Pts',(173.12737613877,-79.5,31.9817149468016));
#22911=CARTESIAN_POINT('Ctrl Pts',(173.,-79.5,31.7750984267225));
#22912=CARTESIAN_POINT('',(173.,-79.5,31.7750984267225));
#22913=CARTESIAN_POINT('',(173.423859320912,-79.9545698442563,31.5137951986038));
#22914=CARTESIAN_POINT('',(173.,-79.5,31.7750984267225));
#22915=CARTESIAN_POINT('',(173.423859320912,-79.9545698442563,38.3862048013962));
#22916=CARTESIAN_POINT('Ctrl Pts',(173.423859320912,-79.9545698442563,31.5137951986038));
#22917=CARTESIAN_POINT('Ctrl Pts',(173.568618196577,-79.9231780784845,31.7540659828401));
#22918=CARTESIAN_POINT('Ctrl Pts',(173.695468913621,-79.8788938435096,32.0051494847125));
#22919=CARTESIAN_POINT('Ctrl Pts',(174.12628339776,-79.6894007116804,33.0353820059301));
#22920=CARTESIAN_POINT('Ctrl Pts',(174.450714954638,-79.3629293846521,34.7340491444972));
#22921=CARTESIAN_POINT('Ctrl Pts',(174.161182840155,-79.6758255748561,36.8926040756434));
#22922=CARTESIAN_POINT('Ctrl Pts',(173.637590761883,-79.9082209948182,38.031453352118));
#22923=CARTESIAN_POINT('Ctrl Pts',(173.423859320912,-79.9545698442563,38.3862048013962));
#22924=CARTESIAN_POINT('',(173.,-79.5,38.1249015732775));
#22925=CARTESIAN_POINT('',(173.423859320912,-79.9545698442563,38.3862048013962));
#22926=CARTESIAN_POINT('Ctrl Pts',(173.,-79.5,38.1249015732775));
#22927=CARTESIAN_POINT('Ctrl Pts',(173.188066435025,-79.5,37.8198394735476));
#22928=CARTESIAN_POINT('Ctrl Pts',(173.703245236199,-79.4042429279699,36.8063140810353));
#22929=CARTESIAN_POINT('Ctrl Pts',(174.071557599229,-79.1859166649607,34.7416667897528));
#22930=CARTESIAN_POINT('Ctrl Pts',(173.669726357979,-79.408303904808,33.1292333356263));
#22931=CARTESIAN_POINT('Ctrl Pts',(173.246666721935,-79.4868291602657,32.2030935271079));
#22932=CARTESIAN_POINT('Ctrl Pts',(173.12737613877,-79.5,31.9817149468016));
#22933=CARTESIAN_POINT('Ctrl Pts',(173.,-79.5,31.7750984267225));
#22934=CARTESIAN_POINT('Ctrl Pts',(173.,-80.,38.9972212689696));
#22935=CARTESIAN_POINT('Ctrl Pts',(173.153269804814,-80.,38.8021888152602));
#22936=CARTESIAN_POINT('Ctrl Pts',(173.295884311895,-79.9823219353749,38.5986177234898));
#22937=CARTESIAN_POINT('Ctrl Pts',(173.423859320912,-79.9545698442563,38.3862048013962));
#22938=CARTESIAN_POINT('Ctrl Pts',(172.868956743003,-79.8333333333333,38.8942385394793));
#22939=CARTESIAN_POINT('Ctrl Pts',(173.018326552783,-79.8333333333333,38.7041687436251));
#22940=CARTESIAN_POINT('Ctrl Pts',(173.157177965592,-79.8215479569166,38.5057231579888));
#22941=CARTESIAN_POINT('Ctrl Pts',(173.282572880608,-79.8030465628376,38.2991037253566));
#22942=CARTESIAN_POINT('Ctrl Pts',(172.737913486005,-79.6666666666667,38.791255809989));
#22943=CARTESIAN_POINT('Ctrl Pts',(172.883383300752,-79.6666666666667,38.6061486719899));
#22944=CARTESIAN_POINT('Ctrl Pts',(173.018471619289,-79.6607739784583,38.4128285924879));
#22945=CARTESIAN_POINT('Ctrl Pts',(173.141286440304,-79.6515232814188,38.2120026493171));
#22946=CARTESIAN_POINT('Ctrl Pts',(172.606870229008,-79.5,38.6882730804986));
#22947=CARTESIAN_POINT('Ctrl Pts',(172.748440048721,-79.5,38.5081286003548));
#22948=CARTESIAN_POINT('Ctrl Pts',(172.879765272986,-79.5,38.3199340269869));
#22949=CARTESIAN_POINT('Ctrl Pts',(173.,-79.5,38.1249015732775));
#22950=CARTESIAN_POINT('Ctrl Pts',(173.423859320912,-79.9545698442563,38.3862048013962));
#22951=CARTESIAN_POINT('Ctrl Pts',(173.295884311895,-79.9823219353749,38.5986177234898));
#22952=CARTESIAN_POINT('Ctrl Pts',(173.153269804814,-80.,38.8021888152602));
#22953=CARTESIAN_POINT('Ctrl Pts',(173.,-80.,38.9972212689696));
#22954=CARTESIAN_POINT('Ctrl Pts',(172.606870229008,-79.5,38.6882730804986));
#22955=CARTESIAN_POINT('Ctrl Pts',(172.748440048721,-79.5,38.5081286003548));
#22956=CARTESIAN_POINT('Ctrl Pts',(172.879765272986,-79.5,38.3199340269869));
#22957=CARTESIAN_POINT('Ctrl Pts',(173.,-79.5,38.1249015732775));
#22958=CARTESIAN_POINT('Ctrl Pts',(173.423859320912,-79.9545698442563,31.5137951986038));
#22959=CARTESIAN_POINT('Ctrl Pts',(173.295884311895,-79.9823219353749,31.3013822765102));
#22960=CARTESIAN_POINT('Ctrl Pts',(173.153269804814,-80.,31.0978111847398));
#22961=CARTESIAN_POINT('Ctrl Pts',(173.,-80.,30.9027787310303));
#22962=CARTESIAN_POINT('Ctrl Pts',(173.282572880608,-79.8030465628376,31.6008962746434));
#22963=CARTESIAN_POINT('Ctrl Pts',(173.157177965592,-79.8215479569166,31.3942768420111));
#22964=CARTESIAN_POINT('Ctrl Pts',(173.018326552783,-79.8333333333333,31.1958312563749));
#22965=CARTESIAN_POINT('Ctrl Pts',(172.868956743003,-79.8333333333333,31.0057614605207));
#22966=CARTESIAN_POINT('Ctrl Pts',(173.141286440304,-79.6515232814188,31.6879973506829));
#22967=CARTESIAN_POINT('Ctrl Pts',(173.018471619289,-79.6607739784583,31.4871714075121));
#22968=CARTESIAN_POINT('Ctrl Pts',(172.883383300752,-79.6666666666667,31.29385132801));
#22969=CARTESIAN_POINT('Ctrl Pts',(172.737913486005,-79.6666666666667,31.108744190011));
#22970=CARTESIAN_POINT('Ctrl Pts',(173.,-79.5,31.7750984267225));
#22971=CARTESIAN_POINT('Ctrl Pts',(172.879765272986,-79.5,31.580065973013));
#22972=CARTESIAN_POINT('Ctrl Pts',(172.748440048721,-79.5,31.3918713996451));
#22973=CARTESIAN_POINT('Ctrl Pts',(172.606870229008,-79.5,31.2117269195013));
#22974=CARTESIAN_POINT('Ctrl Pts',(173.,-80.,30.9027787310303));
#22975=CARTESIAN_POINT('Ctrl Pts',(173.153269804814,-80.,31.0978111847398));
#22976=CARTESIAN_POINT('Ctrl Pts',(173.295884311895,-79.9823219353749,31.3013822765102));
#22977=CARTESIAN_POINT('Ctrl Pts',(173.423859320912,-79.9545698442563,31.5137951986038));
#22978=CARTESIAN_POINT('Ctrl Pts',(173.,-79.5,31.7750984267225));
#22979=CARTESIAN_POINT('Ctrl Pts',(172.879765272986,-79.5,31.580065973013));
#22980=CARTESIAN_POINT('Ctrl Pts',(172.748440048721,-79.5,31.3918713996451));
#22981=CARTESIAN_POINT('Ctrl Pts',(172.606870229008,-79.5,31.2117269195013));
#22982=CARTESIAN_POINT('Origin',(125.8,-80.,-42.));
#22983=CARTESIAN_POINT('',(173.,-80.,40.));
#22984=CARTESIAN_POINT('',(173.,-80.,-21.));
#22985=CARTESIAN_POINT('',(138.1,-80.,40.));
#22986=CARTESIAN_POINT('Origin',(173.,-78.,-21.));
#22987=CARTESIAN_POINT('',(173.423859320912,-79.9545698442563,-31.5137951986038));
#22988=CARTESIAN_POINT('Ctrl Pts',(173.423859320912,-79.9545698442563,-31.5137951986038));
#22989=CARTESIAN_POINT('Ctrl Pts',(173.295884311895,-79.9823219353749,-31.3013822765102));
#22990=CARTESIAN_POINT('Ctrl Pts',(173.153269804814,-80.,-31.0978111847398));
#22991=CARTESIAN_POINT('Ctrl Pts',(173.,-80.,-30.9027787310304));
#22992=CARTESIAN_POINT('',(173.423859320912,-79.9545698442563,-38.3862048013962));
#22993=CARTESIAN_POINT('Ctrl Pts',(173.423859320912,-79.9545698442563,-38.3862048013962));
#22994=CARTESIAN_POINT('Ctrl Pts',(173.943894783993,-79.8417972672725,-37.5230499311273));
#22995=CARTESIAN_POINT('Ctrl Pts',(174.412080939248,-79.4069780593559,-35.8280882420133));
#22996=CARTESIAN_POINT('Ctrl Pts',(174.252601993115,-79.5822812285807,-33.3779001916364));
#22997=CARTESIAN_POINT('Ctrl Pts',(173.770549629633,-79.8793881262671,-32.089231778783));
#22998=CARTESIAN_POINT('Ctrl Pts',(173.423859320912,-79.9545698442563,-31.5137951986038));
#22999=CARTESIAN_POINT('',(173.,-80.,-38.9972212689696));
#23000=CARTESIAN_POINT('Ctrl Pts',(173.,-80.,-38.9972212689696));
#23001=CARTESIAN_POINT('Ctrl Pts',(173.153269804814,-80.,-38.8021888152602));
#23002=CARTESIAN_POINT('Ctrl Pts',(173.295884311895,-79.9823219353749,-38.5986177234898));
#23003=CARTESIAN_POINT('Ctrl Pts',(173.423859320912,-79.9545698442563,-38.3862048013962));
#23004=CARTESIAN_POINT('',(173.,-80.,-40.));
#23005=CARTESIAN_POINT('',(173.,-80.,-21.));
#23006=CARTESIAN_POINT('',(175.,-78.,-40.));
#23007=CARTESIAN_POINT('Origin',(173.,-78.,-40.));
#23008=CARTESIAN_POINT('',(175.,-78.,40.));
#23009=CARTESIAN_POINT('',(175.,-78.,-21.));
#23010=CARTESIAN_POINT('Origin',(173.,-78.,40.));
#23011=CARTESIAN_POINT('Origin',(167.85,-80.,34.95));
#23012=CARTESIAN_POINT('',(161.8,-62.,34.95));
#23013=CARTESIAN_POINT('',(161.8,-80.,34.95));
#23014=CARTESIAN_POINT('Origin',(167.85,-62.,34.95));
#23015=CARTESIAN_POINT('Origin',(132.15,-79.75,34.95));
#23016=CARTESIAN_POINT('',(136.002908530333,-79.5,39.6145038167939));
#23017=CARTESIAN_POINT('',(136.321330722923,-80.,40.));
#23018=CARTESIAN_POINT('',(128.132061068702,-79.5,30.4268742285492));
#23019=CARTESIAN_POINT('Origin',(132.15,-79.5,34.95));
#23020=CARTESIAN_POINT('',(128.132061068702,-79.5,30.4268742285492));
#23021=CARTESIAN_POINT('Ctrl Pts',(127.441253216958,-79.9675621326039,30.3984720929491));
#23022=CARTESIAN_POINT('Ctrl Pts',(127.010949285711,-79.8891045588851,30.8509787580965));
#23023=CARTESIAN_POINT('Ctrl Pts',(126.359829906089,-79.505173748897,31.8485409396476));
#23024=CARTESIAN_POINT('Ctrl Pts',(125.980839327581,-78.8803260190864,33.2693000226215));
#23025=CARTESIAN_POINT('Ctrl Pts',(125.89482908045,-78.6140190998926,34.4028408191624));
#23026=CARTESIAN_POINT('Ctrl Pts',(125.888503697217,-78.5931683273057,35.1083194295444));
#23027=CARTESIAN_POINT('Ctrl Pts',(125.923956953429,-78.7098702272533,36.1351458834427));
#23028=CARTESIAN_POINT('Ctrl Pts',(126.144405087748,-79.2432835801445,37.4747106349361));
#23029=CARTESIAN_POINT('Ctrl Pts',(126.667036945875,-79.6927084333072,38.5244922950161));
#23030=CARTESIAN_POINT('Ctrl Pts',(127.151416515836,-79.8969423996626,39.177231226563));
#23031=CARTESIAN_POINT('Ctrl Pts',(127.289669164758,-79.9399237215032,39.3421224520473));
#23032=CARTESIAN_POINT('Ctrl Pts',(127.441253216958,-79.9675621326039,39.5015279070509));
#23033=CARTESIAN_POINT('Ctrl Pts',(127.560835477972,-79.8117080884026,30.5140616591908));
#23034=CARTESIAN_POINT('Ctrl Pts',(127.154974662842,-79.7602628230784,30.9380771467348));
#23035=CARTESIAN_POINT('Ctrl Pts',(126.505755059624,-79.4351002932416,31.8909513534322));
#23036=CARTESIAN_POINT('Ctrl Pts',(126.07741695658,-78.8533419955133,33.2824824759202));
#23037=CARTESIAN_POINT('Ctrl Pts',(125.965427423976,-78.5983678503514,34.4062520213906));
#23038=CARTESIAN_POINT('Ctrl Pts',(125.956887081345,-78.5784245844343,35.1073387341663));
#23039=CARTESIAN_POINT('Ctrl Pts',(126.004467234684,-78.6903079144387,36.1272907384385));
#23040=CARTESIAN_POINT('Ctrl Pts',(126.273693479842,-79.1962424615693,37.4481542849529));
#23041=CARTESIAN_POINT('Ctrl Pts',(126.813063908194,-79.5941607689053,38.4609627973759));
#23042=CARTESIAN_POINT('Ctrl Pts',(127.285673917206,-79.7601242813882,39.0809512291426));
#23043=CARTESIAN_POINT('Ctrl Pts',(127.417963408171,-79.7933724658796,39.2365237097017));
#23044=CARTESIAN_POINT('Ctrl Pts',(127.560835477972,-79.8117080884026,39.3859383408092));
#23045=CARTESIAN_POINT('Ctrl Pts',(127.680417738986,-79.6558540442013,30.6296512254325));
#23046=CARTESIAN_POINT('Ctrl Pts',(127.300909005748,-79.6288417358066,31.0254726966277));
#23047=CARTESIAN_POINT('Ctrl Pts',(126.651492608816,-79.3655282549205,31.9333992201126));
#23048=CARTESIAN_POINT('Ctrl Pts',(126.175369589829,-78.8255363022201,33.2958500568041));
#23049=CARTESIAN_POINT('Ctrl Pts',(126.037188345547,-78.5824120899783,34.4097905529733));
#23050=CARTESIAN_POINT('Ctrl Pts',(126.026621490162,-78.5632074329542,35.1065199042014));
#23051=CARTESIAN_POINT('Ctrl Pts',(126.085386653903,-78.6703247029404,36.1193807396987));
#23052=CARTESIAN_POINT('Ctrl Pts',(126.402558439516,-79.1492775981534,37.4214590655734));
#23053=CARTESIAN_POINT('Ctrl Pts',(126.96087633252,-79.4942962941443,38.3976021536797));
#23054=CARTESIAN_POINT('Ctrl Pts',(127.419433872465,-79.6236341102445,38.9846162323084));
#23055=CARTESIAN_POINT('Ctrl Pts',(127.546626060281,-79.6465512556236,39.1309577515217));
#23056=CARTESIAN_POINT('Ctrl Pts',(127.680417738986,-79.6558540442013,39.2703487745675));
#23057=CARTESIAN_POINT('Ctrl Pts',(127.8,-79.5,30.7452407916743));
#23058=CARTESIAN_POINT('Ctrl Pts',(127.444934382879,-79.5,31.1125710852661));
#23059=CARTESIAN_POINT('Ctrl Pts',(126.79741776235,-79.2954547992651,31.9758096338973));
#23060=CARTESIAN_POINT('Ctrl Pts',(126.271947218828,-78.798552278647,33.3090325101028));
#23061=CARTESIAN_POINT('Ctrl Pts',(126.107786689073,-78.5667608404371,34.4132017552016));
#23062=CARTESIAN_POINT('Ctrl Pts',(126.09500487429,-78.5484636900828,35.1055392088234));
#23063=CARTESIAN_POINT('Ctrl Pts',(126.165896935158,-78.6507623901258,36.1115255946945));
#23064=CARTESIAN_POINT('Ctrl Pts',(126.53184683161,-79.1022364795782,37.3949027155902));
#23065=CARTESIAN_POINT('Ctrl Pts',(127.106903294839,-79.3957486297424,38.3340726560396));
#23066=CARTESIAN_POINT('Ctrl Pts',(127.553691273835,-79.48681599197,38.8883362348881));
#23067=CARTESIAN_POINT('Ctrl Pts',(127.674920303693,-79.5,39.0253590091761));
#23068=CARTESIAN_POINT('Ctrl Pts',(127.8,-79.5,39.1547592083257));
#23069=CARTESIAN_POINT('',(127.8,-79.5,39.1547592083257));
#23070=CARTESIAN_POINT('',(127.441253216958,-79.9675621326039,39.5015279070509));
#23071=CARTESIAN_POINT('',(127.8,-79.5,39.1547592083257));
#23072=CARTESIAN_POINT('',(127.441253216958,-79.9675621326039,30.3984720929491));
#23073=CARTESIAN_POINT('Ctrl Pts',(127.441253216958,-79.9675621326039,39.5015279070509));
#23074=CARTESIAN_POINT('Ctrl Pts',(127.289669164758,-79.9399237215032,39.3421224520473));
#23075=CARTESIAN_POINT('Ctrl Pts',(127.151416515836,-79.8969423996626,39.177231226563));
#23076=CARTESIAN_POINT('Ctrl Pts',(126.667036945875,-79.6927084333072,38.5244922950161));
#23077=CARTESIAN_POINT('Ctrl Pts',(126.144405087748,-79.2432835801445,37.4747106349361));
#23078=CARTESIAN_POINT('Ctrl Pts',(125.923956953429,-78.7098702272533,36.1351458834427));
#23079=CARTESIAN_POINT('Ctrl Pts',(125.888503697217,-78.5931683273057,35.1083194295444));
#23080=CARTESIAN_POINT('Ctrl Pts',(125.89482908045,-78.6140190998926,34.4028408191624));
#23081=CARTESIAN_POINT('Ctrl Pts',(125.980839327581,-78.8803260190864,33.2693000226215));
#23082=CARTESIAN_POINT('Ctrl Pts',(126.359829906089,-79.505173748897,31.8485409396476));
#23083=CARTESIAN_POINT('Ctrl Pts',(127.010949285711,-79.8891045588851,30.8509787580965));
#23084=CARTESIAN_POINT('Ctrl Pts',(127.441253216958,-79.9675621326039,30.3984720929491));
#23085=CARTESIAN_POINT('',(127.8,-79.5,30.7452407916743));
#23086=CARTESIAN_POINT('',(127.441253216958,-79.9675621326039,30.3984720929491));
#23087=CARTESIAN_POINT('',(126.100434613226,-78.555599219619,34.950001316873));
#23088=CARTESIAN_POINT('Ctrl Pts',(127.8,-79.5,30.7452407916743));
#23089=CARTESIAN_POINT('Ctrl Pts',(127.444934382879,-79.5,31.1125710852661));
#23090=CARTESIAN_POINT('Ctrl Pts',(126.79741776235,-79.2954547992651,31.9758096338973));
#23091=CARTESIAN_POINT('Ctrl Pts',(126.271947218828,-78.798552278647,33.3090325101028));
#23092=CARTESIAN_POINT('Ctrl Pts',(126.114775132993,-78.5766283857558,34.36619639491));
#23093=CARTESIAN_POINT('Ctrl Pts',(126.100704378151,-78.5566089729325,34.829752350636));
#23094=CARTESIAN_POINT('Ctrl Pts',(126.10063677192,-78.556545254597,34.9500019294114));
#23095=CARTESIAN_POINT('Ctrl Pts',(126.10063677192,-78.556545254597,34.9500019294114));
#23096=CARTESIAN_POINT('Ctrl Pts',(126.100608073589,-78.5565182066481,35.0010469611779));
#23097=CARTESIAN_POINT('Ctrl Pts',(126.103299297984,-78.5604327138508,35.2232403619927));
#23098=CARTESIAN_POINT('Ctrl Pts',(126.165896935158,-78.6507623901258,36.1115255946945));
#23099=CARTESIAN_POINT('Ctrl Pts',(126.53184683161,-79.1022364795782,37.3949027155902));
#23100=CARTESIAN_POINT('Ctrl Pts',(127.106903294839,-79.3957486297424,38.3340726560396));
#23101=CARTESIAN_POINT('Ctrl Pts',(127.553691273835,-79.48681599197,38.8883362348881));
#23102=CARTESIAN_POINT('Ctrl Pts',(127.674920303693,-79.5,39.0253590091761));
#23103=CARTESIAN_POINT('Ctrl Pts',(127.8,-79.5,39.1547592083257));
#23104=CARTESIAN_POINT('Ctrl Pts',(127.8,-80.,30.0530621813219));
#23105=CARTESIAN_POINT('Ctrl Pts',(127.675853962606,-80.,30.1633423773672));
#23106=CARTESIAN_POINT('Ctrl Pts',(127.555667352303,-79.9884233304841,30.2781544405375));
#23107=CARTESIAN_POINT('Ctrl Pts',(127.441253216958,-79.9675621326039,30.3984720929491));
#23108=CARTESIAN_POINT('Ctrl Pts',(127.910687022901,-79.8333333333333,30.1776661970643));
#23109=CARTESIAN_POINT('Ctrl Pts',(127.789699917756,-79.8333333333333,30.285140281251));
#23110=CARTESIAN_POINT('Ctrl Pts',(127.672644263207,-79.8256155536561,30.397089825568));
#23111=CARTESIAN_POINT('Ctrl Pts',(127.560835477972,-79.8117080884026,30.5140616591908));
#23112=CARTESIAN_POINT('Ctrl Pts',(128.021374045802,-79.6666666666667,30.3022702128068));
#23113=CARTESIAN_POINT('Ctrl Pts',(127.903545872906,-79.6666666666667,30.4069381851348));
#23114=CARTESIAN_POINT('Ctrl Pts',(127.789621174111,-79.662807776828,30.5160252105985));
#23115=CARTESIAN_POINT('Ctrl Pts',(127.680417738986,-79.6558540442013,30.6296512254325));
#23116=CARTESIAN_POINT('Ctrl Pts',(128.132061068702,-79.5,30.4268742285492));
#23117=CARTESIAN_POINT('Ctrl Pts',(128.017391828056,-79.5,30.5287360890186));
#23118=CARTESIAN_POINT('Ctrl Pts',(127.906598085016,-79.5,30.634960595629));
#23119=CARTESIAN_POINT('Ctrl Pts',(127.8,-79.5,30.7452407916743));
#23120=CARTESIAN_POINT('Ctrl Pts',(127.441253216958,-79.9675621326039,30.3984720929491));
#23121=CARTESIAN_POINT('Ctrl Pts',(127.555667352303,-79.9884233304841,30.2781544405375));
#23122=CARTESIAN_POINT('Ctrl Pts',(127.675853962606,-80.,30.1633423773672));
#23123=CARTESIAN_POINT('Ctrl Pts',(127.8,-80.,30.0530621813219));
#23124=CARTESIAN_POINT('Ctrl Pts',(128.132061068702,-79.5,30.4268742285492));
#23125=CARTESIAN_POINT('Ctrl Pts',(128.017391828056,-79.5,30.5287360890186));
#23126=CARTESIAN_POINT('Ctrl Pts',(127.906598085016,-79.5,30.634960595629));
#23127=CARTESIAN_POINT('Ctrl Pts',(127.8,-79.5,30.7452407916743));
#23128=CARTESIAN_POINT('Origin',(132.15,-79.75,34.95));
#23129=CARTESIAN_POINT('',(127.8,-80.,39.8469378186781));
#23130=CARTESIAN_POINT('',(128.132061068702,-79.5,39.4731257714508));
#23131=CARTESIAN_POINT('',(127.8,-80.,39.8469378186781));
#23132=CARTESIAN_POINT('',(128.297091469667,-79.5,39.6145038167939));
#23133=CARTESIAN_POINT('Origin',(132.15,-79.5,34.95));
#23134=CARTESIAN_POINT('',(127.978669277077,-80.,40.));
#23135=CARTESIAN_POINT('',(128.297091469667,-79.5,39.6145038167939));
#23136=CARTESIAN_POINT('Origin',(132.15,-80.,34.95));
#23137=CARTESIAN_POINT('Ctrl Pts',(127.441253216958,-79.9675621326039,39.5015279070509));
#23138=CARTESIAN_POINT('Ctrl Pts',(127.555667352303,-79.9884233304841,39.6218455594625));
#23139=CARTESIAN_POINT('Ctrl Pts',(127.675853962606,-80.,39.7366576226328));
#23140=CARTESIAN_POINT('Ctrl Pts',(127.8,-80.,39.8469378186781));
#23141=CARTESIAN_POINT('Ctrl Pts',(127.560835477972,-79.8117080884026,39.3859383408092));
#23142=CARTESIAN_POINT('Ctrl Pts',(127.672644263207,-79.8256155536561,39.502910174432));
#23143=CARTESIAN_POINT('Ctrl Pts',(127.789699917756,-79.8333333333333,39.614859718749));
#23144=CARTESIAN_POINT('Ctrl Pts',(127.910687022901,-79.8333333333333,39.7223338029357));
#23145=CARTESIAN_POINT('Ctrl Pts',(127.680417738986,-79.6558540442013,39.2703487745675));
#23146=CARTESIAN_POINT('Ctrl Pts',(127.789621174111,-79.662807776828,39.3839747894015));
#23147=CARTESIAN_POINT('Ctrl Pts',(127.903545872906,-79.6666666666667,39.4930618148652));
#23148=CARTESIAN_POINT('Ctrl Pts',(128.021374045802,-79.6666666666667,39.5977297871932));
#23149=CARTESIAN_POINT('Ctrl Pts',(127.8,-79.5,39.1547592083257));
#23150=CARTESIAN_POINT('Ctrl Pts',(127.906598085016,-79.5,39.2650394043711));
#23151=CARTESIAN_POINT('Ctrl Pts',(128.017391828056,-79.5,39.3712639109814));
#23152=CARTESIAN_POINT('Ctrl Pts',(128.132061068702,-79.5,39.4731257714508));
#23153=CARTESIAN_POINT('Ctrl Pts',(127.8,-80.,39.8469378186781));
#23154=CARTESIAN_POINT('Ctrl Pts',(127.675853962606,-80.,39.7366576226328));
#23155=CARTESIAN_POINT('Ctrl Pts',(127.555667352303,-79.9884233304841,39.6218455594625));
#23156=CARTESIAN_POINT('Ctrl Pts',(127.441253216958,-79.9675621326039,39.5015279070509));
#23157=CARTESIAN_POINT('Ctrl Pts',(127.8,-79.5,39.1547592083257));
#23158=CARTESIAN_POINT('Ctrl Pts',(127.906598085016,-79.5,39.2650394043711));
#23159=CARTESIAN_POINT('Ctrl Pts',(128.017391828056,-79.5,39.3712639109814));
#23160=CARTESIAN_POINT('Ctrl Pts',(128.132061068702,-79.5,39.4731257714508));
#23161=CARTESIAN_POINT('Ctrl Pts',(128.54404266268,-79.9563089001744,40.4157589290663));
#23162=CARTESIAN_POINT('Ctrl Pts',(129.263478466491,-79.8576414856572,40.8800278303036));
#23163=CARTESIAN_POINT('Ctrl Pts',(130.510527749596,-79.5181474324866,41.3195198524985));
#23164=CARTESIAN_POINT('Ctrl Pts',(132.744228870775,-79.3603992958393,41.4617635687488));
#23165=CARTESIAN_POINT('Ctrl Pts',(134.073121497376,-79.6275582417068,41.2167183481929));
#23166=CARTESIAN_POINT('Ctrl Pts',(135.177351519555,-79.8589667197824,40.7531589114286));
#23167=CARTESIAN_POINT('Ctrl Pts',(135.474525863015,-79.9177118275984,40.597373300574));
#23168=CARTESIAN_POINT('Ctrl Pts',(135.75595733732,-79.9563089001744,40.4157589290663));
#23169=CARTESIAN_POINT('Ctrl Pts',(128.635473025189,-79.8042059334496,40.2771726193775));
#23170=CARTESIAN_POINT('Ctrl Pts',(129.319563648041,-79.7397843653748,40.7221495906837));
#23171=CARTESIAN_POINT('Ctrl Pts',(130.533213469025,-79.4441152647883,41.1796746951226));
#23172=CARTESIAN_POINT('Ctrl Pts',(132.736413250553,-79.3011545618022,41.3347921069928));
#23173=CARTESIAN_POINT('Ctrl Pts',(134.044121571737,-79.5424668480034,41.0686029938564));
#23174=CARTESIAN_POINT('Ctrl Pts',(135.111425223576,-79.732438948176,40.6038297677597));
#23175=CARTESIAN_POINT('Ctrl Pts',(135.396943415579,-79.778678001914,40.4513160090136));
#23176=CARTESIAN_POINT('Ctrl Pts',(135.664526974811,-79.8042059334496,40.2771726193775));
#23177=CARTESIAN_POINT('Ctrl Pts',(128.726903387699,-79.6521029667248,40.1385863096888));
#23178=CARTESIAN_POINT('Ctrl Pts',(129.376253487347,-79.6178571202824,40.5629593217589));
#23179=CARTESIAN_POINT('Ctrl Pts',(130.555816201489,-79.3692164847842,41.0391855198158));
#23180=CARTESIAN_POINT('Ctrl Pts',(132.728756439743,-79.2403531910525,41.2071722557424));
#23181=CARTESIAN_POINT('Ctrl Pts',(134.01444316861,-79.4556586603759,40.9185292434998));
#23182=CARTESIAN_POINT('Ctrl Pts',(135.045825549294,-79.6063925474043,40.4552855381036));
#23183=CARTESIAN_POINT('Ctrl Pts',(135.319060054152,-79.6390338256844,40.3045183600193));
#23184=CARTESIAN_POINT('Ctrl Pts',(135.573096612301,-79.6521029667248,40.1385863096888));
#23185=CARTESIAN_POINT('Ctrl Pts',(128.818333750208,-79.5,40.));
#23186=CARTESIAN_POINT('Ctrl Pts',(129.432338668897,-79.5,40.4050810821389));
#23187=CARTESIAN_POINT('Ctrl Pts',(130.578501920918,-79.2951843170859,40.8993403624398));
#23188=CARTESIAN_POINT('Ctrl Pts',(132.720940819521,-79.1811084570154,41.0802007939864));
#23189=CARTESIAN_POINT('Ctrl Pts',(133.985443242971,-79.3705672666724,40.7704138891633));
#23190=CARTESIAN_POINT('Ctrl Pts',(134.979899253315,-79.4798647757979,40.3059563944347));
#23191=CARTESIAN_POINT('Ctrl Pts',(135.241477606716,-79.5,40.1584610684589));
#23192=CARTESIAN_POINT('Ctrl Pts',(135.481666249792,-79.5,40.));
#23193=CARTESIAN_POINT('',(135.481666249792,-79.5,40.));
#23194=CARTESIAN_POINT('',(135.75595733732,-79.9563089001744,40.4157589290663));
#23195=CARTESIAN_POINT('',(135.481666249792,-79.5,40.));
#23196=CARTESIAN_POINT('',(128.54404266268,-79.9563089001744,40.4157589290663));
#23197=CARTESIAN_POINT('Ctrl Pts',(135.75595733732,-79.9563089001744,40.4157589290663));
#23198=CARTESIAN_POINT('Ctrl Pts',(135.474525863015,-79.9177118275984,40.597373300574));
#23199=CARTESIAN_POINT('Ctrl Pts',(135.177351519555,-79.8589667197824,40.7531589114286));
#23200=CARTESIAN_POINT('Ctrl Pts',(134.073121497376,-79.6275582417068,41.2167183481929));
#23201=CARTESIAN_POINT('Ctrl Pts',(132.744228870775,-79.3603992958393,41.4617635687488));
#23202=CARTESIAN_POINT('Ctrl Pts',(130.510527749596,-79.5181474324866,41.3195198524985));
#23203=CARTESIAN_POINT('Ctrl Pts',(129.263478466491,-79.8576414856572,40.8800278303036));
#23204=CARTESIAN_POINT('Ctrl Pts',(128.54404266268,-79.9563089001744,40.4157589290663));
#23205=CARTESIAN_POINT('',(128.818333750208,-79.5,40.));
#23206=CARTESIAN_POINT('',(128.54404266268,-79.9563089001744,40.4157589290663));
#23207=CARTESIAN_POINT('Ctrl Pts',(128.818333750208,-79.5,40.));
#23208=CARTESIAN_POINT('Ctrl Pts',(129.432338668897,-79.5,40.4050810821389));
#23209=CARTESIAN_POINT('Ctrl Pts',(130.578501920918,-79.2951843170859,40.8993403624398));
#23210=CARTESIAN_POINT('Ctrl Pts',(132.720940819521,-79.1811084570154,41.0802007939864));
#23211=CARTESIAN_POINT('Ctrl Pts',(133.985443242971,-79.3705672666724,40.7704138891633));
#23212=CARTESIAN_POINT('Ctrl Pts',(134.979899253315,-79.4798647757979,40.3059563944347));
#23213=CARTESIAN_POINT('Ctrl Pts',(135.241477606716,-79.5,40.1584610684589));
#23214=CARTESIAN_POINT('Ctrl Pts',(135.481666249792,-79.5,40.));
#23215=CARTESIAN_POINT('Ctrl Pts',(127.978669277077,-80.,40.));
#23216=CARTESIAN_POINT('Ctrl Pts',(128.159138387108,-80.,40.1490685828142));
#23217=CARTESIAN_POINT('Ctrl Pts',(128.347413162951,-79.9832757598348,40.2888692728855));
#23218=CARTESIAN_POINT('Ctrl Pts',(128.54404266268,-79.9563089001744,40.4157589290663));
#23219=CARTESIAN_POINT('Ctrl Pts',(128.08481000794,-79.8333333333333,39.8715012722646));
#23220=CARTESIAN_POINT('Ctrl Pts',(128.260687028658,-79.8333333333333,40.0167767613686));
#23221=CARTESIAN_POINT('Ctrl Pts',(128.444230322027,-79.8221838398899,40.152892198886));
#23222=CARTESIAN_POINT('Ctrl Pts',(128.635473025189,-79.8042059334496,40.2771726193776));
#23223=CARTESIAN_POINT('Ctrl Pts',(128.190950738804,-79.6666666666667,39.7430025445293));
#23224=CARTESIAN_POINT('Ctrl Pts',(128.362235670207,-79.6666666666667,39.8844849399229));
#23225=CARTESIAN_POINT('Ctrl Pts',(128.541047481102,-79.6610919199449,40.0169151248865));
#23226=CARTESIAN_POINT('Ctrl Pts',(128.726903387699,-79.6521029667248,40.1385863096888));
#23227=CARTESIAN_POINT('Ctrl Pts',(128.297091469667,-79.5,39.6145038167939));
#23228=CARTESIAN_POINT('Ctrl Pts',(128.463784311757,-79.5,39.7521931184773));
#23229=CARTESIAN_POINT('Ctrl Pts',(128.637864640177,-79.5,39.8809380508869));
#23230=CARTESIAN_POINT('Ctrl Pts',(128.818333750208,-79.5,40.));
#23231=CARTESIAN_POINT('Ctrl Pts',(128.54404266268,-79.9563089001744,40.4157589290663));
#23232=CARTESIAN_POINT('Ctrl Pts',(128.347413162951,-79.9832757598348,40.2888692728855));
#23233=CARTESIAN_POINT('Ctrl Pts',(128.159138387108,-80.,40.1490685828142));
#23234=CARTESIAN_POINT('Ctrl Pts',(127.978669277077,-80.,40.));
#23235=CARTESIAN_POINT('Ctrl Pts',(128.297091469667,-79.5,39.6145038167939));
#23236=CARTESIAN_POINT('Ctrl Pts',(128.463784311757,-79.5,39.7521931184773));
#23237=CARTESIAN_POINT('Ctrl Pts',(128.637864640177,-79.5,39.8809380508869));
#23238=CARTESIAN_POINT('Ctrl Pts',(128.818333750208,-79.5,40.));
#23239=CARTESIAN_POINT('Ctrl Pts',(135.75595733732,-79.9563089001744,40.4157589290663));
#23240=CARTESIAN_POINT('Ctrl Pts',(135.952586837049,-79.9832757598348,40.2888692728855));
#23241=CARTESIAN_POINT('Ctrl Pts',(136.140861612892,-80.,40.1490685828142));
#23242=CARTESIAN_POINT('Ctrl Pts',(136.321330722923,-80.,40.));
#23243=CARTESIAN_POINT('Ctrl Pts',(135.664526974811,-79.8042059334496,40.2771726193776));
#23244=CARTESIAN_POINT('Ctrl Pts',(135.855769677973,-79.8221838398899,40.152892198886));
#23245=CARTESIAN_POINT('Ctrl Pts',(136.039312971342,-79.8333333333333,40.0167767613686));
#23246=CARTESIAN_POINT('Ctrl Pts',(136.21518999206,-79.8333333333333,39.8715012722646));
#23247=CARTESIAN_POINT('Ctrl Pts',(135.573096612301,-79.6521029667248,40.1385863096888));
#23248=CARTESIAN_POINT('Ctrl Pts',(135.758952518898,-79.6610919199449,40.0169151248865));
#23249=CARTESIAN_POINT('Ctrl Pts',(135.937764329793,-79.6666666666667,39.8844849399229));
#23250=CARTESIAN_POINT('Ctrl Pts',(136.109049261197,-79.6666666666667,39.7430025445293));
#23251=CARTESIAN_POINT('Ctrl Pts',(135.481666249792,-79.5,40.));
#23252=CARTESIAN_POINT('Ctrl Pts',(135.662135359823,-79.5,39.8809380508869));
#23253=CARTESIAN_POINT('Ctrl Pts',(135.836215688243,-79.5,39.7521931184773));
#23254=CARTESIAN_POINT('Ctrl Pts',(136.002908530333,-79.5,39.6145038167939));
#23255=CARTESIAN_POINT('Ctrl Pts',(136.321330722923,-80.,40.));
#23256=CARTESIAN_POINT('Ctrl Pts',(136.140861612892,-80.,40.1490685828142));
#23257=CARTESIAN_POINT('Ctrl Pts',(135.952586837049,-79.9832757598348,40.2888692728855));
#23258=CARTESIAN_POINT('Ctrl Pts',(135.75595733732,-79.9563089001744,40.4157589290663));
#23259=CARTESIAN_POINT('Ctrl Pts',(135.481666249792,-79.5,40.));
#23260=CARTESIAN_POINT('Ctrl Pts',(135.662135359823,-79.5,39.8809380508869));
#23261=CARTESIAN_POINT('Ctrl Pts',(135.836215688243,-79.5,39.7521931184773));
#23262=CARTESIAN_POINT('Ctrl Pts',(136.002908530333,-79.5,39.6145038167939));
#23263=CARTESIAN_POINT('Origin',(125.8,-80.,-42.));
#23264=CARTESIAN_POINT('',(127.8,-80.,40.));
#23265=CARTESIAN_POINT('',(138.1,-80.,40.));
#23266=CARTESIAN_POINT('',(127.8,-80.,-21.));
#23267=CARTESIAN_POINT('Origin',(138.1,-78.,40.));
#23268=CARTESIAN_POINT('',(173.,-78.,42.));
#23269=CARTESIAN_POINT('Origin',(173.,-78.,40.));
#23270=CARTESIAN_POINT('',(127.8,-78.,42.));
#23271=CARTESIAN_POINT('',(138.1,-78.,42.));
#23272=CARTESIAN_POINT('Origin',(127.8,-78.,40.));
#23273=CARTESIAN_POINT('Origin',(132.15,-80.,34.95));
#23274=CARTESIAN_POINT('',(126.1,-62.,34.95));
#23275=CARTESIAN_POINT('',(126.1,-80.,34.95));
#23276=CARTESIAN_POINT('Origin',(132.15,-62.,34.95));
#23277=CARTESIAN_POINT('Origin',(167.85,-79.75,-34.95));
#23278=CARTESIAN_POINT('',(172.606870229008,-79.5,-38.6882730804986));
#23279=CARTESIAN_POINT('',(173.,-80.,-38.9972212689696));
#23280=CARTESIAN_POINT('',(171.702908530333,-79.5,-39.6145038167939));
#23281=CARTESIAN_POINT('Origin',(167.85,-79.5,-34.95));
#23282=CARTESIAN_POINT('',(172.021330722923,-80.,-40.));
#23283=CARTESIAN_POINT('',(171.702908530333,-79.5,-39.6145038167939));
#23284=CARTESIAN_POINT('Origin',(167.85,-80.,-34.95));
#23285=CARTESIAN_POINT('Ctrl Pts',(171.45595733732,-79.9563089001744,-40.4157589290663));
#23286=CARTESIAN_POINT('Ctrl Pts',(171.174525863015,-79.9177118275984,-40.5973733005741));
#23287=CARTESIAN_POINT('Ctrl Pts',(170.877133620805,-79.8584176853714,-40.7532400506391));
#23288=CARTESIAN_POINT('Ctrl Pts',(170.169540370025,-79.7125526259848,-41.0499532608049));
#23289=CARTESIAN_POINT('Ctrl Pts',(169.328708923034,-79.5317501944907,-41.2992260645674));
#23290=CARTESIAN_POINT('Ctrl Pts',(167.994480347266,-79.3928715097831,-41.4336284766179));
#23291=CARTESIAN_POINT('Ctrl Pts',(166.882801505965,-79.4695633321676,-41.3620613931844));
#23292=CARTESIAN_POINT('Ctrl Pts',(165.580759305438,-79.685637902348,-41.1009423825717));
#23293=CARTESIAN_POINT('Ctrl Pts',(164.783619515538,-79.8823083392865,-40.7639606049943));
#23294=CARTESIAN_POINT('Ctrl Pts',(164.24404266268,-79.9563089001744,-40.4157589290663));
#23295=CARTESIAN_POINT('Ctrl Pts',(171.364526974811,-79.8042059334496,-40.2771726193776));
#23296=CARTESIAN_POINT('Ctrl Pts',(171.096840486452,-79.7785219817075,-40.4510535247975));
#23297=CARTESIAN_POINT('Ctrl Pts',(170.811354113016,-79.7321092034511,-40.6042844297561));
#23298=CARTESIAN_POINT('Ctrl Pts',(170.127025529992,-79.6122205931232,-40.9007863045982));
#23299=CARTESIAN_POINT('Ctrl Pts',(169.306987876026,-79.4555015304909,-41.1586880147503));
#23300=CARTESIAN_POINT('Ctrl Pts',(167.992632142232,-79.3306382944245,-41.3037702678481));
#23301=CARTESIAN_POINT('Ctrl Pts',(166.896385122953,-79.3998081962153,-41.2261517187221));
#23302=CARTESIAN_POINT('Ctrl Pts',(165.620142363097,-79.5900140227366,-40.9520929972732));
#23303=CARTESIAN_POINT('Ctrl Pts',(164.848437702289,-79.7556443218945,-40.6109203734391));
#23304=CARTESIAN_POINT('Ctrl Pts',(164.335473025189,-79.8042059334496,-40.2771726193775));
#23305=CARTESIAN_POINT('Ctrl Pts',(171.273096612301,-79.6521029667248,-40.1385863096888));
#23306=CARTESIAN_POINT('Ctrl Pts',(171.019162983279,-79.6391898458909,-40.3047808442354));
#23307=CARTESIAN_POINT('Ctrl Pts',(170.745556079207,-79.6057940059781,-40.4552285335035));
#23308=CARTESIAN_POINT('Ctrl Pts',(170.084629406995,-79.5115784193021,-40.7517034972954));
#23309=CARTESIAN_POINT('Ctrl Pts',(169.28540248269,-79.3786758644581,-41.0179405613137));
#23310=CARTESIAN_POINT('Ctrl Pts',(167.990907646826,-79.2678110265308,-41.1737902675345));
#23311=CARTESIAN_POINT('Ctrl Pts',(166.910151354644,-79.3291259492015,-41.0899409156025));
#23312=CARTESIAN_POINT('Ctrl Pts',(165.659561421505,-79.4936989232242,-40.8031820113288));
#23313=CARTESIAN_POINT('Ctrl Pts',(164.914019252474,-79.626664017392,-40.4568510431595));
#23314=CARTESIAN_POINT('Ctrl Pts',(164.426903387699,-79.6521029667248,-40.1385863096888));
#23315=CARTESIAN_POINT('Ctrl Pts',(171.181666249792,-79.5,-40.));
#23316=CARTESIAN_POINT('Ctrl Pts',(170.941477606716,-79.5,-40.1584610684588));
#23317=CARTESIAN_POINT('Ctrl Pts',(170.679776571418,-79.4794855240578,-40.3062729126205));
#23318=CARTESIAN_POINT('Ctrl Pts',(170.042114566962,-79.4112463864405,-40.6025365410887));
#23319=CARTESIAN_POINT('Ctrl Pts',(169.263681435681,-79.3024272004583,-40.8774025114966));
#23320=CARTESIAN_POINT('Ctrl Pts',(167.989059441792,-79.2055778111722,-41.0439320587647));
#23321=CARTESIAN_POINT('Ctrl Pts',(166.923734971632,-79.2593708132491,-40.9540312411402));
#23322=CARTESIAN_POINT('Ctrl Pts',(165.698944479165,-79.3980750436128,-40.6543326260304));
#23323=CARTESIAN_POINT('Ctrl Pts',(164.978837439225,-79.5,-40.3038108116042));
#23324=CARTESIAN_POINT('Ctrl Pts',(164.518333750208,-79.5,-40.));
#23325=CARTESIAN_POINT('',(164.518333750209,-79.5,-40.));
#23326=CARTESIAN_POINT('',(164.24404266268,-79.9563089001744,-40.4157589290664));
#23327=CARTESIAN_POINT('',(164.518333750209,-79.5,-40.));
#23328=CARTESIAN_POINT('',(171.45595733732,-79.9563089001744,-40.4157589290663));
#23329=CARTESIAN_POINT('Ctrl Pts',(164.24404266268,-79.9563089001744,-40.4157589290663));
#23330=CARTESIAN_POINT('Ctrl Pts',(164.783619515538,-79.8823083392865,-40.7639606049943));
#23331=CARTESIAN_POINT('Ctrl Pts',(165.580759305438,-79.685637902348,-41.1009423825717));
#23332=CARTESIAN_POINT('Ctrl Pts',(166.882801505965,-79.4695633321676,-41.3620613931844));
#23333=CARTESIAN_POINT('Ctrl Pts',(167.994480347266,-79.3928715097831,-41.4336284766179));
#23334=CARTESIAN_POINT('Ctrl Pts',(169.328708923034,-79.5317501944907,-41.2992260645674));
#23335=CARTESIAN_POINT('Ctrl Pts',(170.169540370025,-79.7125526259848,-41.0499532608049));
#23336=CARTESIAN_POINT('Ctrl Pts',(170.877133620805,-79.8584176853714,-40.7532400506391));
#23337=CARTESIAN_POINT('Ctrl Pts',(171.174525863015,-79.9177118275984,-40.5973733005741));
#23338=CARTESIAN_POINT('Ctrl Pts',(171.45595733732,-79.9563089001744,-40.4157589290663));
#23339=CARTESIAN_POINT('',(171.181666249792,-79.5,-40.));
#23340=CARTESIAN_POINT('',(171.45595733732,-79.9563089001744,-40.4157589290663));
#23341=CARTESIAN_POINT('Ctrl Pts',(171.181666249792,-79.5,-40.));
#23342=CARTESIAN_POINT('Ctrl Pts',(170.941477606716,-79.5,-40.1584610684588));
#23343=CARTESIAN_POINT('Ctrl Pts',(170.679776571418,-79.4794855240578,-40.3062729126205));
#23344=CARTESIAN_POINT('Ctrl Pts',(170.042114566962,-79.4112463864405,-40.6025365410887));
#23345=CARTESIAN_POINT('Ctrl Pts',(169.263681435681,-79.3024272004583,-40.8774025114966));
#23346=CARTESIAN_POINT('Ctrl Pts',(167.989059441792,-79.2055778111722,-41.0439320587647));
#23347=CARTESIAN_POINT('Ctrl Pts',(166.923734971632,-79.2593708132491,-40.9540312411402));
#23348=CARTESIAN_POINT('Ctrl Pts',(165.698944479165,-79.3980750436128,-40.6543326260304));
#23349=CARTESIAN_POINT('Ctrl Pts',(164.978837439225,-79.5,-40.3038108116042));
#23350=CARTESIAN_POINT('Ctrl Pts',(164.518333750208,-79.5,-40.));
#23351=CARTESIAN_POINT('Ctrl Pts',(172.021330722923,-80.,-40.));
#23352=CARTESIAN_POINT('Ctrl Pts',(171.840861612892,-80.,-40.1490685828142));
#23353=CARTESIAN_POINT('Ctrl Pts',(171.652586837049,-79.9832757598348,-40.2888692728855));
#23354=CARTESIAN_POINT('Ctrl Pts',(171.45595733732,-79.9563089001744,-40.4157589290663));
#23355=CARTESIAN_POINT('Ctrl Pts',(171.91518999206,-79.8333333333333,-39.8715012722646));
#23356=CARTESIAN_POINT('Ctrl Pts',(171.739312971342,-79.8333333333333,-40.0167767613686));
#23357=CARTESIAN_POINT('Ctrl Pts',(171.555769677973,-79.8221838398899,-40.152892198886));
#23358=CARTESIAN_POINT('Ctrl Pts',(171.364526974811,-79.8042059334496,-40.2771726193776));
#23359=CARTESIAN_POINT('Ctrl Pts',(171.809049261197,-79.6666666666667,-39.7430025445293));
#23360=CARTESIAN_POINT('Ctrl Pts',(171.637764329793,-79.6666666666667,-39.8844849399229));
#23361=CARTESIAN_POINT('Ctrl Pts',(171.458952518898,-79.6610919199449,-40.0169151248865));
#23362=CARTESIAN_POINT('Ctrl Pts',(171.273096612301,-79.6521029667248,-40.1385863096888));
#23363=CARTESIAN_POINT('Ctrl Pts',(171.702908530333,-79.5,-39.6145038167939));
#23364=CARTESIAN_POINT('Ctrl Pts',(171.536215688243,-79.5,-39.7521931184773));
#23365=CARTESIAN_POINT('Ctrl Pts',(171.362135359823,-79.5,-39.8809380508869));
#23366=CARTESIAN_POINT('Ctrl Pts',(171.181666249792,-79.5,-40.));
#23367=CARTESIAN_POINT('Ctrl Pts',(171.45595733732,-79.9563089001744,-40.4157589290663));
#23368=CARTESIAN_POINT('Ctrl Pts',(171.652586837049,-79.9832757598348,-40.2888692728855));
#23369=CARTESIAN_POINT('Ctrl Pts',(171.840861612892,-80.,-40.1490685828142));
#23370=CARTESIAN_POINT('Ctrl Pts',(172.021330722923,-80.,-40.));
#23371=CARTESIAN_POINT('Ctrl Pts',(171.702908530333,-79.5,-39.6145038167939));
#23372=CARTESIAN_POINT('Ctrl Pts',(171.536215688243,-79.5,-39.7521931184773));
#23373=CARTESIAN_POINT('Ctrl Pts',(171.362135359823,-79.5,-39.8809380508869));
#23374=CARTESIAN_POINT('Ctrl Pts',(171.181666249792,-79.5,-40.));
#23375=CARTESIAN_POINT('Origin',(167.85,-79.75,-34.95));
#23376=CARTESIAN_POINT('',(163.997091469667,-79.5,-39.6145038167939));
#23377=CARTESIAN_POINT('',(163.678669277077,-80.,-40.));
#23378=CARTESIAN_POINT('',(161.8,-79.5,-34.95));
#23379=CARTESIAN_POINT('Origin',(167.85,-79.5,-34.95));
#23380=CARTESIAN_POINT('',(172.606870229008,-79.5,-31.2117269195014));
#23381=CARTESIAN_POINT('Origin',(167.85,-79.5,-34.95));
#23382=CARTESIAN_POINT('',(172.606870229008,-79.5,-31.2117269195014));
#23383=CARTESIAN_POINT('Ctrl Pts',(164.24404266268,-79.9563089001744,-40.4157589290664));
#23384=CARTESIAN_POINT('Ctrl Pts',(164.047413162951,-79.9832757598348,-40.2888692728855));
#23385=CARTESIAN_POINT('Ctrl Pts',(163.859138387108,-80.,-40.1490685828142));
#23386=CARTESIAN_POINT('Ctrl Pts',(163.678669277077,-80.,-40.));
#23387=CARTESIAN_POINT('Ctrl Pts',(164.335473025189,-79.8042059334496,-40.2771726193776));
#23388=CARTESIAN_POINT('Ctrl Pts',(164.144230322027,-79.8221838398899,-40.152892198886));
#23389=CARTESIAN_POINT('Ctrl Pts',(163.960687028658,-79.8333333333333,-40.0167767613686));
#23390=CARTESIAN_POINT('Ctrl Pts',(163.78481000794,-79.8333333333333,-39.8715012722646));
#23391=CARTESIAN_POINT('Ctrl Pts',(164.426903387699,-79.6521029667248,-40.1385863096888));
#23392=CARTESIAN_POINT('Ctrl Pts',(164.241047481102,-79.6610919199449,-40.0169151248865));
#23393=CARTESIAN_POINT('Ctrl Pts',(164.062235670207,-79.6666666666667,-39.8844849399229));
#23394=CARTESIAN_POINT('Ctrl Pts',(163.890950738804,-79.6666666666667,-39.7430025445293));
#23395=CARTESIAN_POINT('Ctrl Pts',(164.518333750209,-79.5,-40.));
#23396=CARTESIAN_POINT('Ctrl Pts',(164.337864640177,-79.5,-39.880938050887));
#23397=CARTESIAN_POINT('Ctrl Pts',(164.163784311757,-79.5,-39.7521931184773));
#23398=CARTESIAN_POINT('Ctrl Pts',(163.997091469667,-79.5,-39.6145038167939));
#23399=CARTESIAN_POINT('Ctrl Pts',(163.678669277077,-80.,-40.));
#23400=CARTESIAN_POINT('Ctrl Pts',(163.859138387108,-80.,-40.1490685828142));
#23401=CARTESIAN_POINT('Ctrl Pts',(164.047413162951,-79.9832757598348,-40.2888692728855));
#23402=CARTESIAN_POINT('Ctrl Pts',(164.24404266268,-79.9563089001744,-40.4157589290664));
#23403=CARTESIAN_POINT('Ctrl Pts',(164.518333750209,-79.5,-40.));
#23404=CARTESIAN_POINT('Ctrl Pts',(164.337864640177,-79.5,-39.880938050887));
#23405=CARTESIAN_POINT('Ctrl Pts',(164.163784311757,-79.5,-39.7521931184773));
#23406=CARTESIAN_POINT('Ctrl Pts',(163.997091469667,-79.5,-39.6145038167939));
#23407=CARTESIAN_POINT('Ctrl Pts',(173.423859320912,-79.9545698442563,-31.5137951986038));
#23408=CARTESIAN_POINT('Ctrl Pts',(173.770549629633,-79.8793881262671,-32.089231778783));
#23409=CARTESIAN_POINT('Ctrl Pts',(174.252601993115,-79.5822812285807,-33.3779001916364));
#23410=CARTESIAN_POINT('Ctrl Pts',(174.412080939248,-79.4069780593559,-35.8280882420133));
#23411=CARTESIAN_POINT('Ctrl Pts',(173.943894783993,-79.8417972672725,-37.5230499311273));
#23412=CARTESIAN_POINT('Ctrl Pts',(173.423859320912,-79.9545698442563,-38.3862048013962));
#23413=CARTESIAN_POINT('Ctrl Pts',(173.282572880608,-79.8030465628375,-31.6008962746434));
#23414=CARTESIAN_POINT('Ctrl Pts',(173.615386259174,-79.7529254175114,-32.1494660917847));
#23415=CARTESIAN_POINT('Ctrl Pts',(174.107434573101,-79.5010021055637,-33.3992547618186));
#23416=CARTESIAN_POINT('Ctrl Pts',(174.281848391946,-79.3436199687264,-35.8173556194049));
#23417=CARTESIAN_POINT('Ctrl Pts',(173.781792948457,-79.7278648448483,-37.4762489996446));
#23418=CARTESIAN_POINT('Ctrl Pts',(173.282572880608,-79.8030465628376,-38.2991037253567));
#23419=CARTESIAN_POINT('Ctrl Pts',(173.141286440304,-79.6515232814188,-31.6879973506829));
#23420=CARTESIAN_POINT('Ctrl Pts',(173.460222888715,-79.6264627087557,-32.2097004047863));
#23421=CARTESIAN_POINT('Ctrl Pts',(173.962267153088,-79.4197229825467,-33.4206093320008));
#23422=CARTESIAN_POINT('Ctrl Pts',(174.151615844645,-79.2802618780969,-35.8066229967965));
#23423=CARTESIAN_POINT('Ctrl Pts',(173.61969111292,-79.6139324224242,-37.4294480681618));
#23424=CARTESIAN_POINT('Ctrl Pts',(173.141286440304,-79.6515232814188,-38.2120026493171));
#23425=CARTESIAN_POINT('Ctrl Pts',(173.,-79.5,-31.7750984267225));
#23426=CARTESIAN_POINT('Ctrl Pts',(173.305059518256,-79.5,-32.2699347177879));
#23427=CARTESIAN_POINT('Ctrl Pts',(173.817099733074,-79.3384438595296,-33.4419639021829));
#23428=CARTESIAN_POINT('Ctrl Pts',(174.021383297343,-79.2169037874674,-35.795890374188));
#23429=CARTESIAN_POINT('Ctrl Pts',(173.457589277384,-79.5,-37.382647136679));
#23430=CARTESIAN_POINT('Ctrl Pts',(173.,-79.5,-38.1249015732775));
#23431=CARTESIAN_POINT('',(173.,-79.5,-38.1249015732775));
#23432=CARTESIAN_POINT('',(173.,-79.5,-38.1249015732775));
#23433=CARTESIAN_POINT('',(173.,-79.5,-31.7750984267225));
#23434=CARTESIAN_POINT('',(173.423859320912,-79.9545698442563,-31.5137951986038));
#23435=CARTESIAN_POINT('Ctrl Pts',(173.,-79.5,-31.7750984267225));
#23436=CARTESIAN_POINT('Ctrl Pts',(173.305059518256,-79.5,-32.2699347177879));
#23437=CARTESIAN_POINT('Ctrl Pts',(173.817099733074,-79.3384438595296,-33.4419639021829));
#23438=CARTESIAN_POINT('Ctrl Pts',(174.021383297343,-79.2169037874674,-35.795890374188));
#23439=CARTESIAN_POINT('Ctrl Pts',(173.457589277384,-79.5,-37.382647136679));
#23440=CARTESIAN_POINT('Ctrl Pts',(173.,-79.5,-38.1249015732775));
#23441=CARTESIAN_POINT('Ctrl Pts',(173.,-80.,-30.9027787310304));
#23442=CARTESIAN_POINT('Ctrl Pts',(173.153269804814,-80.,-31.0978111847398));
#23443=CARTESIAN_POINT('Ctrl Pts',(173.295884311895,-79.9823219353749,-31.3013822765102));
#23444=CARTESIAN_POINT('Ctrl Pts',(173.423859320912,-79.9545698442563,-31.5137951986038));
#23445=CARTESIAN_POINT('Ctrl Pts',(172.868956743003,-79.8333333333333,-31.0057614605207));
#23446=CARTESIAN_POINT('Ctrl Pts',(173.018326552783,-79.8333333333333,-31.1958312563749));
#23447=CARTESIAN_POINT('Ctrl Pts',(173.157177965592,-79.8215479569166,-31.3942768420112));
#23448=CARTESIAN_POINT('Ctrl Pts',(173.282572880608,-79.8030465628376,-31.6008962746434));
#23449=CARTESIAN_POINT('Ctrl Pts',(172.737913486005,-79.6666666666667,-31.108744190011));
#23450=CARTESIAN_POINT('Ctrl Pts',(172.883383300752,-79.6666666666667,-31.2938513280101));
#23451=CARTESIAN_POINT('Ctrl Pts',(173.018471619289,-79.6607739784583,-31.4871714075121));
#23452=CARTESIAN_POINT('Ctrl Pts',(173.141286440304,-79.6515232814188,-31.6879973506829));
#23453=CARTESIAN_POINT('Ctrl Pts',(172.606870229008,-79.5,-31.2117269195014));
#23454=CARTESIAN_POINT('Ctrl Pts',(172.748440048721,-79.5,-31.3918713996452));
#23455=CARTESIAN_POINT('Ctrl Pts',(172.879765272986,-79.5,-31.5800659730131));
#23456=CARTESIAN_POINT('Ctrl Pts',(173.,-79.5,-31.7750984267225));
#23457=CARTESIAN_POINT('Ctrl Pts',(172.606870229008,-79.5,-31.2117269195014));
#23458=CARTESIAN_POINT('Ctrl Pts',(172.748440048721,-79.5,-31.3918713996452));
#23459=CARTESIAN_POINT('Ctrl Pts',(172.879765272986,-79.5,-31.5800659730131));
#23460=CARTESIAN_POINT('Ctrl Pts',(173.,-79.5,-31.7750984267225));
#23461=CARTESIAN_POINT('Ctrl Pts',(173.423859320912,-79.9545698442563,-38.3862048013962));
#23462=CARTESIAN_POINT('Ctrl Pts',(173.295884311895,-79.9823219353749,-38.5986177234898));
#23463=CARTESIAN_POINT('Ctrl Pts',(173.153269804814,-80.,-38.8021888152602));
#23464=CARTESIAN_POINT('Ctrl Pts',(173.,-80.,-38.9972212689696));
#23465=CARTESIAN_POINT('Ctrl Pts',(173.282572880608,-79.8030465628376,-38.2991037253567));
#23466=CARTESIAN_POINT('Ctrl Pts',(173.157177965592,-79.8215479569166,-38.5057231579888));
#23467=CARTESIAN_POINT('Ctrl Pts',(173.018326552783,-79.8333333333333,-38.7041687436251));
#23468=CARTESIAN_POINT('Ctrl Pts',(172.868956743003,-79.8333333333333,-38.8942385394793));
#23469=CARTESIAN_POINT('Ctrl Pts',(173.141286440304,-79.6515232814188,-38.2120026493171));
#23470=CARTESIAN_POINT('Ctrl Pts',(173.018471619289,-79.6607739784583,-38.4128285924879));
#23471=CARTESIAN_POINT('Ctrl Pts',(172.883383300752,-79.6666666666667,-38.6061486719899));
#23472=CARTESIAN_POINT('Ctrl Pts',(172.737913486005,-79.6666666666667,-38.791255809989));
#23473=CARTESIAN_POINT('Ctrl Pts',(173.,-79.5,-38.1249015732775));
#23474=CARTESIAN_POINT('Ctrl Pts',(172.879765272986,-79.5,-38.3199340269869));
#23475=CARTESIAN_POINT('Ctrl Pts',(172.748440048721,-79.5,-38.5081286003548));
#23476=CARTESIAN_POINT('Ctrl Pts',(172.606870229008,-79.5,-38.6882730804986));
#23477=CARTESIAN_POINT('Ctrl Pts',(173.,-79.5,-38.1249015732775));
#23478=CARTESIAN_POINT('Ctrl Pts',(172.879765272986,-79.5,-38.3199340269869));
#23479=CARTESIAN_POINT('Ctrl Pts',(172.748440048721,-79.5,-38.5081286003548));
#23480=CARTESIAN_POINT('Ctrl Pts',(172.606870229008,-79.5,-38.6882730804986));
#23481=CARTESIAN_POINT('Origin',(167.85,-80.,-34.95));
#23482=CARTESIAN_POINT('',(161.8,-62.,-34.95));
#23483=CARTESIAN_POINT('',(161.8,-80.,-34.95));
#23484=CARTESIAN_POINT('Origin',(167.85,-62.,-34.95));
#23485=CARTESIAN_POINT('Origin',(132.15,-79.75,-34.95));
#23486=CARTESIAN_POINT('',(128.132061068702,-79.5,-30.4268742285492));
#23487=CARTESIAN_POINT('',(127.8,-80.,-30.0530621813219));
#23488=CARTESIAN_POINT('',(136.002908530333,-79.5,-39.6145038167939));
#23489=CARTESIAN_POINT('Origin',(132.15,-79.5,-34.95));
#23490=CARTESIAN_POINT('',(136.002908530333,-79.5,-39.6145038167939));
#23491=CARTESIAN_POINT('Ctrl Pts',(135.75595733732,-79.9563089001744,-40.4157589290663));
#23492=CARTESIAN_POINT('Ctrl Pts',(134.86451977282,-79.8340522106591,-40.9910246253239));
#23493=CARTESIAN_POINT('Ctrl Pts',(133.087218623523,-79.3066015901477,-41.5050220648132));
#23494=CARTESIAN_POINT('Ctrl Pts',(130.476050150785,-79.522629291586,-41.3301097614915));
#23495=CARTESIAN_POINT('Ctrl Pts',(129.138334372346,-79.8748044404976,-40.7992693932379));
#23496=CARTESIAN_POINT('Ctrl Pts',(128.54404266268,-79.9563089001744,-40.4157589290663));
#23497=CARTESIAN_POINT('Ctrl Pts',(135.664526974811,-79.8042059334496,-40.2771726193776));
#23498=CARTESIAN_POINT('Ctrl Pts',(134.816635130887,-79.7227014737727,-40.827992194093));
#23499=CARTESIAN_POINT('Ctrl Pts',(133.07704459393,-79.2522044265217,-41.3826863416403));
#23500=CARTESIAN_POINT('Ctrl Pts',(130.49676626701,-79.4479951419512,-41.1885457912196));
#23501=CARTESIAN_POINT('Ctrl Pts',(129.200734254472,-79.7498696269984,-40.6443856691878));
#23502=CARTESIAN_POINT('Ctrl Pts',(128.635473025189,-79.8042059334496,-40.2771726193776));
#23503=CARTESIAN_POINT('Ctrl Pts',(135.573096612301,-79.6521029667248,-40.1385863096888));
#23504=CARTESIAN_POINT('Ctrl Pts',(134.768750488954,-79.6113507368864,-40.6649597628621));
#23505=CARTESIAN_POINT('Ctrl Pts',(133.066870564337,-79.1978072628957,-41.2603506184674));
#23506=CARTESIAN_POINT('Ctrl Pts',(130.517482383235,-79.3733609923163,-41.0469818209476));
#23507=CARTESIAN_POINT('Ctrl Pts',(129.263134136597,-79.6249348134992,-40.4895019451377));
#23508=CARTESIAN_POINT('Ctrl Pts',(128.726903387699,-79.6521029667248,-40.1385863096888));
#23509=CARTESIAN_POINT('Ctrl Pts',(135.481666249792,-79.5,-40.));
#23510=CARTESIAN_POINT('Ctrl Pts',(134.720865847021,-79.5,-40.5019273316312));
#23511=CARTESIAN_POINT('Ctrl Pts',(133.056696534744,-79.1434100992696,-41.1380148952945));
#23512=CARTESIAN_POINT('Ctrl Pts',(130.53819849946,-79.2987268426815,-40.9054178506757));
#23513=CARTESIAN_POINT('Ctrl Pts',(129.325534018722,-79.5,-40.3346182210876));
#23514=CARTESIAN_POINT('Ctrl Pts',(128.818333750208,-79.5,-40.));
#23515=CARTESIAN_POINT('',(128.818333750208,-79.5,-40.));
#23516=CARTESIAN_POINT('',(128.54404266268,-79.9563089001744,-40.4157589290663));
#23517=CARTESIAN_POINT('',(128.818333750208,-79.5,-40.));
#23518=CARTESIAN_POINT('',(135.75595733732,-79.9563089001744,-40.4157589290663));
#23519=CARTESIAN_POINT('Ctrl Pts',(128.54404266268,-79.9563089001744,-40.4157589290663));
#23520=CARTESIAN_POINT('Ctrl Pts',(129.138334372346,-79.8748044404976,-40.7992693932379));
#23521=CARTESIAN_POINT('Ctrl Pts',(130.476050150785,-79.522629291586,-41.3301097614915));
#23522=CARTESIAN_POINT('Ctrl Pts',(133.087218623523,-79.3066015901477,-41.5050220648132));
#23523=CARTESIAN_POINT('Ctrl Pts',(134.86451977282,-79.8340522106591,-40.9910246253239));
#23524=CARTESIAN_POINT('Ctrl Pts',(135.75595733732,-79.9563089001744,-40.4157589290663));
#23525=CARTESIAN_POINT('',(135.481666249792,-79.5,-40.));
#23526=CARTESIAN_POINT('',(135.75595733732,-79.9563089001744,-40.4157589290663));
#23527=CARTESIAN_POINT('Ctrl Pts',(135.481666249792,-79.5,-40.));
#23528=CARTESIAN_POINT('Ctrl Pts',(134.720865847021,-79.5,-40.5019273316312));
#23529=CARTESIAN_POINT('Ctrl Pts',(133.056696534744,-79.1434100992696,-41.1380148952945));
#23530=CARTESIAN_POINT('Ctrl Pts',(130.53819849946,-79.2987268426815,-40.9054178506757));
#23531=CARTESIAN_POINT('Ctrl Pts',(129.325534018722,-79.5,-40.3346182210876));
#23532=CARTESIAN_POINT('Ctrl Pts',(128.818333750208,-79.5,-40.));
#23533=CARTESIAN_POINT('Ctrl Pts',(136.321330722923,-80.,-40.));
#23534=CARTESIAN_POINT('Ctrl Pts',(136.140861612892,-80.,-40.1490685828142));
#23535=CARTESIAN_POINT('Ctrl Pts',(135.952586837049,-79.9832757598348,-40.2888692728855));
#23536=CARTESIAN_POINT('Ctrl Pts',(135.75595733732,-79.9563089001744,-40.4157589290663));
#23537=CARTESIAN_POINT('Ctrl Pts',(136.21518999206,-79.8333333333333,-39.8715012722646));
#23538=CARTESIAN_POINT('Ctrl Pts',(136.039312971342,-79.8333333333333,-40.0167767613686));
#23539=CARTESIAN_POINT('Ctrl Pts',(135.855769677973,-79.8221838398898,-40.152892198886));
#23540=CARTESIAN_POINT('Ctrl Pts',(135.664526974811,-79.8042059334496,-40.2771726193775));
#23541=CARTESIAN_POINT('Ctrl Pts',(136.109049261196,-79.6666666666667,-39.7430025445293));
#23542=CARTESIAN_POINT('Ctrl Pts',(135.937764329793,-79.6666666666667,-39.8844849399229));
#23543=CARTESIAN_POINT('Ctrl Pts',(135.758952518898,-79.6610919199449,-40.0169151248865));
#23544=CARTESIAN_POINT('Ctrl Pts',(135.573096612301,-79.6521029667248,-40.1385863096888));
#23545=CARTESIAN_POINT('Ctrl Pts',(136.002908530333,-79.5,-39.6145038167939));
#23546=CARTESIAN_POINT('Ctrl Pts',(135.836215688243,-79.5,-39.7521931184773));
#23547=CARTESIAN_POINT('Ctrl Pts',(135.662135359823,-79.5,-39.8809380508869));
#23548=CARTESIAN_POINT('Ctrl Pts',(135.481666249792,-79.5,-40.));
#23549=CARTESIAN_POINT('Ctrl Pts',(135.75595733732,-79.9563089001744,-40.4157589290663));
#23550=CARTESIAN_POINT('Ctrl Pts',(135.952586837049,-79.9832757598348,-40.2888692728855));
#23551=CARTESIAN_POINT('Ctrl Pts',(136.140861612892,-80.,-40.1490685828142));
#23552=CARTESIAN_POINT('Ctrl Pts',(136.321330722923,-80.,-40.));
#23553=CARTESIAN_POINT('Ctrl Pts',(136.002908530333,-79.5,-39.6145038167939));
#23554=CARTESIAN_POINT('Ctrl Pts',(135.836215688243,-79.5,-39.7521931184773));
#23555=CARTESIAN_POINT('Ctrl Pts',(135.662135359823,-79.5,-39.8809380508869));
#23556=CARTESIAN_POINT('Ctrl Pts',(135.481666249792,-79.5,-40.));
#23557=CARTESIAN_POINT('Origin',(132.15,-79.75,-34.95));
#23558=CARTESIAN_POINT('',(127.978669277077,-80.,-40.));
#23559=CARTESIAN_POINT('',(128.297091469667,-79.5,-39.6145038167939));
#23560=CARTESIAN_POINT('',(127.978669277077,-80.,-40.));
#23561=CARTESIAN_POINT('',(128.132061068702,-79.5,-39.4731257714508));
#23562=CARTESIAN_POINT('Origin',(132.15,-79.5,-34.95));
#23563=CARTESIAN_POINT('',(127.8,-80.,-39.8469378186781));
#23564=CARTESIAN_POINT('',(128.132061068702,-79.5,-39.4731257714508));
#23565=CARTESIAN_POINT('Origin',(132.15,-80.,-34.95));
#23566=CARTESIAN_POINT('Ctrl Pts',(128.54404266268,-79.9563089001744,-40.4157589290663));
#23567=CARTESIAN_POINT('Ctrl Pts',(128.347413162951,-79.9832757598348,-40.2888692728855));
#23568=CARTESIAN_POINT('Ctrl Pts',(128.159138387108,-80.,-40.1490685828142));
#23569=CARTESIAN_POINT('Ctrl Pts',(127.978669277077,-80.,-40.));
#23570=CARTESIAN_POINT('Ctrl Pts',(128.635473025189,-79.8042059334496,-40.2771726193776));
#23571=CARTESIAN_POINT('Ctrl Pts',(128.444230322027,-79.8221838398899,-40.152892198886));
#23572=CARTESIAN_POINT('Ctrl Pts',(128.260687028658,-79.8333333333333,-40.0167767613686));
#23573=CARTESIAN_POINT('Ctrl Pts',(128.08481000794,-79.8333333333333,-39.8715012722646));
#23574=CARTESIAN_POINT('Ctrl Pts',(128.726903387699,-79.6521029667248,-40.1385863096888));
#23575=CARTESIAN_POINT('Ctrl Pts',(128.541047481102,-79.6610919199449,-40.0169151248865));
#23576=CARTESIAN_POINT('Ctrl Pts',(128.362235670207,-79.6666666666667,-39.8844849399229));
#23577=CARTESIAN_POINT('Ctrl Pts',(128.190950738804,-79.6666666666667,-39.7430025445293));
#23578=CARTESIAN_POINT('Ctrl Pts',(128.818333750208,-79.5,-40.));
#23579=CARTESIAN_POINT('Ctrl Pts',(128.637864640177,-79.5,-39.8809380508869));
#23580=CARTESIAN_POINT('Ctrl Pts',(128.463784311757,-79.5,-39.7521931184773));
#23581=CARTESIAN_POINT('Ctrl Pts',(128.297091469667,-79.5,-39.6145038167939));
#23582=CARTESIAN_POINT('Ctrl Pts',(127.978669277077,-80.,-40.));
#23583=CARTESIAN_POINT('Ctrl Pts',(128.159138387108,-80.,-40.1490685828142));
#23584=CARTESIAN_POINT('Ctrl Pts',(128.347413162951,-79.9832757598348,-40.2888692728855));
#23585=CARTESIAN_POINT('Ctrl Pts',(128.54404266268,-79.9563089001744,-40.4157589290663));
#23586=CARTESIAN_POINT('Ctrl Pts',(128.818333750208,-79.5,-40.));
#23587=CARTESIAN_POINT('Ctrl Pts',(128.637864640177,-79.5,-39.8809380508869));
#23588=CARTESIAN_POINT('Ctrl Pts',(128.463784311757,-79.5,-39.7521931184773));
#23589=CARTESIAN_POINT('Ctrl Pts',(128.297091469667,-79.5,-39.6145038167939));
#23590=CARTESIAN_POINT('Ctrl Pts',(127.441253216958,-79.9675621326039,-39.5015279070509));
#23591=CARTESIAN_POINT('Ctrl Pts',(127.289669164758,-79.9399237215032,-39.3421224520473));
#23592=CARTESIAN_POINT('Ctrl Pts',(127.151415155152,-79.8968591135527,-39.177273607699));
#23593=CARTESIAN_POINT('Ctrl Pts',(126.747822450792,-79.7272180669214,-38.6329022417233));
#23594=CARTESIAN_POINT('Ctrl Pts',(126.309241566678,-79.4002098919181,-37.8369213100636));
#23595=CARTESIAN_POINT('Ctrl Pts',(126.016731927051,-78.9348910451195,-36.7243946241636));
#23596=CARTESIAN_POINT('Ctrl Pts',(125.908910631778,-78.6594899573144,-35.7606410832674));
#23597=CARTESIAN_POINT('Ctrl Pts',(125.874564564028,-78.539222263838,-34.6737546688422));
#23598=CARTESIAN_POINT('Ctrl Pts',(125.959716424683,-78.8398710347191,-33.3757926529076));
#23599=CARTESIAN_POINT('Ctrl Pts',(126.19182965441,-79.2152610702774,-32.5114778246844));
#23600=CARTESIAN_POINT('Ctrl Pts',(126.605719238663,-79.6417913070752,-31.4720528940946));
#23601=CARTESIAN_POINT('Ctrl Pts',(126.956346564086,-79.879148811921,-30.9083988597416));
#23602=CARTESIAN_POINT('Ctrl Pts',(127.441253216958,-79.9675621326039,-30.3984720929491));
#23603=CARTESIAN_POINT('Ctrl Pts',(127.560835477972,-79.8117080884026,-39.3859383408092));
#23604=CARTESIAN_POINT('Ctrl Pts',(127.418051256897,-79.793325904393,-39.2365308900623));
#23605=CARTESIAN_POINT('Ctrl Pts',(127.285541376279,-79.7601112769345,-39.0809829743555));
#23606=CARTESIAN_POINT('Ctrl Pts',(126.892285897958,-79.6220738739707,-38.5639460493882));
#23607=CARTESIAN_POINT('Ctrl Pts',(126.445927355906,-79.3364444622307,-37.7985867380201));
#23608=CARTESIAN_POINT('Ctrl Pts',(126.117811983079,-78.9038208567144,-36.7085188864408));
#23609=CARTESIAN_POINT('Ctrl Pts',(125.984367943213,-78.641976174545,-35.7554810788007));
#23610=CARTESIAN_POINT('Ctrl Pts',(125.937829906089,-78.5264059109537,-34.675311760547));
#23611=CARTESIAN_POINT('Ctrl Pts',(126.053536439328,-78.815363072233,-33.3868639282635));
#23612=CARTESIAN_POINT('Ctrl Pts',(126.314374424777,-79.1645141230009,-32.5409073868163));
#23613=CARTESIAN_POINT('Ctrl Pts',(126.750190464145,-79.5498792003576,-31.5311694756925));
#23614=CARTESIAN_POINT('Ctrl Pts',(127.10393121897,-79.7535405122166,-30.9919480485029));
#23615=CARTESIAN_POINT('Ctrl Pts',(127.560835477972,-79.8117080884026,-30.5140616591908));
#23616=CARTESIAN_POINT('Ctrl Pts',(127.680417738986,-79.6558540442013,-39.2703487745675));
#23617=CARTESIAN_POINT('Ctrl Pts',(127.546538211555,-79.6465978171103,-39.1309505711611));
#23618=CARTESIAN_POINT('Ctrl Pts',(127.419530900695,-79.6234887330038,-38.9846663648664));
#23619=CARTESIAN_POINT('Ctrl Pts',(127.0371705816,-79.5164766117353,-38.4950640805886));
#23620=CARTESIAN_POINT('Ctrl Pts',(126.582405406193,-79.2725817140427,-37.7601742584199));
#23621=CARTESIAN_POINT('Ctrl Pts',(126.219183523991,-78.8725648656119,-36.6928083383561));
#23622=CARTESIAN_POINT('Ctrl Pts',(126.060127983946,-78.624209642852,-35.7503531124082));
#23623=CARTESIAN_POINT('Ctrl Pts',(126.001233420716,-78.5134310859227,-34.6771492579932));
#23624=CARTESIAN_POINT('Ctrl Pts',(126.147547546007,-78.7904336631507,-33.3978245371211));
#23625=CARTESIAN_POINT('Ctrl Pts',(126.436984817076,-79.1133706812403,-32.5702845288468));
#23626=CARTESIAN_POINT('Ctrl Pts',(126.894910069842,-79.4576583699608,-31.5904079306342));
#23627=CARTESIAN_POINT('Ctrl Pts',(127.252294250593,-79.6256082997044,-31.0756336801975));
#23628=CARTESIAN_POINT('Ctrl Pts',(127.680417738986,-79.6558540442013,-30.6296512254325));
#23629=CARTESIAN_POINT('Ctrl Pts',(127.8,-79.5,-39.1547592083257));
#23630=CARTESIAN_POINT('Ctrl Pts',(127.674920303693,-79.5,-39.0253590091761));
#23631=CARTESIAN_POINT('Ctrl Pts',(127.553657121821,-79.4867408963856,-38.8883757315229));
#23632=CARTESIAN_POINT('Ctrl Pts',(127.181634028765,-79.4113324187846,-38.4261078882536));
#23633=CARTESIAN_POINT('Ctrl Pts',(126.719091195421,-79.2088162843553,-37.7218396863763));
#23634=CARTESIAN_POINT('Ctrl Pts',(126.320263580019,-78.8414946772068,-36.6769326006333));
#23635=CARTESIAN_POINT('Ctrl Pts',(126.13558529538,-78.6066958600826,-35.7451931079415));
#23636=CARTESIAN_POINT('Ctrl Pts',(126.064498762777,-78.5006147330384,-34.6787063496979));
#23637=CARTESIAN_POINT('Ctrl Pts',(126.241367560652,-78.7659257006646,-33.408895812477));
#23638=CARTESIAN_POINT('Ctrl Pts',(126.559529587444,-79.0626237339638,-32.5997140909787));
#23639=CARTESIAN_POINT('Ctrl Pts',(127.039381295324,-79.3657462632432,-31.6495245122321));
#23640=CARTESIAN_POINT('Ctrl Pts',(127.399878905477,-79.5,-31.1591828689588));
#23641=CARTESIAN_POINT('Ctrl Pts',(127.8,-79.5,-30.7452407916743));
#23642=CARTESIAN_POINT('',(127.8,-79.5,-30.7452407916743));
#23643=CARTESIAN_POINT('',(127.441253216958,-79.9675621326039,-30.3984720929491));
#23644=CARTESIAN_POINT('',(127.8,-79.5,-30.7452407916743));
#23645=CARTESIAN_POINT('',(127.441253216958,-79.9675621326039,-39.5015279070509));
#23646=CARTESIAN_POINT('Ctrl Pts',(127.441253216958,-79.9675621326039,-30.3984720929491));
#23647=CARTESIAN_POINT('Ctrl Pts',(126.956346564086,-79.879148811921,-30.9083988597416));
#23648=CARTESIAN_POINT('Ctrl Pts',(126.605719238663,-79.6417913070752,-31.4720528940946));
#23649=CARTESIAN_POINT('Ctrl Pts',(126.19182965441,-79.2152610702774,-32.5114778246844));
#23650=CARTESIAN_POINT('Ctrl Pts',(125.959716424683,-78.8398710347191,-33.3757926529076));
#23651=CARTESIAN_POINT('Ctrl Pts',(125.874564564028,-78.539222263838,-34.6737546688422));
#23652=CARTESIAN_POINT('Ctrl Pts',(125.908910631778,-78.6594899573144,-35.7606410832674));
#23653=CARTESIAN_POINT('Ctrl Pts',(126.016731927051,-78.9348910451195,-36.7243946241636));
#23654=CARTESIAN_POINT('Ctrl Pts',(126.309241566678,-79.4002098919181,-37.8369213100636));
#23655=CARTESIAN_POINT('Ctrl Pts',(126.747822450792,-79.7272180669214,-38.6329022417233));
#23656=CARTESIAN_POINT('Ctrl Pts',(127.151415155152,-79.8968591135527,-39.177273607699));
#23657=CARTESIAN_POINT('Ctrl Pts',(127.289669164758,-79.9399237215032,-39.3421224520473));
#23658=CARTESIAN_POINT('Ctrl Pts',(127.441253216958,-79.9675621326039,-39.5015279070509));
#23659=CARTESIAN_POINT('',(127.8,-79.5,-39.1547592083257));
#23660=CARTESIAN_POINT('',(127.441253216958,-79.9675621326039,-39.5015279070509));
#23661=CARTESIAN_POINT('',(126.099985641713,-78.5536625203857,-34.9499999997728));
#23662=CARTESIAN_POINT('Ctrl Pts',(127.8,-79.5,-39.1547592083257));
#23663=CARTESIAN_POINT('Ctrl Pts',(127.674920303693,-79.5,-39.0253590091761));
#23664=CARTESIAN_POINT('Ctrl Pts',(127.553657121821,-79.4867408963856,-38.8883757315229));
#23665=CARTESIAN_POINT('Ctrl Pts',(127.181634028765,-79.4113324187846,-38.4261078882536));
#23666=CARTESIAN_POINT('Ctrl Pts',(126.719091195421,-79.2088162843553,-37.7218396863763));
#23667=CARTESIAN_POINT('Ctrl Pts',(126.320263580019,-78.8414946772068,-36.6769326006333));
#23668=CARTESIAN_POINT('Ctrl Pts',(126.135611810772,-78.6067295715856,-35.7453268834825));
#23669=CARTESIAN_POINT('Ctrl Pts',(126.100062446419,-78.5536857633005,-35.2122559673255));
#23670=CARTESIAN_POINT('Ctrl Pts',(126.099985641713,-78.5536625203857,-34.9499999997728));
#23671=CARTESIAN_POINT('Ctrl Pts',(126.099985641713,-78.5536625203857,-34.9499999997728));
#23672=CARTESIAN_POINT('Ctrl Pts',(126.099985597579,-78.5536625070295,-34.9498492984475));
#23673=CARTESIAN_POINT('Ctrl Pts',(126.099852207044,-78.5536464527083,-34.4248900938296));
#23674=CARTESIAN_POINT('Ctrl Pts',(126.241367560652,-78.7659257006646,-33.408895812477));
#23675=CARTESIAN_POINT('Ctrl Pts',(126.559529587444,-79.0626237339638,-32.5997140909787));
#23676=CARTESIAN_POINT('Ctrl Pts',(127.039381295324,-79.3657462632432,-31.6495245122321));
#23677=CARTESIAN_POINT('Ctrl Pts',(127.399878905477,-79.5,-31.1591828689588));
#23678=CARTESIAN_POINT('Ctrl Pts',(127.8,-79.5,-30.7452407916743));
#23679=CARTESIAN_POINT('Ctrl Pts',(127.8,-80.,-39.8469378186781));
#23680=CARTESIAN_POINT('Ctrl Pts',(127.675853962606,-80.,-39.7366576226328));
#23681=CARTESIAN_POINT('Ctrl Pts',(127.555667352303,-79.9884233304841,-39.6218455594625));
#23682=CARTESIAN_POINT('Ctrl Pts',(127.441253216958,-79.9675621326039,-39.5015279070509));
#23683=CARTESIAN_POINT('Ctrl Pts',(127.910687022901,-79.8333333333333,-39.7223338029357));
#23684=CARTESIAN_POINT('Ctrl Pts',(127.789699917756,-79.8333333333333,-39.614859718749));
#23685=CARTESIAN_POINT('Ctrl Pts',(127.672644263207,-79.8256155536561,-39.502910174432));
#23686=CARTESIAN_POINT('Ctrl Pts',(127.560835477972,-79.8117080884026,-39.3859383408092));
#23687=CARTESIAN_POINT('Ctrl Pts',(128.021374045802,-79.6666666666667,-39.5977297871932));
#23688=CARTESIAN_POINT('Ctrl Pts',(127.903545872906,-79.6666666666667,-39.4930618148652));
#23689=CARTESIAN_POINT('Ctrl Pts',(127.789621174111,-79.662807776828,-39.3839747894015));
#23690=CARTESIAN_POINT('Ctrl Pts',(127.680417738986,-79.6558540442013,-39.2703487745675));
#23691=CARTESIAN_POINT('Ctrl Pts',(128.132061068702,-79.5,-39.4731257714508));
#23692=CARTESIAN_POINT('Ctrl Pts',(128.017391828056,-79.5,-39.3712639109814));
#23693=CARTESIAN_POINT('Ctrl Pts',(127.906598085016,-79.5,-39.2650394043711));
#23694=CARTESIAN_POINT('Ctrl Pts',(127.8,-79.5,-39.1547592083257));
#23695=CARTESIAN_POINT('Ctrl Pts',(127.441253216958,-79.9675621326039,-39.5015279070509));
#23696=CARTESIAN_POINT('Ctrl Pts',(127.555667352303,-79.9884233304841,-39.6218455594625));
#23697=CARTESIAN_POINT('Ctrl Pts',(127.675853962606,-80.,-39.7366576226328));
#23698=CARTESIAN_POINT('Ctrl Pts',(127.8,-80.,-39.8469378186781));
#23699=CARTESIAN_POINT('Ctrl Pts',(128.132061068702,-79.5,-39.4731257714508));
#23700=CARTESIAN_POINT('Ctrl Pts',(128.017391828056,-79.5,-39.3712639109814));
#23701=CARTESIAN_POINT('Ctrl Pts',(127.906598085016,-79.5,-39.2650394043711));
#23702=CARTESIAN_POINT('Ctrl Pts',(127.8,-79.5,-39.1547592083257));
#23703=CARTESIAN_POINT('Ctrl Pts',(127.441253216958,-79.9675621326039,-30.3984720929491));
#23704=CARTESIAN_POINT('Ctrl Pts',(127.555667352303,-79.9884233304841,-30.2781544405375));
#23705=CARTESIAN_POINT('Ctrl Pts',(127.675853962606,-80.,-30.1633423773672));
#23706=CARTESIAN_POINT('Ctrl Pts',(127.8,-80.,-30.0530621813219));
#23707=CARTESIAN_POINT('Ctrl Pts',(127.560835477972,-79.8117080884026,-30.5140616591908));
#23708=CARTESIAN_POINT('Ctrl Pts',(127.672644263207,-79.8256155536561,-30.397089825568));
#23709=CARTESIAN_POINT('Ctrl Pts',(127.789699917756,-79.8333333333333,-30.285140281251));
#23710=CARTESIAN_POINT('Ctrl Pts',(127.910687022901,-79.8333333333333,-30.1776661970643));
#23711=CARTESIAN_POINT('Ctrl Pts',(127.680417738986,-79.6558540442013,-30.6296512254325));
#23712=CARTESIAN_POINT('Ctrl Pts',(127.789621174111,-79.662807776828,-30.5160252105985));
#23713=CARTESIAN_POINT('Ctrl Pts',(127.903545872906,-79.6666666666667,-30.4069381851348));
#23714=CARTESIAN_POINT('Ctrl Pts',(128.021374045802,-79.6666666666667,-30.3022702128068));
#23715=CARTESIAN_POINT('Ctrl Pts',(127.8,-79.5,-30.7452407916743));
#23716=CARTESIAN_POINT('Ctrl Pts',(127.906598085016,-79.5,-30.634960595629));
#23717=CARTESIAN_POINT('Ctrl Pts',(128.017391828056,-79.5,-30.5287360890186));
#23718=CARTESIAN_POINT('Ctrl Pts',(128.132061068702,-79.5,-30.4268742285492));
#23719=CARTESIAN_POINT('Ctrl Pts',(127.8,-80.,-30.0530621813219));
#23720=CARTESIAN_POINT('Ctrl Pts',(127.675853962606,-80.,-30.1633423773672));
#23721=CARTESIAN_POINT('Ctrl Pts',(127.555667352303,-79.9884233304841,-30.2781544405375));
#23722=CARTESIAN_POINT('Ctrl Pts',(127.441253216958,-79.9675621326039,-30.3984720929491));
#23723=CARTESIAN_POINT('Ctrl Pts',(127.8,-79.5,-30.7452407916743));
#23724=CARTESIAN_POINT('Ctrl Pts',(127.906598085016,-79.5,-30.634960595629));
#23725=CARTESIAN_POINT('Ctrl Pts',(128.017391828056,-79.5,-30.5287360890186));
#23726=CARTESIAN_POINT('Ctrl Pts',(128.132061068702,-79.5,-30.4268742285492));
#23727=CARTESIAN_POINT('Origin',(125.8,-80.,-42.));
#23728=CARTESIAN_POINT('',(127.8,-80.,-40.));
#23729=CARTESIAN_POINT('',(127.8,-80.,-21.));
#23730=CARTESIAN_POINT('',(138.1,-80.,-40.));
#23731=CARTESIAN_POINT('Origin',(127.8,-78.,-21.));
#23732=CARTESIAN_POINT('',(125.8,-78.,40.));
#23733=CARTESIAN_POINT('Origin',(127.8,-78.,40.));
#23734=CARTESIAN_POINT('',(125.8,-78.,-40.));
#23735=CARTESIAN_POINT('',(125.8,-78.,-21.));
#23736=CARTESIAN_POINT('Origin',(127.8,-78.,-40.));
#23737=CARTESIAN_POINT('Origin',(132.15,-80.,-34.95));
#23738=CARTESIAN_POINT('',(126.1,-62.,-34.95));
#23739=CARTESIAN_POINT('',(126.1,-80.,-34.95));
#23740=CARTESIAN_POINT('Origin',(132.15,-62.,-34.95));
#23741=CARTESIAN_POINT('Ctrl Pts',(172.66998797436,-54.6177973391537,-42.11123563516));
#23742=CARTESIAN_POINT('Ctrl Pts',(172.674080622603,-54.619644562519,-42.1144831050407));
#23743=CARTESIAN_POINT('Ctrl Pts',(172.678173128461,-54.6215008410306,-42.1177253206949));
#23744=CARTESIAN_POINT('Ctrl Pts',(172.682265412335,-54.6233661469982,-42.1209622367086));
#23745=CARTESIAN_POINT('Ctrl Pts',(172.89432770979,-54.5345306308824,-41.8799969243272));
#23746=CARTESIAN_POINT('Ctrl Pts',(172.898404757568,-54.5364306414694,-41.8832527980149));
#23747=CARTESIAN_POINT('Ctrl Pts',(172.902480959001,-54.5383400353523,-41.8865042916576));
#23748=CARTESIAN_POINT('Ctrl Pts',(172.906556234951,-54.540258782111,-41.8897513603237));
#23749=CARTESIAN_POINT('Ctrl Pts',(173.11866744522,-54.4512639226111,-41.6487582134943));
#23750=CARTESIAN_POINT('Ctrl Pts',(173.122728892534,-54.4532167204199,-41.6520224909892));
#23751=CARTESIAN_POINT('Ctrl Pts',(173.126788789542,-54.455179229674,-41.6552832626203));
#23752=CARTESIAN_POINT('Ctrl Pts',(173.130847057568,-54.4571514172237,-41.6585404839387));
#23753=CARTESIAN_POINT('Ctrl Pts',(173.343007180649,-54.3679972143398,-41.4175195026615));
#23754=CARTESIAN_POINT('Ctrl Pts',(173.347053027499,-54.3700027993703,-41.4207921839634));
#23755=CARTESIAN_POINT('Ctrl Pts',(173.351096620082,-54.3720184239957,-41.424062233583));
#23756=CARTESIAN_POINT('Ctrl Pts',(173.355137880184,-54.3740440523364,-41.4273296075537));
#23757=CARTESIAN_POINT('',(173.343007180649,-54.3679972143398,-41.4175195026615));
#23758=CARTESIAN_POINT('',(172.66998797436,-54.6177973391537,-42.11123563516));
#23759=CARTESIAN_POINT('Ctrl Pts',(173.343007180649,-54.3679972143398,-41.4175195026615));
#23760=CARTESIAN_POINT('Ctrl Pts',(173.11866744522,-54.4512639226111,-41.6487582134943));
#23761=CARTESIAN_POINT('Ctrl Pts',(172.89432770979,-54.5345306308824,-41.8799969243272));
#23762=CARTESIAN_POINT('Ctrl Pts',(172.66998797436,-54.6177973391537,-42.11123563516));
#23763=CARTESIAN_POINT('',(173.355137880184,-54.3740440523365,-41.4273296075537));
#23764=CARTESIAN_POINT('Ctrl Pts',(173.343007180649,-54.3679972143398,-41.4175195026615));
#23765=CARTESIAN_POINT('Ctrl Pts',(173.347053027499,-54.3700027993703,-41.4207921839634));
#23766=CARTESIAN_POINT('Ctrl Pts',(173.351096620082,-54.3720184239957,-41.424062233583));
#23767=CARTESIAN_POINT('Ctrl Pts',(173.355137880184,-54.3740440523364,-41.4273296075537));
#23768=CARTESIAN_POINT('',(172.682265412335,-54.6233661469982,-42.1209622367086));
#23769=CARTESIAN_POINT('Ctrl Pts',(173.355137880184,-54.3740440523364,-41.4273296075537));
#23770=CARTESIAN_POINT('Ctrl Pts',(173.130847057568,-54.4571514172237,-41.6585404839387));
#23771=CARTESIAN_POINT('Ctrl Pts',(172.906556234951,-54.540258782111,-41.8897513603237));
#23772=CARTESIAN_POINT('Ctrl Pts',(172.682265412335,-54.6233661469982,-42.1209622367086));
#23773=CARTESIAN_POINT('Ctrl Pts',(172.682265412346,-54.6233661470033,-42.1209622367175));
#23774=CARTESIAN_POINT('Ctrl Pts',(172.678173128469,-54.6215008410342,-42.1177253207011));
#23775=CARTESIAN_POINT('Ctrl Pts',(172.674080622608,-54.619644562521,-42.1144831050443));
#23776=CARTESIAN_POINT('Ctrl Pts',(172.669987974361,-54.6177973391542,-42.1112356351609));
#23777=CARTESIAN_POINT('Ctrl Pts',(172.682265412335,-54.6233661469982,-42.1209622367086));
#23778=CARTESIAN_POINT('Ctrl Pts',(173.215637563912,-54.8664827752239,-42.5428491125249));
#23779=CARTESIAN_POINT('Ctrl Pts',(173.745325571242,-55.2614905271195,-42.8738456760892));
#23780=CARTESIAN_POINT('Ctrl Pts',(174.217811580545,-55.9131609972939,-43.079781844656));
#23781=CARTESIAN_POINT('Ctrl Pts',(174.312192137058,-56.0793965789834,-43.1103778842156));
#23782=CARTESIAN_POINT('Ctrl Pts',(174.435796016049,-56.3890168894375,-43.1269819071719));
#23783=CARTESIAN_POINT('Ctrl Pts',(174.47235407616,-56.5277138229442,-43.1199886669764));
#23784=CARTESIAN_POINT('Ctrl Pts',(174.496492816042,-56.7264202902178,-43.0887325863734));
#23785=CARTESIAN_POINT('Ctrl Pts',(174.5,-56.7847063150805,-43.076852451079));
#23786=CARTESIAN_POINT('Ctrl Pts',(174.5,-56.8425310374202,-43.0623574561495));
#23787=CARTESIAN_POINT('Ctrl Pts',(172.906556234951,-54.540258782111,-41.8897513603237));
#23788=CARTESIAN_POINT('Ctrl Pts',(173.438158459423,-54.7903069194011,-42.3123493732582));
#23789=CARTESIAN_POINT('Ctrl Pts',(173.951777237242,-55.1979783837946,-42.6621969802207));
#23790=CARTESIAN_POINT('Ctrl Pts',(174.400091244966,-55.8634829413806,-42.897229613997));
#23791=CARTESIAN_POINT('Ctrl Pts',(174.489150256805,-56.032697189635,-42.9342422759036));
#23792=CARTESIAN_POINT('Ctrl Pts',(174.605182937368,-56.3464560071092,-42.9602413169397));
#23793=CARTESIAN_POINT('Ctrl Pts',(174.639555462911,-56.4864133676013,-42.9560967838325));
#23794=CARTESIAN_POINT('Ctrl Pts',(174.662739203426,-56.6858634968676,-42.9267868754762));
#23795=CARTESIAN_POINT('Ctrl Pts',(174.666281991153,-56.7442283004779,-42.9151689331802));
#23796=CARTESIAN_POINT('Ctrl Pts',(174.666585068858,-56.8020063133375,-42.9006926242979));
#23797=CARTESIAN_POINT('Ctrl Pts',(173.130847057568,-54.4571514172237,-41.6585404839387));
#23798=CARTESIAN_POINT('Ctrl Pts',(173.659338898785,-54.7142323226278,-42.0836859927104));
#23799=CARTESIAN_POINT('Ctrl Pts',(174.157044295027,-55.1347188176983,-42.4519992190559));
#23800=CARTESIAN_POINT('Ctrl Pts',(174.582681714858,-55.8137303528632,-42.7143006025566));
#23801=CARTESIAN_POINT('Ctrl Pts',(174.665886765686,-55.9860386883128,-42.7583769624203));
#23802=CARTESIAN_POINT('Ctrl Pts',(174.77469850772,-56.3038647001878,-42.7933478117247));
#23803=CARTESIAN_POINT('Ctrl Pts',(174.806676184536,-56.4451249038791,-42.7922907429087));
#23804=CARTESIAN_POINT('Ctrl Pts',(174.829014350795,-56.6453016466416,-42.7648116347366));
#23805=CARTESIAN_POINT('Ctrl Pts',(174.83254353756,-56.7037531597607,-42.7535060960931));
#23806=CARTESIAN_POINT('Ctrl Pts',(174.833170137715,-56.7614815892548,-42.7390277924464));
#23807=CARTESIAN_POINT('Ctrl Pts',(173.355137880184,-54.3740440523364,-41.4273296075537));
#23808=CARTESIAN_POINT('Ctrl Pts',(173.881859794296,-54.6380564668049,-41.8531862534437));
#23809=CARTESIAN_POINT('Ctrl Pts',(174.363495961026,-55.0712066743734,-42.2403505231874));
#23810=CARTESIAN_POINT('Ctrl Pts',(174.76496137928,-55.7640522969499,-42.5317483718976));
#23811=CARTESIAN_POINT('Ctrl Pts',(174.842844885433,-55.9393392989643,-42.5822413541083));
#23812=CARTESIAN_POINT('Ctrl Pts',(174.944085429039,-56.2613038178594,-42.6266072214926));
#23813=CARTESIAN_POINT('Ctrl Pts',(174.973877571286,-56.4038244485362,-42.6283988597648));
#23814=CARTESIAN_POINT('Ctrl Pts',(174.995260738178,-56.6047448532914,-42.6028659238394));
#23815=CARTESIAN_POINT('Ctrl Pts',(174.998825528713,-56.663275145158,-42.5918225781943));
#23816=CARTESIAN_POINT('Ctrl Pts',(174.999755206573,-56.7209568651721,-42.5773629605948));
#23817=CARTESIAN_POINT('',(174.999755206573,-56.7209568651721,-42.5773629605948));
#23818=CARTESIAN_POINT('Ctrl Pts',(173.355137880175,-54.374044052332,-41.4273296075466));
#23819=CARTESIAN_POINT('Ctrl Pts',(173.88185979429,-54.6380564668001,-41.8531862534394));
#23820=CARTESIAN_POINT('Ctrl Pts',(174.363495961024,-55.0712066743705,-42.2403505231862));
#23821=CARTESIAN_POINT('Ctrl Pts',(174.66758815857,-55.5960064163895,-42.4610714324983));
#23822=CARTESIAN_POINT('Ctrl Pts',(174.76496137928,-55.7640522969499,-42.5317483718976));
#23823=CARTESIAN_POINT('Ctrl Pts',(174.842844885433,-55.9393392989643,-42.5822413541083));
#23824=CARTESIAN_POINT('Ctrl Pts',(174.898252534763,-56.1155463453136,-42.6065222235573));
#23825=CARTESIAN_POINT('Ctrl Pts',(174.944085429039,-56.2613038178594,-42.6266072214926));
#23826=CARTESIAN_POINT('Ctrl Pts',(174.973877571286,-56.4038244485362,-42.6283988597648));
#23827=CARTESIAN_POINT('Ctrl Pts',(174.988900500091,-56.5449828162991,-42.6104604748416));
#23828=CARTESIAN_POINT('Ctrl Pts',(174.995260738178,-56.6047448532914,-42.6028659238394));
#23829=CARTESIAN_POINT('Ctrl Pts',(174.998825528713,-56.663275145158,-42.5918225781943));
#23830=CARTESIAN_POINT('Ctrl Pts',(174.999755206573,-56.7209568651721,-42.5773629605948));
#23831=CARTESIAN_POINT('',(174.5,-56.8425310374202,-43.0623574561495));
#23832=CARTESIAN_POINT('',(174.999755206573,-56.7209568651721,-42.5773629605948));
#23833=CARTESIAN_POINT('Ctrl Pts',(174.5,-56.8425310374202,-43.0623574561495));
#23834=CARTESIAN_POINT('Ctrl Pts',(174.5,-56.7847063150805,-43.076852451079));
#23835=CARTESIAN_POINT('Ctrl Pts',(174.496492816042,-56.7264202902178,-43.0887325863734));
#23836=CARTESIAN_POINT('Ctrl Pts',(174.47235407616,-56.5277138229442,-43.1199886669764));
#23837=CARTESIAN_POINT('Ctrl Pts',(174.435796016049,-56.3890168894375,-43.1269819071719));
#23838=CARTESIAN_POINT('Ctrl Pts',(174.312192137058,-56.0793965789834,-43.1103778842156));
#23839=CARTESIAN_POINT('Ctrl Pts',(174.217811580545,-55.9131609972939,-43.079781844656));
#23840=CARTESIAN_POINT('Ctrl Pts',(173.745325571242,-55.2614905271195,-42.8738456760892));
#23841=CARTESIAN_POINT('Ctrl Pts',(173.215637563912,-54.8664827752239,-42.5428491125249));
#23842=CARTESIAN_POINT('Ctrl Pts',(172.682265412335,-54.6233661469982,-42.1209622367086));
#23843=CARTESIAN_POINT('Ctrl Pts',(172.761788838589,-54.6513921669961,-42.1680911210267));
#23844=CARTESIAN_POINT('Ctrl Pts',(172.756002505546,-54.6497207785918,-42.165366227668));
#23845=CARTESIAN_POINT('Ctrl Pts',(172.719569461485,-54.6401760230924,-42.1505779818549));
#23846=CARTESIAN_POINT('Ctrl Pts',(172.66998797436,-54.6177973391537,-42.11123563516));
#23847=CARTESIAN_POINT('Ctrl Pts',(172.922596211878,-54.5437202426897,-41.8972936159369));
#23848=CARTESIAN_POINT('Ctrl Pts',(172.921559444571,-54.5435041843234,-41.8968224784597));
#23849=CARTESIAN_POINT('Ctrl Pts',(172.910302152746,-54.5409830080962,-41.892409256866));
#23850=CARTESIAN_POINT('Ctrl Pts',(172.89432770979,-54.5345306308824,-41.8799969243272));
#23851=CARTESIAN_POINT('Ctrl Pts',(173.083403585168,-54.4360483183833,-41.6264961108471));
#23852=CARTESIAN_POINT('Ctrl Pts',(173.087116383597,-54.4372875900551,-41.6282787292514));
#23853=CARTESIAN_POINT('Ctrl Pts',(173.101034844007,-54.4417899931,-41.6342405318772));
#23854=CARTESIAN_POINT('Ctrl Pts',(173.11866744522,-54.4512639226111,-41.6487582134943));
#23855=CARTESIAN_POINT('Ctrl Pts',(173.244210958458,-54.3283763940769,-41.3556986057572));
#23856=CARTESIAN_POINT('Ctrl Pts',(173.252673322623,-54.3310709957867,-41.3597349800431));
#23857=CARTESIAN_POINT('Ctrl Pts',(173.291767535267,-54.3425969781039,-41.3760718068883));
#23858=CARTESIAN_POINT('Ctrl Pts',(173.343007180649,-54.3679972143398,-41.4175195026615));
#23859=CARTESIAN_POINT('',(172.761788838585,-54.651392166995,-42.168091121025));
#23860=CARTESIAN_POINT('Ctrl Pts',(172.669987974309,-54.6177973391308,-42.1112356351198));
#23861=CARTESIAN_POINT('Ctrl Pts',(172.719569461453,-54.6401760230827,-42.1505779818392));
#23862=CARTESIAN_POINT('Ctrl Pts',(172.756002505533,-54.6497207785884,-42.1653662276628));
#23863=CARTESIAN_POINT('Ctrl Pts',(172.761788838586,-54.6513921669954,-42.1680911210256));
#23864=CARTESIAN_POINT('',(172.95698498009,-54.520694527064,-41.8393833818205));
#23865=CARTESIAN_POINT('Ctrl Pts',(172.761788838589,-54.6513921669961,-42.1680911210267));
#23866=CARTESIAN_POINT('Ctrl Pts',(172.826854219089,-54.6078262870188,-42.0585218746247));
#23867=CARTESIAN_POINT('Ctrl Pts',(172.89191959959,-54.5642604070414,-41.9489526282227));
#23868=CARTESIAN_POINT('Ctrl Pts',(172.95698498009,-54.5206945270641,-41.8393833818207));
#23869=CARTESIAN_POINT('',(173.244210958463,-54.3283763940785,-41.3556986057596));
#23870=CARTESIAN_POINT('Ctrl Pts',(172.95698498009,-54.5206945270641,-41.8393833818207));
#23871=CARTESIAN_POINT('Ctrl Pts',(173.052726972879,-54.456588482735,-41.6781551231329));
#23872=CARTESIAN_POINT('Ctrl Pts',(173.148468965669,-54.392482438406,-41.516926864445));
#23873=CARTESIAN_POINT('Ctrl Pts',(173.244210958458,-54.3283763940769,-41.3556986057572));
#23874=CARTESIAN_POINT('Ctrl Pts',(173.244210958458,-54.3283763940769,-41.3556986057572));
#23875=CARTESIAN_POINT('Ctrl Pts',(173.252673322623,-54.3310709957867,-41.3597349800431));
#23876=CARTESIAN_POINT('Ctrl Pts',(173.291767535267,-54.3425969781039,-41.3760718068883));
#23877=CARTESIAN_POINT('Ctrl Pts',(173.343007180649,-54.3679972143398,-41.4175195026615));
#23878=CARTESIAN_POINT('Origin',(174.75,-56.3562342901464,-41.1223792414288));
#23879=CARTESIAN_POINT('',(175.,-57.351354804662,-40.));
#23880=CARTESIAN_POINT('',(174.499999999905,-58.3461592102992,-41.3228756557483));
#23881=CARTESIAN_POINT('Ctrl Pts',(174.499999999896,-58.3461592104135,-41.3228756556501));
#23882=CARTESIAN_POINT('Ctrl Pts',(174.545769052472,-58.3053873720851,-41.270978428147));
#23883=CARTESIAN_POINT('Ctrl Pts',(174.588496139891,-58.2661562974069,-41.217054380861));
#23884=CARTESIAN_POINT('Ctrl Pts',(174.701138126955,-58.1568455611625,-41.0593011894553));
#23885=CARTESIAN_POINT('Ctrl Pts',(174.776779134635,-58.0729443622281,-40.9266860356746));
#23886=CARTESIAN_POINT('Ctrl Pts',(174.86686770893,-57.9430044328017,-40.7239686970479));
#23887=CARTESIAN_POINT('Ctrl Pts',(174.904968042358,-57.8725498634399,-40.6161672831003));
#23888=CARTESIAN_POINT('Ctrl Pts',(174.957119187857,-57.7379468702121,-40.4252008690903));
#23889=CARTESIAN_POINT('Ctrl Pts',(174.978867869175,-57.6455132484847,-40.3052809972307));
#23890=CARTESIAN_POINT('Ctrl Pts',(174.996519917819,-57.4970226095956,-40.1383691282534));
#23891=CARTESIAN_POINT('Ctrl Pts',(175.,-57.4269240433684,-40.0670009716212));
#23892=CARTESIAN_POINT('Ctrl Pts',(175.,-57.351354804662,-40.));
#23893=CARTESIAN_POINT('',(174.5,-56.8829468279694,-43.0517765313875));
#23894=CARTESIAN_POINT('Origin',(174.5,-56.3562342901464,-41.1223792414288));
#23895=CARTESIAN_POINT('',(175.,-56.7512686935136,-42.5694272088978));
#23896=CARTESIAN_POINT('',(174.5,-56.8829468279694,-43.0517765313875));
#23897=CARTESIAN_POINT('Origin',(175.,-56.3562342901464,-41.1223792414288));
#23898=CARTESIAN_POINT('Ctrl Pts',(174.5,-56.8425310374202,-43.0623574561495));
#23899=CARTESIAN_POINT('Ctrl Pts',(174.5,-56.8560393157734,-43.0589713192462));
#23900=CARTESIAN_POINT('Ctrl Pts',(174.5,-56.8695122257409,-43.0554440878163));
#23901=CARTESIAN_POINT('Ctrl Pts',(174.5,-56.8829468279694,-43.0517765313875));
#23902=CARTESIAN_POINT('Ctrl Pts',(174.666585068858,-56.8020063133375,-42.9006926242979));
#23903=CARTESIAN_POINT('Ctrl Pts',(174.666639498249,-56.8143888954835,-42.8975886395879));
#23904=CARTESIAN_POINT('Ctrl Pts',(174.666666666667,-56.8267390644414,-42.8943553506173));
#23905=CARTESIAN_POINT('Ctrl Pts',(174.666666666667,-56.8390541164841,-42.890993423891));
#23906=CARTESIAN_POINT('Ctrl Pts',(174.833170137715,-56.7614815892548,-42.7390277924464));
#23907=CARTESIAN_POINT('Ctrl Pts',(174.833278996499,-56.7727384751935,-42.7362059599296));
#23908=CARTESIAN_POINT('Ctrl Pts',(174.833333333333,-56.7839659031418,-42.7332666134184));
#23909=CARTESIAN_POINT('Ctrl Pts',(174.833333333333,-56.7951614049989,-42.7302103163944));
#23910=CARTESIAN_POINT('Ctrl Pts',(174.999755206573,-56.7209568651721,-42.5773629605948));
#23911=CARTESIAN_POINT('Ctrl Pts',(174.999918494748,-56.7310880549036,-42.5748232802713));
#23912=CARTESIAN_POINT('Ctrl Pts',(175.,-56.7411927418423,-42.5721778762194));
#23913=CARTESIAN_POINT('Ctrl Pts',(175.,-56.7512686935137,-42.5694272088978));
#23914=CARTESIAN_POINT('Ctrl Pts',(174.5,-56.8829468279694,-43.0517765313875));
#23915=CARTESIAN_POINT('Ctrl Pts',(174.5,-56.8695122257409,-43.0554440878163));
#23916=CARTESIAN_POINT('Ctrl Pts',(174.5,-56.8560393157734,-43.0589713192462));
#23917=CARTESIAN_POINT('Ctrl Pts',(174.5,-56.8425310374202,-43.0623574561495));
#23918=CARTESIAN_POINT('Ctrl Pts',(174.999755206573,-56.7209568651721,-42.5773629605948));
#23919=CARTESIAN_POINT('Ctrl Pts',(174.999918494748,-56.7310880549036,-42.5748232802713));
#23920=CARTESIAN_POINT('Ctrl Pts',(175.,-56.7411927418423,-42.5721778762194));
#23921=CARTESIAN_POINT('Ctrl Pts',(175.,-56.7512686935137,-42.5694272088978));
#23922=CARTESIAN_POINT('Ctrl Pts',(172.761788838585,-54.651392166995,-42.168091121025));
#23923=CARTESIAN_POINT('Ctrl Pts',(172.841192559056,-54.574303158249,-42.0424115797416));
#23924=CARTESIAN_POINT('Ctrl Pts',(172.920596279528,-54.5111710705365,-41.908178056654));
#23925=CARTESIAN_POINT('Ctrl Pts',(173.,-54.463528575122,-41.7686493678573));
#23926=CARTESIAN_POINT('Ctrl Pts',(172.922596211877,-54.5437202426895,-41.8972936159365));
#23927=CARTESIAN_POINT('Ctrl Pts',(172.948533142216,-54.5068055874631,-41.859694919166));
#23928=CARTESIAN_POINT('Ctrl Pts',(172.97426662197,-54.4797095101407,-41.8160378311823));
#23929=CARTESIAN_POINT('Ctrl Pts',(173.,-54.463528575122,-41.7686493678573));
#23930=CARTESIAN_POINT('Ctrl Pts',(173.08340358517,-54.436048318384,-41.6264961108481));
#23931=CARTESIAN_POINT('Ctrl Pts',(173.055873725375,-54.4393080166772,-41.6769782585905));
#23932=CARTESIAN_POINT('Ctrl Pts',(173.027936964413,-54.4482479497449,-41.7238976057107));
#23933=CARTESIAN_POINT('Ctrl Pts',(173.,-54.463528575122,-41.7686493678573));
#23934=CARTESIAN_POINT('Ctrl Pts',(173.244210958463,-54.3283763940785,-41.3556986057596));
#23935=CARTESIAN_POINT('Ctrl Pts',(173.163214308534,-54.3718104458914,-41.494261598015));
#23936=CARTESIAN_POINT('Ctrl Pts',(173.081607306855,-54.4167863893491,-41.631757380239));
#23937=CARTESIAN_POINT('Ctrl Pts',(173.,-54.463528575122,-41.7686493678573));
#23938=CARTESIAN_POINT('',(173.,-54.463528575122,-41.7686493678573));
#23939=CARTESIAN_POINT('Ctrl Pts',(172.761788838585,-54.651392166995,-42.168091121025));
#23940=CARTESIAN_POINT('Ctrl Pts',(172.841192559056,-54.574303158249,-42.0424115797416));
#23941=CARTESIAN_POINT('Ctrl Pts',(172.920596279528,-54.5111710705365,-41.908178056654));
#23942=CARTESIAN_POINT('Ctrl Pts',(173.,-54.463528575122,-41.7686493678573));
#23943=CARTESIAN_POINT('Ctrl Pts',(173.,-54.463528575122,-41.7686493678573));
#23944=CARTESIAN_POINT('Ctrl Pts',(173.081607306855,-54.4167863893491,-41.631757380239));
#23945=CARTESIAN_POINT('Ctrl Pts',(173.163214308534,-54.3718104458914,-41.494261598015));
#23946=CARTESIAN_POINT('Ctrl Pts',(173.244210958463,-54.3283763940785,-41.3556986057596));
#23947=CARTESIAN_POINT('Origin',(125.8,-56.3562342901464,-41.1223792414288));
#23948=CARTESIAN_POINT('',(173.,-58.153393661244,-42.));
#23949=CARTESIAN_POINT('Ctrl Pts',(174.499999999851,-58.3461592103039,-41.3228756557013));
#23950=CARTESIAN_POINT('Ctrl Pts',(174.461424720572,-58.3417521272735,-41.3666159110033));
#23951=CARTESIAN_POINT('Ctrl Pts',(174.420873583764,-58.3360427437949,-41.4087347797137));
#23952=CARTESIAN_POINT('Ctrl Pts',(174.256201391015,-58.3101344177017,-41.5653968322566));
#23953=CARTESIAN_POINT('Ctrl Pts',(174.118673603566,-58.2827371839977,-41.6665038929614));
#23954=CARTESIAN_POINT('Ctrl Pts',(173.822610223296,-58.2285507903109,-41.8308404000116));
#23955=CARTESIAN_POINT('Ctrl Pts',(173.663743266442,-58.2018772085049,-41.8942257523251));
#23956=CARTESIAN_POINT('Ctrl Pts',(173.335981739516,-58.164172163974,-41.9788285866254));
#23957=CARTESIAN_POINT('Ctrl Pts',(173.167046229782,-58.1533936609661,-42.));
#23958=CARTESIAN_POINT('Ctrl Pts',(173.,-58.1533936609661,-42.));
#23959=CARTESIAN_POINT('',(160.,-58.153393661244,-42.));
#23960=CARTESIAN_POINT('',(125.8,-58.153393661244,-42.));
#23961=CARTESIAN_POINT('',(162.,-55.5753783097334,-42.9636461796681));
#23962=CARTESIAN_POINT('Ctrl Pts',(160.,-58.1533936622468,-41.9999999973774));
#23963=CARTESIAN_POINT('Ctrl Pts',(160.022635178212,-58.1533936622468,-41.9999999973774));
#23964=CARTESIAN_POINT('Ctrl Pts',(160.045231132923,-58.151516657946,-42.0038756670436));
#23965=CARTESIAN_POINT('Ctrl Pts',(160.096465139443,-58.1432332860682,-42.0205631325354));
#23966=CARTESIAN_POINT('Ctrl Pts',(160.126719309599,-58.1360093928662,-42.0350714541553));
#23967=CARTESIAN_POINT('Ctrl Pts',(160.22848683334,-58.1032750521955,-42.0970139060601));
#23968=CARTESIAN_POINT('Ctrl Pts',(160.306498809967,-58.069336621093,-42.15765241691));
#23969=CARTESIAN_POINT('Ctrl Pts',(160.605864004126,-57.9112848828316,-42.3968423684444));
#23970=CARTESIAN_POINT('Ctrl Pts',(160.90925083337,-57.7038897039527,-42.6497063660358));
#23971=CARTESIAN_POINT('Ctrl Pts',(161.417356253422,-57.1425466698487,-42.9804088994022));
#23972=CARTESIAN_POINT('Ctrl Pts',(161.590327339247,-56.8907533740651,-43.0674615146063));
#23973=CARTESIAN_POINT('Ctrl Pts',(161.824128439415,-56.4279006785006,-43.1315274209591));
#23974=CARTESIAN_POINT('Ctrl Pts',(161.904779002332,-56.2130118801458,-43.129561872258));
#23975=CARTESIAN_POINT('Ctrl Pts',(161.983794647709,-55.8514686747774,-43.0631018472003));
#23976=CARTESIAN_POINT('Ctrl Pts',(162.,-55.7108001207802,-43.0210767068981));
#23977=CARTESIAN_POINT('Ctrl Pts',(162.,-55.5753783097334,-42.9636461796681));
#23978=CARTESIAN_POINT('',(162.,-54.463528575122,-41.7686493678573));
#23979=CARTESIAN_POINT('Origin',(162.,-56.3562342901464,-41.1223792414288));
#23980=CARTESIAN_POINT('',(125.8,-54.463528575122,-41.7686493678573));
#23981=CARTESIAN_POINT('Ctrl Pts',(172.669987974283,-54.6177973391178,42.1112356350969));
#23982=CARTESIAN_POINT('Ctrl Pts',(172.69185108023,-54.6276652871456,42.1285837612678));
#23983=CARTESIAN_POINT('Ctrl Pts',(172.73830709009,-54.644963812684,42.1577290355036));
#23984=CARTESIAN_POINT('Ctrl Pts',(172.759754438233,-54.6508063297863,42.1671363033964));
#23985=CARTESIAN_POINT('Ctrl Pts',(172.762221454692,-54.6515169577276,42.1682945422782));
#23986=CARTESIAN_POINT('Ctrl Pts',(172.894327709765,-54.5345306308711,41.8799969243054));
#23987=CARTESIAN_POINT('Ctrl Pts',(172.901371688395,-54.5373758259908,41.8854701796426));
#23988=CARTESIAN_POINT('Ctrl Pts',(172.916128759429,-54.5422404819325,41.8945407469037));
#23989=CARTESIAN_POINT('Ctrl Pts',(172.922366122002,-54.5436871571058,41.8971924349675));
#23990=CARTESIAN_POINT('Ctrl Pts',(172.922663031267,-54.5437329784674,41.8973236981606));
#23991=CARTESIAN_POINT('Ctrl Pts',(173.118667445246,-54.4512639226244,41.6487582135139));
#23992=CARTESIAN_POINT('Ctrl Pts',(173.11089229656,-54.4470863648361,41.6423565980175));
#23993=CARTESIAN_POINT('Ctrl Pts',(173.093950428767,-54.4395171511809,41.6313524583038));
#23994=CARTESIAN_POINT('Ctrl Pts',(173.08497780577,-54.4365679844252,41.6272485665385));
#23995=CARTESIAN_POINT('Ctrl Pts',(173.083104607842,-54.4359489992072,41.6263528540431));
#23996=CARTESIAN_POINT('Ctrl Pts',(173.343007180728,-54.3679972143777,41.4175195027224));
#23997=CARTESIAN_POINT('Ctrl Pts',(173.320412904725,-54.3567969036813,41.3992430163923));
#23998=CARTESIAN_POINT('Ctrl Pts',(173.271772098106,-54.3367938204293,41.368164169704));
#23999=CARTESIAN_POINT('Ctrl Pts',(173.247589489539,-54.3294488117447,41.3573046981095));
#24000=CARTESIAN_POINT('Ctrl Pts',(173.243546184418,-54.328165019947,41.3553820099255));
#24001=CARTESIAN_POINT('',(173.343007180728,-54.3679972143777,41.4175195027224));
#24002=CARTESIAN_POINT('',(172.669987974283,-54.6177973391178,42.1112356350969));
#24003=CARTESIAN_POINT('Ctrl Pts',(173.343007180728,-54.3679972143777,41.4175195027224));
#24004=CARTESIAN_POINT('Ctrl Pts',(173.118667445246,-54.4512639226244,41.6487582135139));
#24005=CARTESIAN_POINT('Ctrl Pts',(172.894327709765,-54.5345306308711,41.8799969243054));
#24006=CARTESIAN_POINT('Ctrl Pts',(172.669987974283,-54.6177973391178,42.1112356350969));
#24007=CARTESIAN_POINT('',(173.243546184425,-54.3281650199493,41.3553820099289));
#24008=CARTESIAN_POINT('Ctrl Pts',(173.343007180728,-54.3679972143777,41.4175195027224));
#24009=CARTESIAN_POINT('Ctrl Pts',(173.320412904725,-54.3567969036813,41.3992430163923));
#24010=CARTESIAN_POINT('Ctrl Pts',(173.271772098106,-54.3367938204293,41.368164169704));
#24011=CARTESIAN_POINT('Ctrl Pts',(173.247589489539,-54.3294488117447,41.3573046981095));
#24012=CARTESIAN_POINT('Ctrl Pts',(173.243546184418,-54.328165019947,41.3553820099255));
#24013=CARTESIAN_POINT('',(172.943915700111,-54.5294555245376,41.8614299246169));
#24014=CARTESIAN_POINT('Ctrl Pts',(173.243546184418,-54.328165019947,41.3553820099255));
#24015=CARTESIAN_POINT('Ctrl Pts',(173.143669356316,-54.3952618548106,41.5240646481561));
#24016=CARTESIAN_POINT('Ctrl Pts',(173.043792528214,-54.4623586896742,41.6927472863866));
#24017=CARTESIAN_POINT('Ctrl Pts',(172.943915700112,-54.5294555245378,41.8614299246172));
#24018=CARTESIAN_POINT('',(172.762221454686,-54.6515169577261,42.1682945422757));
#24019=CARTESIAN_POINT('Ctrl Pts',(172.943915700112,-54.5294555245378,41.8614299246172));
#24020=CARTESIAN_POINT('Ctrl Pts',(172.883350951638,-54.5701426689344,41.9637181305042));
#24021=CARTESIAN_POINT('Ctrl Pts',(172.822786203165,-54.610829813331,42.0660063363912));
#24022=CARTESIAN_POINT('Ctrl Pts',(172.762221454692,-54.6515169577276,42.1682945422782));
#24023=CARTESIAN_POINT('Ctrl Pts',(172.762221454692,-54.6515169577276,42.1682945422782));
#24024=CARTESIAN_POINT('Ctrl Pts',(172.759754438233,-54.6508063297863,42.1671363033964));
#24025=CARTESIAN_POINT('Ctrl Pts',(172.73830709009,-54.644963812684,42.1577290355036));
#24026=CARTESIAN_POINT('Ctrl Pts',(172.69185108023,-54.6276652871456,42.1285837612678));
#24027=CARTESIAN_POINT('Ctrl Pts',(172.669987974283,-54.6177973391178,42.1112356350969));
#24028=CARTESIAN_POINT('Ctrl Pts',(172.682265412035,-54.6233661468611,42.1209622364707));
#24029=CARTESIAN_POINT('Ctrl Pts',(172.678173128254,-54.6215008409364,42.1177253205304));
#24030=CARTESIAN_POINT('Ctrl Pts',(172.67408062253,-54.6196445624853,42.1144831049818));
#24031=CARTESIAN_POINT('Ctrl Pts',(172.669987974283,-54.6177973391178,42.1112356350969));
#24032=CARTESIAN_POINT('Ctrl Pts',(172.906556234659,-54.5402587819729,41.8897513600897));
#24033=CARTESIAN_POINT('Ctrl Pts',(172.902480958804,-54.5383400352597,41.8865042914994));
#24034=CARTESIAN_POINT('Ctrl Pts',(172.89840475748,-54.5364306414273,41.8832527979434));
#24035=CARTESIAN_POINT('Ctrl Pts',(172.894327709765,-54.5345306308711,41.8799969243054));
#24036=CARTESIAN_POINT('Ctrl Pts',(173.130847057282,-54.4571514170847,41.6585404837086));
#24037=CARTESIAN_POINT('Ctrl Pts',(173.126788789354,-54.455179229583,41.6552832624683));
#24038=CARTESIAN_POINT('Ctrl Pts',(173.12272889243,-54.4532167203693,41.6520224909049));
#24039=CARTESIAN_POINT('Ctrl Pts',(173.118667445246,-54.4512639226244,41.6487582135139));
#24040=CARTESIAN_POINT('Ctrl Pts',(173.355137879905,-54.3740440521965,41.4273296073276));
#24041=CARTESIAN_POINT('Ctrl Pts',(173.351096619904,-54.3720184239062,41.4240622334373));
#24042=CARTESIAN_POINT('Ctrl Pts',(173.34705302738,-54.3700027993113,41.4207921838665));
#24043=CARTESIAN_POINT('Ctrl Pts',(173.343007180728,-54.3679972143777,41.4175195027224));
#24044=CARTESIAN_POINT('',(172.682265412035,-54.6233661468611,42.1209622364707));
#24045=CARTESIAN_POINT('Ctrl Pts',(172.669987974283,-54.6177973391178,42.1112356350969));
#24046=CARTESIAN_POINT('Ctrl Pts',(172.673021360544,-54.6191664628845,42.1136425926307));
#24047=CARTESIAN_POINT('Ctrl Pts',(172.676054668529,-54.6205405610396,42.1160466637328));
#24048=CARTESIAN_POINT('Ctrl Pts',(172.680147061872,-54.6224011921202,42.119286319929));
#24049=CARTESIAN_POINT('Ctrl Pts',(172.681206244385,-54.6228833671227,42.1201244557024));
#24050=CARTESIAN_POINT('Ctrl Pts',(172.682265412038,-54.6233661468624,42.1209622364729));
#24051=CARTESIAN_POINT('',(173.355137879905,-54.3740440521965,41.4273296073276));
#24052=CARTESIAN_POINT('Ctrl Pts',(173.355137879905,-54.3740440521965,41.4273296073276));
#24053=CARTESIAN_POINT('Ctrl Pts',(173.130847057282,-54.4571514170847,41.6585404837086));
#24054=CARTESIAN_POINT('Ctrl Pts',(172.906556234659,-54.5402587819729,41.8897513600897));
#24055=CARTESIAN_POINT('Ctrl Pts',(172.682265412035,-54.6233661468611,42.1209622364707));
#24056=CARTESIAN_POINT('Ctrl Pts',(173.355137879905,-54.3740440521965,41.4273296073277));
#24057=CARTESIAN_POINT('Ctrl Pts',(173.354091918257,-54.3735197777119,41.4264839434067));
#24058=CARTESIAN_POINT('Ctrl Pts',(173.353045800347,-54.3729961733496,41.4256381002379));
#24059=CARTESIAN_POINT('Ctrl Pts',(173.349003338184,-54.3709757257882,41.4223693442523));
#24060=CARTESIAN_POINT('Ctrl Pts',(173.346005878614,-54.3694837124628,41.4199451463202));
#24061=CARTESIAN_POINT('Ctrl Pts',(173.343007180728,-54.3679972143777,41.4175195027224));
#24062=CARTESIAN_POINT('Ctrl Pts',(174.5,-56.8425310374202,43.0623574561495));
#24063=CARTESIAN_POINT('Ctrl Pts',(174.5,-56.7847063150805,43.076852451079));
#24064=CARTESIAN_POINT('Ctrl Pts',(174.496496807675,-56.726424924067,43.0887347398924));
#24065=CARTESIAN_POINT('Ctrl Pts',(174.472374635079,-56.5277343616924,43.1200003168992));
#24066=CARTESIAN_POINT('Ctrl Pts',(174.435819579446,-56.3890515008375,43.1269934025858));
#24067=CARTESIAN_POINT('Ctrl Pts',(174.312313762606,-56.0795034004758,43.1104492732835));
#24068=CARTESIAN_POINT('Ctrl Pts',(174.217660640189,-55.9131275752079,43.079676621033));
#24069=CARTESIAN_POINT('Ctrl Pts',(173.942183918571,-55.532355907991,42.959817332661));
#24070=CARTESIAN_POINT('Ctrl Pts',(173.741291684645,-55.3264070661798,42.8511994836494));
#24071=CARTESIAN_POINT('Ctrl Pts',(173.265184684464,-54.9358232466634,42.5556672491669));
#24072=CARTESIAN_POINT('Ctrl Pts',(172.974300346141,-54.7564787367862,42.3519561225039));
#24073=CARTESIAN_POINT('Ctrl Pts',(172.682265412035,-54.6233661468611,42.1209622364707));
#24074=CARTESIAN_POINT('Ctrl Pts',(174.666585068858,-56.8020063133375,42.9006926242979));
#24075=CARTESIAN_POINT('Ctrl Pts',(174.666275223311,-56.7442298071472,42.9151773304318));
#24076=CARTESIAN_POINT('Ctrl Pts',(174.662752482402,-56.6858660630933,42.9267775056715));
#24077=CARTESIAN_POINT('Ctrl Pts',(174.639550570743,-56.4864395729044,42.9561400122007));
#24078=CARTESIAN_POINT('Ctrl Pts',(174.605246474233,-56.3464817138786,42.9602032167489));
#24079=CARTESIAN_POINT('Ctrl Pts',(174.48920343284,-56.0328192806896,42.9343985844122));
#24080=CARTESIAN_POINT('Ctrl Pts',(174.400067029284,-55.8634208915866,42.8969672866207));
#24081=CARTESIAN_POINT('Ctrl Pts',(174.138352490568,-55.4746412639251,42.7605554030612));
#24082=CARTESIAN_POINT('Ctrl Pts',(173.945647760261,-55.2634045021095,42.6421788065363));
#24083=CARTESIAN_POINT('Ctrl Pts',(173.483301232679,-54.8620390670757,42.3305939920553));
#24084=CARTESIAN_POINT('Ctrl Pts',(173.197434721993,-54.6771744507838,42.1213898659891));
#24085=CARTESIAN_POINT('Ctrl Pts',(172.906556234659,-54.5402587819729,41.8897513600897));
#24086=CARTESIAN_POINT('Ctrl Pts',(174.833170137715,-56.7614815892548,42.7390277924464));
#24087=CARTESIAN_POINT('Ctrl Pts',(174.832550305402,-56.7037516530913,42.7534976988416));
#24088=CARTESIAN_POINT('Ctrl Pts',(174.829009502811,-56.645308594404,42.7648244865385));
#24089=CARTESIAN_POINT('Ctrl Pts',(174.806721608943,-56.4451411607773,42.7922706501334));
#24090=CARTESIAN_POINT('Ctrl Pts',(174.774691045787,-56.303909416709,42.7933951250364));
#24091=CARTESIAN_POINT('Ctrl Pts',(174.666060639652,-55.9861389428714,42.7583804524309));
#24092=CARTESIAN_POINT('Ctrl Pts',(174.58251031073,-55.8137112952995,42.7142096468544));
#24093=CARTESIAN_POINT('Ctrl Pts',(174.334441347141,-55.4169347605697,42.561393695158));
#24094=CARTESIAN_POINT('Ctrl Pts',(174.149980589901,-55.2004048120655,42.4331810744332));
#24095=CARTESIAN_POINT('Ctrl Pts',(173.701401705862,-54.7882591897525,42.1055501983502));
#24096=CARTESIAN_POINT('Ctrl Pts',(173.420397262025,-54.5979019067952,41.8910633003636));
#24097=CARTESIAN_POINT('Ctrl Pts',(173.130847057282,-54.4571514170847,41.6585404837086));
#24098=CARTESIAN_POINT('Ctrl Pts',(174.999755206573,-56.7209568651721,42.5773629605948));
#24099=CARTESIAN_POINT('Ctrl Pts',(174.998825528713,-56.663275145158,42.5918225781943));
#24100=CARTESIAN_POINT('Ctrl Pts',(174.995265177538,-56.6047497334302,42.6028672523175));
#24101=CARTESIAN_POINT('Ctrl Pts',(174.973897544607,-56.4038463719893,42.6284103454349));
#24102=CARTESIAN_POINT('Ctrl Pts',(174.944117940575,-56.2613396297502,42.6266049391994));
#24103=CARTESIAN_POINT('Ctrl Pts',(174.842950309886,-55.9394548230851,42.5823297635595));
#24104=CARTESIAN_POINT('Ctrl Pts',(174.764916699824,-55.7640046116782,42.5315003124422));
#24105=CARTESIAN_POINT('Ctrl Pts',(174.530609919138,-55.3592201165037,42.3621317655582));
#24106=CARTESIAN_POINT('Ctrl Pts',(174.354336665516,-55.1374022479952,42.2241603973201));
#24107=CARTESIAN_POINT('Ctrl Pts',(173.919518254077,-54.7144750101649,41.8804769412387));
#24108=CARTESIAN_POINT('Ctrl Pts',(173.643531637876,-54.5185976207928,41.6604970438488));
#24109=CARTESIAN_POINT('Ctrl Pts',(173.355137879905,-54.3740440521965,41.4273296073276));
#24110=CARTESIAN_POINT('',(174.5,-56.8425310374202,43.0623574561495));
#24111=CARTESIAN_POINT('Ctrl Pts',(172.682265412035,-54.6233661468611,42.1209622364707));
#24112=CARTESIAN_POINT('Ctrl Pts',(172.974300346141,-54.7564787367862,42.3519561225039));
#24113=CARTESIAN_POINT('Ctrl Pts',(173.265184684464,-54.9358232466634,42.5556672491669));
#24114=CARTESIAN_POINT('Ctrl Pts',(173.741291684645,-55.3264070661798,42.8511994836494));
#24115=CARTESIAN_POINT('Ctrl Pts',(173.942183918571,-55.532355907991,42.959817332661));
#24116=CARTESIAN_POINT('Ctrl Pts',(174.217660640189,-55.9131275752079,43.079676621033));
#24117=CARTESIAN_POINT('Ctrl Pts',(174.312313762606,-56.0795034004758,43.1104492732835));
#24118=CARTESIAN_POINT('Ctrl Pts',(174.435819579446,-56.3890515008375,43.1269934025858));
#24119=CARTESIAN_POINT('Ctrl Pts',(174.472374635079,-56.5277343616924,43.1200003168992));
#24120=CARTESIAN_POINT('Ctrl Pts',(174.496496807675,-56.726424924067,43.0887347398924));
#24121=CARTESIAN_POINT('Ctrl Pts',(174.5,-56.7847063150805,43.076852451079));
#24122=CARTESIAN_POINT('Ctrl Pts',(174.5,-56.8425310374202,43.0623574561495));
#24123=CARTESIAN_POINT('',(174.999755206573,-56.7209568651721,42.5773629605948));
#24124=CARTESIAN_POINT('',(174.5,-56.8425310374202,43.0623574561495));
#24125=CARTESIAN_POINT('Ctrl Pts',(174.999755206573,-56.7209568651721,42.5773629605948));
#24126=CARTESIAN_POINT('Ctrl Pts',(174.998825528713,-56.663275145158,42.5918225781943));
#24127=CARTESIAN_POINT('Ctrl Pts',(174.995265177538,-56.6047497334302,42.6028672523175));
#24128=CARTESIAN_POINT('Ctrl Pts',(174.973897544607,-56.4038463719893,42.6284103454349));
#24129=CARTESIAN_POINT('Ctrl Pts',(174.944117940575,-56.2613396297502,42.6266049391994));
#24130=CARTESIAN_POINT('Ctrl Pts',(174.842950309886,-55.9394548230851,42.5823297635595));
#24131=CARTESIAN_POINT('Ctrl Pts',(174.764916699824,-55.7640046116782,42.5315003124422));
#24132=CARTESIAN_POINT('Ctrl Pts',(174.530609919138,-55.3592201165037,42.3621317655582));
#24133=CARTESIAN_POINT('Ctrl Pts',(174.354336665516,-55.1374022479952,42.2241603973201));
#24134=CARTESIAN_POINT('Ctrl Pts',(173.919518254077,-54.7144750101649,41.8804769412387));
#24135=CARTESIAN_POINT('Ctrl Pts',(173.643531637876,-54.5185976207928,41.6604970438488));
#24136=CARTESIAN_POINT('Ctrl Pts',(173.355137879905,-54.3740440521965,41.4273296073276));
#24137=CARTESIAN_POINT('Origin',(174.75,-56.3562342901464,41.1223792414288));
#24138=CARTESIAN_POINT('',(175.,-56.7512686935136,42.5694272088978));
#24139=CARTESIAN_POINT('',(174.5,-56.8829468279694,43.0517765313875));
#24140=CARTESIAN_POINT('',(175.,-56.7512686935136,42.5694272088978));
#24141=CARTESIAN_POINT('',(174.499999999905,-58.3461592102992,41.3228756557482));
#24142=CARTESIAN_POINT('Origin',(174.5,-56.3562342901464,41.1223792414288));
#24143=CARTESIAN_POINT('',(175.,-57.351354804662,40.));
#24144=CARTESIAN_POINT('Ctrl Pts',(175.,-57.351354804662,40.));
#24145=CARTESIAN_POINT('Ctrl Pts',(175.,-57.4269240433685,40.0670009716211));
#24146=CARTESIAN_POINT('Ctrl Pts',(174.996519917819,-57.4970226095956,40.1383691282534));
#24147=CARTESIAN_POINT('Ctrl Pts',(174.978867869175,-57.6455132484847,40.3052809972307));
#24148=CARTESIAN_POINT('Ctrl Pts',(174.957119187857,-57.7379468702121,40.4252008690902));
#24149=CARTESIAN_POINT('Ctrl Pts',(174.904968042358,-57.87254986344,40.6161672831003));
#24150=CARTESIAN_POINT('Ctrl Pts',(174.86686770893,-57.9430044328017,40.7239686970479));
#24151=CARTESIAN_POINT('Ctrl Pts',(174.776779134635,-58.0729443622281,40.9266860356746));
#24152=CARTESIAN_POINT('Ctrl Pts',(174.701138126955,-58.1568455611626,41.0593011894553));
#24153=CARTESIAN_POINT('Ctrl Pts',(174.588496139891,-58.2661562974069,41.217054380861));
#24154=CARTESIAN_POINT('Ctrl Pts',(174.545769052472,-58.3053873720851,41.270978428147));
#24155=CARTESIAN_POINT('Ctrl Pts',(174.499999999896,-58.3461592104135,41.3228756556501));
#24156=CARTESIAN_POINT('Origin',(175.,-56.3562342901464,41.1223792414288));
#24157=CARTESIAN_POINT('Ctrl Pts',(174.5,-56.8829468279694,43.0517765313875));
#24158=CARTESIAN_POINT('Ctrl Pts',(174.5,-56.8695122257409,43.0554440878163));
#24159=CARTESIAN_POINT('Ctrl Pts',(174.5,-56.8560393157734,43.0589713192462));
#24160=CARTESIAN_POINT('Ctrl Pts',(174.5,-56.8425310374202,43.0623574561495));
#24161=CARTESIAN_POINT('Ctrl Pts',(174.666666666667,-56.8390541164841,42.890993423891));
#24162=CARTESIAN_POINT('Ctrl Pts',(174.666666666667,-56.8267390644414,42.8943553506173));
#24163=CARTESIAN_POINT('Ctrl Pts',(174.666639498249,-56.8143888954835,42.8975886395879));
#24164=CARTESIAN_POINT('Ctrl Pts',(174.666585068858,-56.8020063133375,42.9006926242979));
#24165=CARTESIAN_POINT('Ctrl Pts',(174.833333333333,-56.7951614049989,42.7302103163944));
#24166=CARTESIAN_POINT('Ctrl Pts',(174.833333333333,-56.7839659031418,42.7332666134184));
#24167=CARTESIAN_POINT('Ctrl Pts',(174.833278996499,-56.7727384751935,42.7362059599296));
#24168=CARTESIAN_POINT('Ctrl Pts',(174.833170137715,-56.7614815892548,42.7390277924464));
#24169=CARTESIAN_POINT('Ctrl Pts',(175.,-56.7512686935137,42.5694272088978));
#24170=CARTESIAN_POINT('Ctrl Pts',(175.,-56.7411927418423,42.5721778762194));
#24171=CARTESIAN_POINT('Ctrl Pts',(174.999918494748,-56.7310880549036,42.5748232802713));
#24172=CARTESIAN_POINT('Ctrl Pts',(174.999755206573,-56.7209568651721,42.5773629605948));
#24173=CARTESIAN_POINT('Ctrl Pts',(175.,-56.7512686935137,42.5694272088978));
#24174=CARTESIAN_POINT('Ctrl Pts',(175.,-56.7411927418423,42.5721778762194));
#24175=CARTESIAN_POINT('Ctrl Pts',(174.999918494748,-56.7310880549036,42.5748232802713));
#24176=CARTESIAN_POINT('Ctrl Pts',(174.999755206573,-56.7209568651721,42.5773629605948));
#24177=CARTESIAN_POINT('Ctrl Pts',(174.5,-56.8425310374202,43.0623574561495));
#24178=CARTESIAN_POINT('Ctrl Pts',(174.5,-56.8560393157734,43.0589713192462));
#24179=CARTESIAN_POINT('Ctrl Pts',(174.5,-56.8695122257409,43.0554440878163));
#24180=CARTESIAN_POINT('Ctrl Pts',(174.5,-56.8829468279694,43.0517765313875));
#24181=CARTESIAN_POINT('Ctrl Pts',(173.243546184425,-54.3281650199493,41.3553820099289));
#24182=CARTESIAN_POINT('Ctrl Pts',(173.162767797901,-54.3716994765092,41.4940379614493));
#24183=CARTESIAN_POINT('Ctrl Pts',(173.081384049463,-54.41674640089,41.6316402676231));
#24184=CARTESIAN_POINT('Ctrl Pts',(173.,-54.463528575122,41.7686493678573));
#24185=CARTESIAN_POINT('Ctrl Pts',(173.083104607845,-54.4359489992082,41.6263528540445));
#24186=CARTESIAN_POINT('Ctrl Pts',(173.055672188531,-54.4392567683325,41.676877439586));
#24187=CARTESIAN_POINT('Ctrl Pts',(173.027836194607,-54.4482298591699,41.7238446245605));
#24188=CARTESIAN_POINT('Ctrl Pts',(173.,-54.463528575122,41.7686493678573));
#24189=CARTESIAN_POINT('Ctrl Pts',(172.922663031266,-54.5437329784671,41.8973236981601));
#24190=CARTESIAN_POINT('Ctrl Pts',(172.948576579161,-54.5068140601558,41.8597169177226));
#24191=CARTESIAN_POINT('Ctrl Pts',(172.974288339751,-54.4797133174499,41.8160489814978));
#24192=CARTESIAN_POINT('Ctrl Pts',(173.,-54.463528575122,41.7686493678573));
#24193=CARTESIAN_POINT('Ctrl Pts',(172.762221454686,-54.6515169577261,42.1682945422757));
#24194=CARTESIAN_POINT('Ctrl Pts',(172.841480969791,-54.5743713519791,42.0425563958593));
#24195=CARTESIAN_POINT('Ctrl Pts',(172.920740484895,-54.5111967757298,41.9082533384352));
#24196=CARTESIAN_POINT('Ctrl Pts',(173.,-54.463528575122,41.7686493678573));
#24197=CARTESIAN_POINT('',(173.,-54.463528575122,41.7686493678573));
#24198=CARTESIAN_POINT('Ctrl Pts',(173.243546184425,-54.3281650199493,41.3553820099289));
#24199=CARTESIAN_POINT('Ctrl Pts',(173.162767797901,-54.3716994765092,41.4940379614493));
#24200=CARTESIAN_POINT('Ctrl Pts',(173.081384049463,-54.41674640089,41.6316402676231));
#24201=CARTESIAN_POINT('Ctrl Pts',(173.,-54.463528575122,41.7686493678573));
#24202=CARTESIAN_POINT('Ctrl Pts',(173.,-54.463528575122,41.7686493678573));
#24203=CARTESIAN_POINT('Ctrl Pts',(172.920740484895,-54.5111967757298,41.9082533384352));
#24204=CARTESIAN_POINT('Ctrl Pts',(172.841480969791,-54.5743713519791,42.0425563958593));
#24205=CARTESIAN_POINT('Ctrl Pts',(172.762221454686,-54.6515169577261,42.1682945422757));
#24206=CARTESIAN_POINT('Origin',(173.,-45.,45.));
#24207=CARTESIAN_POINT('',(175.,-41.1096563890154,56.3518820725231));
#24208=CARTESIAN_POINT('Origin',(175.,-45.,45.));
#24209=CARTESIAN_POINT('',(173.,-41.7580469908461,54.4599017271026));
#24210=CARTESIAN_POINT('Origin',(173.,-41.1096563890154,56.3518820725231));
#24211=CARTESIAN_POINT('Origin',(173.,-45.,45.));
#24212=CARTESIAN_POINT('Origin',(175.,0.,0.));
#24213=CARTESIAN_POINT('',(175.,-41.1096563890154,-56.3518820725231));
#24214=CARTESIAN_POINT('Origin',(175.,-45.,-45.));
#24215=CARTESIAN_POINT('',(175.,-32.,-58.));
#24216=CARTESIAN_POINT('Origin',(175.,-32.,-32.));
#24217=CARTESIAN_POINT('',(175.,32.,-58.));
#24218=CARTESIAN_POINT('',(175.,-16.,-58.));
#24219=CARTESIAN_POINT('',(175.,41.1096563890154,-56.3518820725231));
#24220=CARTESIAN_POINT('Origin',(175.,32.,-32.));
#24221=CARTESIAN_POINT('',(175.,56.3518820725231,-41.1096563890154));
#24222=CARTESIAN_POINT('Origin',(175.,45.,-45.));
#24223=CARTESIAN_POINT('',(175.,57.9807621135332,-31.));
#24224=CARTESIAN_POINT('Origin',(175.,32.,-32.));
#24225=CARTESIAN_POINT('',(175.,64.,-31.));
#24226=CARTESIAN_POINT('',(175.,26.5,-31.));
#24227=CARTESIAN_POINT('',(175.,64.,31.));
#24228=CARTESIAN_POINT('',(175.,64.,-16.5));
#24229=CARTESIAN_POINT('',(175.,57.9807621135332,31.));
#24230=CARTESIAN_POINT('',(175.,26.5,31.));
#24231=CARTESIAN_POINT('',(175.,56.3518820725231,41.1096563890154));
#24232=CARTESIAN_POINT('Origin',(175.,32.,32.));
#24233=CARTESIAN_POINT('',(175.,41.1096563890154,56.3518820725231));
#24234=CARTESIAN_POINT('Origin',(175.,45.,45.));
#24235=CARTESIAN_POINT('',(175.,32.,58.));
#24236=CARTESIAN_POINT('Origin',(175.,32.,32.));
#24237=CARTESIAN_POINT('',(175.,-32.,58.));
#24238=CARTESIAN_POINT('',(175.,16.,58.));
#24239=CARTESIAN_POINT('Origin',(175.,-32.,32.));
#24240=CARTESIAN_POINT('',(175.,-30.,40.));
#24241=CARTESIAN_POINT('',(175.,-30.,-40.));
#24242=CARTESIAN_POINT('Origin',(138.1,65.75,25.4));
#24243=CARTESIAN_POINT('',(132.55,66.,25.4));
#24244=CARTESIAN_POINT('Origin',(138.1,66.,25.4));
#24245=CARTESIAN_POINT('',(133.05,65.5,25.4));
#24246=CARTESIAN_POINT('',(132.8,65.75,25.4));
#24247=CARTESIAN_POINT('Origin',(138.1,65.5,25.4));
#24248=CARTESIAN_POINT('Origin',(175.,66.,-33.));
#24249=CARTESIAN_POINT('',(127.8,66.,31.));
#24250=CARTESIAN_POINT('',(127.8,66.,-31.));
#24251=CARTESIAN_POINT('',(127.8,66.,-16.5));
#24252=CARTESIAN_POINT('',(173.,66.,31.));
#24253=CARTESIAN_POINT('',(162.7,66.,31.));
#24254=CARTESIAN_POINT('',(173.,66.,-31.));
#24255=CARTESIAN_POINT('',(173.,66.,-16.5));
#24256=CARTESIAN_POINT('',(162.7,66.,-31.));
#24257=CARTESIAN_POINT('',(156.35,66.,-25.4));
#24258=CARTESIAN_POINT('Origin',(161.9,66.,-25.4));
#24259=CARTESIAN_POINT('',(132.55,66.,-25.4));
#24260=CARTESIAN_POINT('Origin',(138.1,66.,-25.4));
#24261=CARTESIAN_POINT('',(140.,66.,1.22464679914735E-15));
#24262=CARTESIAN_POINT('Origin',(150.,66.,0.));
#24263=CARTESIAN_POINT('',(156.35,66.,25.4));
#24264=CARTESIAN_POINT('Origin',(161.9,66.,25.4));
#24265=CARTESIAN_POINT('Origin',(138.1,66.,25.4));
#24266=CARTESIAN_POINT('',(133.05,49.,25.4));
#24267=CARTESIAN_POINT('',(133.05,66.,25.4));
#24268=CARTESIAN_POINT('Origin',(138.1,49.,25.4));
#24269=CARTESIAN_POINT('Origin',(161.9,65.75,-25.4));
#24270=CARTESIAN_POINT('',(156.85,65.5,-25.4));
#24271=CARTESIAN_POINT('',(156.6,65.75,-25.4));
#24272=CARTESIAN_POINT('Origin',(161.9,65.5,-25.4));
#24273=CARTESIAN_POINT('Origin',(161.9,66.,-25.4));
#24274=CARTESIAN_POINT('',(156.85,49.,-25.4));
#24275=CARTESIAN_POINT('',(156.85,66.,-25.4));
#24276=CARTESIAN_POINT('Origin',(161.9,49.,-25.4));
#24277=CARTESIAN_POINT('Origin',(161.9,65.75,25.4));
#24278=CARTESIAN_POINT('',(156.85,65.5,25.4));
#24279=CARTESIAN_POINT('',(156.6,65.75,25.4));
#24280=CARTESIAN_POINT('Origin',(161.9,65.5,25.4));
#24281=CARTESIAN_POINT('Origin',(161.9,66.,25.4));
#24282=CARTESIAN_POINT('',(156.85,49.,25.4));
#24283=CARTESIAN_POINT('',(156.85,66.,25.4));
#24284=CARTESIAN_POINT('Origin',(161.9,49.,25.4));
#24285=CARTESIAN_POINT('Origin',(138.1,65.75,-25.4));
#24286=CARTESIAN_POINT('',(133.05,65.5,-25.4));
#24287=CARTESIAN_POINT('',(132.8,65.75,-25.4));
#24288=CARTESIAN_POINT('Origin',(138.1,65.5,-25.4));
#24289=CARTESIAN_POINT('Origin',(138.1,66.,-25.4));
#24290=CARTESIAN_POINT('',(133.05,49.,-25.4));
#24291=CARTESIAN_POINT('',(133.05,66.,-25.4));
#24292=CARTESIAN_POINT('Origin',(138.1,49.,-25.4));
#24293=CARTESIAN_POINT('Origin',(150.,65.75,0.));
#24294=CARTESIAN_POINT('',(140.5,65.5,-1.16341445918998E-15));
#24295=CARTESIAN_POINT('',(140.25,65.75,1.19403062916867E-15));
#24296=CARTESIAN_POINT('Origin',(150.,65.5,0.));
#24297=CARTESIAN_POINT('Origin',(150.,66.,0.));
#24298=CARTESIAN_POINT('',(140.5024163973,35.9970291210556,0.000659424480330972));
#24299=CARTESIAN_POINT('',(140.5,66.,-1.16341445918998E-15));
#24300=CARTESIAN_POINT('',(140.502173012404,20.0025228153278,0.000820030757110642));
#24301=CARTESIAN_POINT('Ctrl Pts',(140.502472449209,20.002870454282,0.000933029370863217));
#24302=CARTESIAN_POINT('Ctrl Pts',(140.502079425243,20.0023872760223,-0.513648430176057));
#24303=CARTESIAN_POINT('Ctrl Pts',(140.580570085935,20.1416700372709,-1.54333997704372));
#24304=CARTESIAN_POINT('Ctrl Pts',(140.940135198509,20.7760302225561,-2.96372789758379));
#24305=CARTESIAN_POINT('Ctrl Pts',(141.613773440736,22.0590093116005,-4.60669302069982));
#24306=CARTESIAN_POINT('Ctrl Pts',(142.51650955026,24.0303305797403,-5.90697582915808));
#24307=CARTESIAN_POINT('Ctrl Pts',(143.197512601211,26.7250000406644,-6.63359194555753));
#24308=CARTESIAN_POINT('Ctrl Pts',(143.198827571655,29.2764783425835,-6.63422718178349));
#24309=CARTESIAN_POINT('Ctrl Pts',(142.61406517216,31.5865966550244,-6.01113699999118));
#24310=CARTESIAN_POINT('Ctrl Pts',(141.828024497579,33.5000354399014,-4.9254108406999));
#24311=CARTESIAN_POINT('Ctrl Pts',(141.077842938275,34.9766629596617,-3.42496442652058));
#24312=CARTESIAN_POINT('Ctrl Pts',(140.593484092959,35.8349779276441,-1.71480123653937));
#24313=CARTESIAN_POINT('Ctrl Pts',(140.502479291261,35.9969413163685,-0.513694213206118));
#24314=CARTESIAN_POINT('Ctrl Pts',(140.502956649271,35.9963648994868,0.00080685693081263));
#24315=CARTESIAN_POINT('Origin',(150.,20.,0.));
#24316=CARTESIAN_POINT('',(143.175401713146,28.,6.60869565217391));
#24317=CARTESIAN_POINT('Ctrl Pts',(143.175401713146,28.,6.60869565217391));
#24318=CARTESIAN_POINT('Ctrl Pts',(143.175401713146,27.3777956850962,6.60869565217391));
#24319=CARTESIAN_POINT('Ctrl Pts',(143.05419832612,26.1354767285296,6.48707115577184));
#24320=CARTESIAN_POINT('Ctrl Pts',(142.44802175351,23.8795076799284,5.80658697436831));
#24321=CARTESIAN_POINT('Ctrl Pts',(141.407577159842,21.6081542657929,4.31108301914421));
#24322=CARTESIAN_POINT('Ctrl Pts',(140.622943710823,20.2151487945374,2.05828551505037));
#24323=CARTESIAN_POINT('Ctrl Pts',(140.502865436407,20.0033535873405,0.515466350059816));
#24324=CARTESIAN_POINT('Ctrl Pts',(140.502472449209,20.002870454282,0.000933029370863217));
#24325=CARTESIAN_POINT('Ctrl Pts',(140.502956649271,35.9963648994868,0.00080685693081263));
#24326=CARTESIAN_POINT('Ctrl Pts',(140.503434038327,35.9957884451177,0.515341387647046));
#24327=CARTESIAN_POINT('Ctrl Pts',(140.623315085809,35.7840723365628,2.05816288432255));
#24328=CARTESIAN_POINT('Ctrl Pts',(141.409078045969,34.3900535537995,4.31115068270884));
#24329=CARTESIAN_POINT('Ctrl Pts',(142.448051488086,32.1203379370536,5.80658533410845));
#24330=CARTESIAN_POINT('Ctrl Pts',(143.054377037915,29.8642777153372,6.48707561474873));
#24331=CARTESIAN_POINT('Ctrl Pts',(143.175401713146,28.622204314904,6.60869565217392));
#24332=CARTESIAN_POINT('Ctrl Pts',(143.175401713146,28.,6.60869565217392));
#24333=CARTESIAN_POINT('Ctrl Pts',(141.738644179071,28.,6.));
#24334=CARTESIAN_POINT('Ctrl Pts',(141.738644179071,28.466653236178,6.));
#24335=CARTESIAN_POINT('Ctrl Pts',(141.592140624844,29.3982082865029,5.88958180812713));
#24336=CARTESIAN_POINT('Ctrl Pts',(140.858167590841,31.0902534527902,5.27176826386162));
#24337=CARTESIAN_POINT('Ctrl Pts',(139.600462897751,32.7925401653496,3.9140710145646));
#24338=CARTESIAN_POINT('Ctrl Pts',(138.45904623122,34.0471489107534,1.45951606005547));
#24339=CARTESIAN_POINT('Ctrl Pts',(138.453250392708,34.0518051367242,-1.13339199495755));
#24340=CARTESIAN_POINT('Ctrl Pts',(139.199494083175,33.2324972197463,-3.10950717670948));
#24341=CARTESIAN_POINT('Ctrl Pts',(140.107608602332,32.125026579926,-4.4717545790565));
#24342=CARTESIAN_POINT('Ctrl Pts',(141.059131524193,30.6899474912683,-5.45747964472883));
#24343=CARTESIAN_POINT('Ctrl Pts',(141.767001797266,28.9573587569376,-6.02317994135606));
#24344=CARTESIAN_POINT('Ctrl Pts',(141.76540999094,27.0437500304983,-6.02260321372987));
#24345=CARTESIAN_POINT('Ctrl Pts',(140.941037876631,25.0227479348052,-5.36291226594614));
#24346=CARTESIAN_POINT('Ctrl Pts',(139.848252059838,23.5442569837004,-4.18239234774062));
#24347=CARTESIAN_POINT('Ctrl Pts',(139.032795240301,22.5820226669171,-2.69075295964843));
#24348=CARTESIAN_POINT('Ctrl Pts',(138.452453581158,21.9476723726241,-0.97136281248494));
#24349=CARTESIAN_POINT('Ctrl Pts',(138.458852046436,21.9523990462047,1.45962302485803));
#24350=CARTESIAN_POINT('Ctrl Pts',(139.598646035598,23.2061156993447,3.91400958317042));
#24351=CARTESIAN_POINT('Ctrl Pts',(140.858131596355,24.9096307599463,5.27176975304492));
#24352=CARTESIAN_POINT('Ctrl Pts',(141.591924289514,26.6016075463972,5.88957775984548));
#24353=CARTESIAN_POINT('Ctrl Pts',(141.738644179071,27.533346763822,6.));
#24354=CARTESIAN_POINT('Ctrl Pts',(141.738644179071,28.,6.));
#24355=CARTESIAN_POINT('Ctrl Pts',(142.043965696508,28.,6.));
#24356=CARTESIAN_POINT('Ctrl Pts',(142.043965696508,28.489619376602,6.));
#24357=CARTESIAN_POINT('Ctrl Pts',(141.905479893413,29.4675535704741,5.87773555290971));
#24358=CARTESIAN_POINT('Ctrl Pts',(141.217720935708,31.2218964506089,5.20599667447634));
#24359=CARTESIAN_POINT('Ctrl Pts',(140.053424701285,32.9275777830355,3.7514473788431));
#24360=CARTESIAN_POINT('Ctrl Pts',(139.061090117389,34.0443918223547,1.33284727256326));
#24361=CARTESIAN_POINT('Ctrl Pts',(139.059027025196,34.0430682506412,-1.03627554436337));
#24362=CARTESIAN_POINT('Ctrl Pts',(139.702875040431,33.322365386674,-2.95193917049126));
#24363=CARTESIAN_POINT('Ctrl Pts',(140.524068736404,32.258214133341,-4.35124876313713));
#24364=CARTESIAN_POINT('Ctrl Pts',(141.404330684989,30.8114576637609,-5.40538794487833));
#24365=CARTESIAN_POINT('Ctrl Pts',(142.070230027061,29.0064483130425,-6.02585560608033));
#24366=CARTESIAN_POINT('Ctrl Pts',(142.068792362312,26.9942998217749,-6.0249220615482));
#24367=CARTESIAN_POINT('Ctrl Pts',(141.2929367632,24.8886851324338,-5.30236034708324));
#24368=CARTESIAN_POINT('Ctrl Pts',(140.285567337581,23.4147662511711,-4.04197533388614));
#24369=CARTESIAN_POINT('Ctrl Pts',(139.558150790354,22.512706151362,-2.54371757658131));
#24370=CARTESIAN_POINT('Ctrl Pts',(139.058822833885,21.957295463926,-0.888260075897155));
#24371=CARTESIAN_POINT('Ctrl Pts',(139.061067834149,21.9556534193931,1.33302010233888));
#24372=CARTESIAN_POINT('Ctrl Pts',(140.052488123096,23.0724505819996,3.75147334802102));
#24373=CARTESIAN_POINT('Ctrl Pts',(141.217701781722,24.7780427741925,5.20600221509276));
#24374=CARTESIAN_POINT('Ctrl Pts',(141.905368227135,26.5324235696485,5.87774188530814));
#24375=CARTESIAN_POINT('Ctrl Pts',(142.043965696508,27.510380623398,6.));
#24376=CARTESIAN_POINT('Ctrl Pts',(142.043965696508,28.,6.));
#24377=CARTESIAN_POINT('Ctrl Pts',(142.57788822158,28.,6.12463030305979));
#24378=CARTESIAN_POINT('Ctrl Pts',(142.57788822158,28.5395615790993,6.12463030305979));
#24379=CARTESIAN_POINT('Ctrl Pts',(142.453723397324,29.6171845933956,5.99156227883951));
#24380=CARTESIAN_POINT('Ctrl Pts',(141.846341502135,31.5440219059675,5.268772011394));
#24381=CARTESIAN_POINT('Ctrl Pts',(140.844323830014,33.4026543544232,3.71115220069704));
#24382=CARTESIAN_POINT('Ctrl Pts',(140.100655327228,34.5544656664828,1.26154906292248));
#24383=CARTESIAN_POINT('Ctrl Pts',(140.103937101032,34.5500472995073,-0.981414646809834));
#24384=CARTESIAN_POINT('Ctrl Pts',(140.578675206434,33.8115119944716,-2.89529601543811));
#24385=CARTESIAN_POINT('Ctrl Pts',(141.251976097117,32.6708724945202,-4.35505081975209));
#24386=CARTESIAN_POINT('Ctrl Pts',(142.0093534077,31.0940053129146,-5.48116085900691));
#24387=CARTESIAN_POINT('Ctrl Pts',(142.601771765176,29.1092669955987,-6.15227033925031));
#24388=CARTESIAN_POINT('Ctrl Pts',(142.600547825936,26.8912001711519,-6.15101629252184));
#24389=CARTESIAN_POINT('Ctrl Pts',(141.909317212412,24.5751011285043,-5.37058697183273));
#24390=CARTESIAN_POINT('Ctrl Pts',(141.049251669911,22.9739732545708,-4.02397204951632));
#24391=CARTESIAN_POINT('Ctrl Pts',(140.47000213459,22.0173629223548,-2.48551241031029));
#24392=CARTESIAN_POINT('Ctrl Pts',(140.104591253159,21.450847766609,-0.841472379185922));
#24393=CARTESIAN_POINT('Ctrl Pts',(140.100297492759,21.4446966445209,1.26149033180786));
#24394=CARTESIAN_POINT('Ctrl Pts',(140.844653274062,22.5980254068523,3.7109471930761));
#24395=CARTESIAN_POINT('Ctrl Pts',(141.846258982871,24.4557692411548,5.2687424407902));
#24396=CARTESIAN_POINT('Ctrl Pts',(142.453763523801,26.3828695847505,5.99154161878406));
#24397=CARTESIAN_POINT('Ctrl Pts',(142.57788822158,27.4604384209008,6.12463030305979));
#24398=CARTESIAN_POINT('Ctrl Pts',(142.57788822158,28.,6.12463030305979));
#24399=CARTESIAN_POINT('Ctrl Pts',(143.016103530135,28.,6.44419328073923));
#24400=CARTESIAN_POINT('Ctrl Pts',(143.016103530135,28.5974178246517,6.44419328073923));
#24401=CARTESIAN_POINT('Ctrl Pts',(142.896149230359,29.7901391902406,6.31763407548422));
#24402=CARTESIAN_POINT('Ctrl Pts',(142.301895316234,31.9474466700465,5.61797095740714));
#24403=CARTESIAN_POINT('Ctrl Pts',(141.303027832022,34.0939356482408,4.09471435137365));
#24404=CARTESIAN_POINT('Ctrl Pts',(140.467893969615,35.6111302989085,1.4824078247523));
#24405=CARTESIAN_POINT('Ctrl Pts',(140.466527313903,35.6142168793452,-1.15183663734545));
#24406=CARTESIAN_POINT('Ctrl Pts',(141.007809366,34.627410681629,-3.23372564469958));
#24407=CARTESIAN_POINT('Ctrl Pts',(141.70681890823,33.2513146547413,-4.72180677695984));
#24408=CARTESIAN_POINT('Ctrl Pts',(142.46286099909,31.4387556515361,-5.82640140894008));
#24409=CARTESIAN_POINT('Ctrl Pts',(143.038905695447,29.226321106751,-6.47066418005133));
#24410=CARTESIAN_POINT('Ctrl Pts',(143.037683909907,26.7748498264222,-6.46980943905863));
#24411=CARTESIAN_POINT('Ctrl Pts',(142.366284600791,24.1937858935098,-5.7192270911062));
#24412=CARTESIAN_POINT('Ctrl Pts',(141.502681958482,22.3334174658961,-4.39763660762648));
#24413=CARTESIAN_POINT('Ctrl Pts',(140.885992207105,21.1479815909271,-2.79104896834084));
#24414=CARTESIAN_POINT('Ctrl Pts',(140.466409892293,20.3855543526367,-0.987293662979608));
#24415=CARTESIAN_POINT('Ctrl Pts',(140.4678361008,20.3881444401133,1.48246616303375));
#24416=CARTESIAN_POINT('Ctrl Pts',(141.302327362314,21.9049988827169,4.09461479833817));
#24417=CARTESIAN_POINT('Ctrl Pts',(142.301871353512,24.0523749164083,5.61796148916296));
#24418=CARTESIAN_POINT('Ctrl Pts',(142.896065782025,26.2097035136665,6.3176258699495));
#24419=CARTESIAN_POINT('Ctrl Pts',(143.016103530135,27.4025821753484,6.44419328073922));
#24420=CARTESIAN_POINT('Ctrl Pts',(143.016103530135,28.,6.44419328073922));
#24421=CARTESIAN_POINT('Ctrl Pts',(143.175401713146,28.,6.60869565217392));
#24422=CARTESIAN_POINT('Ctrl Pts',(143.175401713146,28.622204314904,6.60869565217392));
#24423=CARTESIAN_POINT('Ctrl Pts',(143.054377037915,29.8642777153372,6.48707561474873));
#24424=CARTESIAN_POINT('Ctrl Pts',(142.448051488086,32.1203379370536,5.80658533410845));
#24425=CARTESIAN_POINT('Ctrl Pts',(141.409078045969,34.3900535537995,4.31115068270884));
#24426=CARTESIAN_POINT('Ctrl Pts',(140.46616862579,36.0628652143378,1.60758290672775));
#24427=CARTESIAN_POINT('Ctrl Pts',(140.461380759193,36.0690735156323,-1.24837379154744));
#24428=CARTESIAN_POINT('Ctrl Pts',(141.077842938275,34.9766629596617,-3.42496442652058));
#24429=CARTESIAN_POINT('Ctrl Pts',(141.828024497579,33.5000354399014,-4.9254108406999));
#24430=CARTESIAN_POINT('Ctrl Pts',(142.61406517216,31.5865966550244,-6.01113699999118));
#24431=CARTESIAN_POINT('Ctrl Pts',(143.198827571655,29.2764783425835,-6.63422718178349));
#24432=CARTESIAN_POINT('Ctrl Pts',(143.197512601211,26.7250000406644,-6.63359194555753));
#24433=CARTESIAN_POINT('Ctrl Pts',(142.51650955026,24.0303305797403,-5.90697582915808));
#24434=CARTESIAN_POINT('Ctrl Pts',(141.613773440736,22.0590093116005,-4.60669302069982));
#24435=CARTESIAN_POINT('Ctrl Pts',(140.940135198509,20.7760302225561,-2.96372789758379));
#24436=CARTESIAN_POINT('Ctrl Pts',(140.460722523566,19.9302298301654,-1.06990686592545));
#24437=CARTESIAN_POINT('Ctrl Pts',(140.466008212273,19.9365320616062,1.60770072303204));
#24438=CARTESIAN_POINT('Ctrl Pts',(141.407577159842,21.6081542657929,4.31108301914421));
#24439=CARTESIAN_POINT('Ctrl Pts',(142.44802175351,23.8795076799284,5.80658697436831));
#24440=CARTESIAN_POINT('Ctrl Pts',(143.05419832612,26.1354767285296,6.48707115577184));
#24441=CARTESIAN_POINT('Ctrl Pts',(143.175401713146,27.3777956850962,6.60869565217391));
#24442=CARTESIAN_POINT('Ctrl Pts',(143.175401713146,28.,6.60869565217391));
#24443=CARTESIAN_POINT('',(141.738644179071,28.,6.));
#24444=CARTESIAN_POINT('Origin',(141.738644179071,28.,8.));
#24445=CARTESIAN_POINT('Ctrl Pts',(141.738644179071,28.,6.));
#24446=CARTESIAN_POINT('Ctrl Pts',(141.738644179071,28.466653236178,6.));
#24447=CARTESIAN_POINT('Ctrl Pts',(141.592140624844,29.3982082865029,5.88958180812713));
#24448=CARTESIAN_POINT('Ctrl Pts',(140.858167590841,31.0902534527902,5.27176826386162));
#24449=CARTESIAN_POINT('Ctrl Pts',(139.600462897751,32.7925401653496,3.9140710145646));
#24450=CARTESIAN_POINT('Ctrl Pts',(138.45904623122,34.0471489107534,1.45951606005547));
#24451=CARTESIAN_POINT('Ctrl Pts',(138.453250392708,34.0518051367242,-1.13339199495755));
#24452=CARTESIAN_POINT('Ctrl Pts',(139.199494083175,33.2324972197463,-3.10950717670948));
#24453=CARTESIAN_POINT('Ctrl Pts',(140.107608602332,32.125026579926,-4.4717545790565));
#24454=CARTESIAN_POINT('Ctrl Pts',(141.059131524193,30.6899474912683,-5.45747964472883));
#24455=CARTESIAN_POINT('Ctrl Pts',(141.767001797266,28.9573587569376,-6.02317994135606));
#24456=CARTESIAN_POINT('Ctrl Pts',(141.76540999094,27.0437500304983,-6.02260321372987));
#24457=CARTESIAN_POINT('Ctrl Pts',(140.941037876631,25.0227479348052,-5.36291226594614));
#24458=CARTESIAN_POINT('Ctrl Pts',(139.848252059838,23.5442569837004,-4.18239234774062));
#24459=CARTESIAN_POINT('Ctrl Pts',(139.032795240301,22.5820226669171,-2.69075295964843));
#24460=CARTESIAN_POINT('Ctrl Pts',(138.452453581158,21.9476723726241,-0.97136281248494));
#24461=CARTESIAN_POINT('Ctrl Pts',(138.458852046436,21.9523990462047,1.45962302485803));
#24462=CARTESIAN_POINT('Ctrl Pts',(139.598646035598,23.2061156993447,3.91400958317042));
#24463=CARTESIAN_POINT('Ctrl Pts',(140.858131596355,24.9096307599463,5.27176975304492));
#24464=CARTESIAN_POINT('Ctrl Pts',(141.591924289514,26.6016075463972,5.88957775984548));
#24465=CARTESIAN_POINT('Ctrl Pts',(141.738644179071,27.533346763822,6.));
#24466=CARTESIAN_POINT('Ctrl Pts',(141.738644179071,28.,6.));
#24467=CARTESIAN_POINT('Origin',(129.8,28.,0.));
#24468=CARTESIAN_POINT('',(129.8,28.,6.));
#24469=CARTESIAN_POINT('Origin',(129.8,28.,0.));
#24470=CARTESIAN_POINT('',(129.8,28.,6.));
#24471=CARTESIAN_POINT('Origin',(127.8,26.5,-31.));
#24472=CARTESIAN_POINT('',(125.8,64.,-31.));
#24473=CARTESIAN_POINT('',(127.8,64.,-33.));
#24474=CARTESIAN_POINT('Origin',(127.8,64.,-31.));
#24475=CARTESIAN_POINT('',(127.8,59.9821371592664,-33.));
#24476=CARTESIAN_POINT('',(127.8,26.5,-33.));
#24477=CARTESIAN_POINT('',(125.8,57.9807621135332,-31.));
#24478=CARTESIAN_POINT('Ctrl Pts',(125.8,57.9807621135332,-31.));
#24479=CARTESIAN_POINT('Ctrl Pts',(125.8,57.982778257817,-31.0019400357417));
#24480=CARTESIAN_POINT('Ctrl Pts',(125.800002822804,57.9847942901491,-31.0038801895753));
#24481=CARTESIAN_POINT('Ctrl Pts',(125.80098220099,58.3344433583997,-31.3404084852548));
#24482=CARTESIAN_POINT('Ctrl Pts',(125.885795069427,58.6701680223804,-31.6705622861173));
#24483=CARTESIAN_POINT('Ctrl Pts',(126.152636007272,59.1545342172526,-32.1543180026666));
#24484=CARTESIAN_POINT('Ctrl Pts',(126.29212533093,59.3337989076212,-32.3354122100755));
#24485=CARTESIAN_POINT('Ctrl Pts',(126.64930385163,59.6459583395507,-32.6532332234622));
#24486=CARTESIAN_POINT('Ctrl Pts',(126.853946614142,59.7672434939641,-32.7780158331185));
#24487=CARTESIAN_POINT('Ctrl Pts',(127.208967246466,59.9010691778161,-32.9160577581802));
#24488=CARTESIAN_POINT('Ctrl Pts',(127.351252183116,59.9385021348617,-32.9548041970754));
#24489=CARTESIAN_POINT('Ctrl Pts',(127.59877150075,59.9747656314413,-32.9923574576679));
#24490=CARTESIAN_POINT('Ctrl Pts',(127.699058685214,59.9821371592665,-33.));
#24491=CARTESIAN_POINT('Ctrl Pts',(127.8,59.9821371592665,-33.));
#24492=CARTESIAN_POINT('',(125.8,26.5,-31.));
#24493=CARTESIAN_POINT('Origin',(127.8,64.,31.));
#24494=CARTESIAN_POINT('',(127.8,64.,33.));
#24495=CARTESIAN_POINT('Origin',(127.8,64.,31.));
#24496=CARTESIAN_POINT('',(125.8,64.,31.));
#24497=CARTESIAN_POINT('Origin',(127.8,64.,31.));
#24498=CARTESIAN_POINT('Origin',(127.8,64.,31.));
#24499=CARTESIAN_POINT('Origin',(127.8,64.,-16.5));
#24500=CARTESIAN_POINT('Origin',(127.8,64.,-31.));
#24501=CARTESIAN_POINT('',(125.8,64.,-16.5));
#24502=CARTESIAN_POINT('Origin',(127.8,26.5,31.));
#24503=CARTESIAN_POINT('',(125.8,57.9807621135332,31.));
#24504=CARTESIAN_POINT('',(127.8,59.9821371592664,33.));
#24505=CARTESIAN_POINT('Ctrl Pts',(127.8,59.9821371592664,33.));
#24506=CARTESIAN_POINT('Ctrl Pts',(127.699058685214,59.9821371592664,33.));
#24507=CARTESIAN_POINT('Ctrl Pts',(127.59877150075,59.9747656314413,32.9923574576679));
#24508=CARTESIAN_POINT('Ctrl Pts',(127.351252183116,59.9385021348617,32.9548041970754));
#24509=CARTESIAN_POINT('Ctrl Pts',(127.208967246466,59.9010691778161,32.9160577581802));
#24510=CARTESIAN_POINT('Ctrl Pts',(126.853946614143,59.7672434939644,32.7780158331189));
#24511=CARTESIAN_POINT('Ctrl Pts',(126.649303851631,59.6459583395513,32.6532332234628));
#24512=CARTESIAN_POINT('Ctrl Pts',(126.29212533093,59.3337989076212,32.3354122100755));
#24513=CARTESIAN_POINT('Ctrl Pts',(126.152636007272,59.1545342172527,32.1543180026667));
#24514=CARTESIAN_POINT('Ctrl Pts',(125.885795045952,58.6701679797686,31.6705622435593));
#24515=CARTESIAN_POINT('Ctrl Pts',(125.800982200837,58.3344433038848,31.3404084324536));
#24516=CARTESIAN_POINT('Ctrl Pts',(125.800002822804,57.9847942902325,31.0038801896633));
#24517=CARTESIAN_POINT('Ctrl Pts',(125.8,57.9827782577327,31.0019400356606));
#24518=CARTESIAN_POINT('Ctrl Pts',(125.8,57.9807621135332,31.));
#24519=CARTESIAN_POINT('',(127.8,26.5,33.));
#24520=CARTESIAN_POINT('',(125.8,26.5,31.));
#24521=CARTESIAN_POINT('Origin',(162.7,64.,31.));
#24522=CARTESIAN_POINT('',(173.,64.,33.));
#24523=CARTESIAN_POINT('Origin',(173.,64.,31.));
#24524=CARTESIAN_POINT('',(162.7,64.,33.));
#24525=CARTESIAN_POINT('Origin',(127.8,64.,-31.));
#24526=CARTESIAN_POINT('Origin',(127.8,64.,-31.));
#24527=CARTESIAN_POINT('Origin',(173.,26.5,31.));
#24528=CARTESIAN_POINT('Origin',(173.,64.,31.));
#24529=CARTESIAN_POINT('',(173.,59.9821371592664,33.));
#24530=CARTESIAN_POINT('',(173.,26.5,33.));
#24531=CARTESIAN_POINT('Ctrl Pts',(175.,57.9807621135332,31.));
#24532=CARTESIAN_POINT('Ctrl Pts',(175.,57.9827782576468,31.0019400355779));
#24533=CARTESIAN_POINT('Ctrl Pts',(174.999997177196,57.984794290312,31.0038801897477));
#24534=CARTESIAN_POINT('Ctrl Pts',(174.999017799316,58.3344432492304,31.3404083795179));
#24535=CARTESIAN_POINT('Ctrl Pts',(174.914204977582,58.6701679370494,31.6705622008938));
#24536=CARTESIAN_POINT('Ctrl Pts',(174.647363992729,59.1545342172525,32.1543180026665));
#24537=CARTESIAN_POINT('Ctrl Pts',(174.50787466907,59.3337989076211,32.3354122100754));
#24538=CARTESIAN_POINT('Ctrl Pts',(174.150696148369,59.6459583395515,32.6532332234631));
#24539=CARTESIAN_POINT('Ctrl Pts',(173.946053385857,59.7672434939645,32.778015833119));
#24540=CARTESIAN_POINT('Ctrl Pts',(173.591032753534,59.9010691778161,32.9160577581802));
#24541=CARTESIAN_POINT('Ctrl Pts',(173.448747816884,59.9385021348617,32.9548041970754));
#24542=CARTESIAN_POINT('Ctrl Pts',(173.20122849925,59.9747656314413,32.9923574576679));
#24543=CARTESIAN_POINT('Ctrl Pts',(173.100941314786,59.9821371592665,33.));
#24544=CARTESIAN_POINT('Ctrl Pts',(173.,59.9821371592665,33.));
#24545=CARTESIAN_POINT('Origin',(173.,64.,31.));
#24546=CARTESIAN_POINT('Origin',(173.,64.,31.));
#24547=CARTESIAN_POINT('Origin',(150.4,53.,-33.));
#24548=CARTESIAN_POINT('',(173.,64.,-33.));
#24549=CARTESIAN_POINT('',(162.7,64.,-33.));
#24550=CARTESIAN_POINT('',(173.,59.9821371592664,-33.));
#24551=CARTESIAN_POINT('',(173.,26.5,-33.));
#24552=CARTESIAN_POINT('',(125.8,59.9821371592664,-33.));
#24553=CARTESIAN_POINT('Origin',(162.7,64.,-31.));
#24554=CARTESIAN_POINT('Origin',(173.,64.,-31.));
#24555=CARTESIAN_POINT('Origin',(173.,64.,-16.5));
#24556=CARTESIAN_POINT('Origin',(173.,64.,-31.));
#24557=CARTESIAN_POINT('Origin',(127.8,-78.,40.));
#24558=CARTESIAN_POINT('Origin',(127.8,-78.,40.));
#24559=CARTESIAN_POINT('Origin',(127.8,-78.,-40.));
#24560=CARTESIAN_POINT('',(127.8,-78.,-42.));
#24561=CARTESIAN_POINT('Origin',(127.8,-78.,-40.));
#24562=CARTESIAN_POINT('Origin',(127.8,-78.,-40.));
#24563=CARTESIAN_POINT('Origin',(127.8,-30.,-40.));
#24564=CARTESIAN_POINT('',(125.8,-56.738633753706,-40.));
#24565=CARTESIAN_POINT('',(127.8,-58.153393661244,-42.));
#24566=CARTESIAN_POINT('Ctrl Pts',(127.8,-58.153393661244,-42.));
#24567=CARTESIAN_POINT('Ctrl Pts',(127.584791560318,-58.153393661244,-42.));
#24568=CARTESIAN_POINT('Ctrl Pts',(127.373410614215,-58.1295267522009,-41.9652805015393));
#24569=CARTESIAN_POINT('Ctrl Pts',(126.961480055368,-58.035764278849,-41.8294081195903));
#24570=CARTESIAN_POINT('Ctrl Pts',(126.768602924821,-57.9646256037392,-41.7265003535616));
#24571=CARTESIAN_POINT('Ctrl Pts',(126.401821931931,-57.7731997224245,-41.4513099318296));
#24572=CARTESIAN_POINT('Ctrl Pts',(126.239997043298,-57.6483119815763,-41.2726961269252));
#24573=CARTESIAN_POINT('Ctrl Pts',(126.009053039754,-57.3937106848192,-40.9118549730253));
#24574=CARTESIAN_POINT('Ctrl Pts',(125.930061060879,-57.2675944513766,-40.7342874762574));
#24575=CARTESIAN_POINT('Ctrl Pts',(125.826244922202,-57.0088681883845,-40.3729721347848));
#24576=CARTESIAN_POINT('Ctrl Pts',(125.800535718264,-56.8761189478115,-40.1889868307275));
#24577=CARTESIAN_POINT('Ctrl Pts',(125.800002761797,-56.7414261694738,-40.0038379708363));
#24578=CARTESIAN_POINT('Ctrl Pts',(125.8,-56.7400300001545,-40.0019189571955));
#24579=CARTESIAN_POINT('Ctrl Pts',(125.8,-56.738633753706,-40.));
#24580=CARTESIAN_POINT('',(127.8,-30.,-42.));
#24581=CARTESIAN_POINT('',(125.8,-30.,-40.));
#24582=CARTESIAN_POINT('Origin',(138.1,-78.,-40.));
#24583=CARTESIAN_POINT('',(173.,-78.,-42.));
#24584=CARTESIAN_POINT('',(138.1,-78.,-42.));
#24585=CARTESIAN_POINT('Origin',(173.,-78.,-40.));
#24586=CARTESIAN_POINT('',(138.1,-80.,-40.));
#24587=CARTESIAN_POINT('Origin',(173.,-78.,-40.));
#24588=CARTESIAN_POINT('Origin',(173.,-78.,-40.));
#24589=CARTESIAN_POINT('Origin',(173.,-78.,40.));
#24590=CARTESIAN_POINT('Origin',(173.,-78.,40.));
#24591=CARTESIAN_POINT('Origin',(127.8,-30.,40.));
#24592=CARTESIAN_POINT('',(127.8,-58.153393661244,42.));
#24593=CARTESIAN_POINT('',(125.8,-56.738633753706,40.));
#24594=CARTESIAN_POINT('Ctrl Pts',(125.8,-56.738633753706,40.));
#24595=CARTESIAN_POINT('Ctrl Pts',(125.8,-56.7400300001106,40.0019189571353));
#24596=CARTESIAN_POINT('Ctrl Pts',(125.800002761797,-56.7414261695115,40.0038379709001));
#24597=CARTESIAN_POINT('Ctrl Pts',(125.800535718258,-56.8761189462298,40.1889868282788));
#24598=CARTESIAN_POINT('Ctrl Pts',(125.826244922082,-57.008868188085,40.3729721343667));
#24599=CARTESIAN_POINT('Ctrl Pts',(125.930061060879,-57.2675944513765,40.7342874762574));
#24600=CARTESIAN_POINT('Ctrl Pts',(126.009053039754,-57.3937106848191,40.9118549730253));
#24601=CARTESIAN_POINT('Ctrl Pts',(126.239997043298,-57.6483119815763,41.2726961269252));
#24602=CARTESIAN_POINT('Ctrl Pts',(126.401821931931,-57.7731997224244,41.4513099318296));
#24603=CARTESIAN_POINT('Ctrl Pts',(126.768602924821,-57.9646256037392,41.7265003535616));
#24604=CARTESIAN_POINT('Ctrl Pts',(126.961480055368,-58.035764278849,41.8294081195903));
#24605=CARTESIAN_POINT('Ctrl Pts',(127.373410614215,-58.1295267522009,41.9652805015393));
#24606=CARTESIAN_POINT('Ctrl Pts',(127.584791560318,-58.153393661244,42.));
#24607=CARTESIAN_POINT('Ctrl Pts',(127.8,-58.153393661244,42.));
#24608=CARTESIAN_POINT('',(125.8,-30.,40.));
#24609=CARTESIAN_POINT('',(127.8,-30.,42.));
#24610=CARTESIAN_POINT('Origin',(173.,-30.,-40.));
#24611=CARTESIAN_POINT('',(173.,-30.,-42.));
#24612=CARTESIAN_POINT('Origin',(150.4,-60.,-42.));
#24613=CARTESIAN_POINT('',(125.8,-58.153393661244,-42.));
#24614=CARTESIAN_POINT('Origin',(125.8,-80.,-42.));
#24615=CARTESIAN_POINT('Origin',(125.8,0.,0.));
#24616=CARTESIAN_POINT('',(125.8,32.,-58.));
#24617=CARTESIAN_POINT('Origin',(125.8,32.,-32.));
#24618=CARTESIAN_POINT('',(125.8,-32.,-58.));
#24619=CARTESIAN_POINT('',(125.8,-16.,-58.));
#24620=CARTESIAN_POINT('Origin',(125.8,-32.,-32.));
#24621=CARTESIAN_POINT('',(125.8,-32.,58.));
#24622=CARTESIAN_POINT('Origin',(125.8,-32.,32.));
#24623=CARTESIAN_POINT('',(125.8,32.,58.));
#24624=CARTESIAN_POINT('',(125.8,16.,58.));
#24625=CARTESIAN_POINT('Origin',(125.8,32.,32.));
#24626=CARTESIAN_POINT('',(125.8,-5.51703383015883E-15,45.05));
#24627=CARTESIAN_POINT('Origin',(125.8,0.,0.));
#24628=CARTESIAN_POINT('',(125.8,-45.,-38.5));
#24629=CARTESIAN_POINT('Origin',(125.8,-45.,-45.));
#24630=CARTESIAN_POINT('',(125.8,45.,51.5));
#24631=CARTESIAN_POINT('Origin',(125.8,45.,45.));
#24632=CARTESIAN_POINT('',(125.8,-45.,51.5));
#24633=CARTESIAN_POINT('Origin',(125.8,-45.,45.));
#24634=CARTESIAN_POINT('',(125.8,45.,-38.5));
#24635=CARTESIAN_POINT('Origin',(125.8,45.,-45.));
#24636=CARTESIAN_POINT('Origin',(127.8,0.,0.));
#24637=CARTESIAN_POINT('',(127.8,-5.27210447032936E-15,43.05));
#24638=CARTESIAN_POINT('Origin',(127.8,-5.51703383015883E-15,45.05));
#24639=CARTESIAN_POINT('',(127.8,-43.05,-5.27210447032936E-15));
#24640=CARTESIAN_POINT('Origin',(127.8,0.,0.));
#24641=CARTESIAN_POINT('Origin',(127.8,0.,0.));
#24642=CARTESIAN_POINT('Origin',(127.75,0.,0.));
#24643=CARTESIAN_POINT('',(129.8,-43.05,-5.27210447032936E-15));
#24644=CARTESIAN_POINT('',(127.75,-43.05,-5.27210447032936E-15));
#24645=CARTESIAN_POINT('Origin',(129.8,0.,0.));
#24646=CARTESIAN_POINT('Origin',(127.8,-32.,-32.));
#24647=CARTESIAN_POINT('',(127.8,-32.,-60.));
#24648=CARTESIAN_POINT('Origin',(127.8,-32.,-58.));
#24649=CARTESIAN_POINT('Origin',(127.8,-32.,-32.));
#24650=CARTESIAN_POINT('Origin',(127.8,-16.,-58.));
#24651=CARTESIAN_POINT('',(127.8,32.,-60.));
#24652=CARTESIAN_POINT('Origin',(127.8,32.,-58.));
#24653=CARTESIAN_POINT('',(127.8,-16.,-60.));
#24654=CARTESIAN_POINT('Origin',(127.8,32.,-32.));
#24655=CARTESIAN_POINT('Origin',(127.8,32.,-32.));
#24656=CARTESIAN_POINT('Ctrl Pts',(131.,-20.,3.7470027081099E-15));
#24657=CARTESIAN_POINT('Ctrl Pts',(131.,-20.,0.861580403347816));
#24658=CARTESIAN_POINT('Ctrl Pts',(131.125764439308,-20.3550945008679,2.58493895098728));
#24659=CARTESIAN_POINT('Ctrl Pts',(131.558266830217,-21.7317216595771,4.69819302523181));
#24660=CARTESIAN_POINT('Ctrl Pts',(132.042509047825,-23.6963135961602,6.25318651247373));
#24661=CARTESIAN_POINT('Ctrl Pts',(132.368536443054,-25.8957266799623,7.08391599385498));
#24662=CARTESIAN_POINT('Ctrl Pts',(132.458664359226,-28.0044871996747,7.29993025650352));
#24663=CARTESIAN_POINT('Ctrl Pts',(132.380954794124,-29.8028754268023,7.11460122145983));
#24664=CARTESIAN_POINT('Ctrl Pts',(132.099300832929,-32.0502219061449,6.39759784836191));
#24665=CARTESIAN_POINT('Ctrl Pts',(131.659463837386,-33.8924146208701,5.09135905413439));
#24666=CARTESIAN_POINT('Ctrl Pts',(131.220675109436,-35.3580600016946,3.08054699453707));
#24667=CARTESIAN_POINT('Ctrl Pts',(130.959270175006,-36.1165905974382,0.896561407374775));
#24668=CARTESIAN_POINT('Ctrl Pts',(131.024509745219,-35.9339672140204,-1.76828950301325));
#24669=CARTESIAN_POINT('Ctrl Pts',(131.400892644271,-34.7994666629145,-4.05880603285176));
#24670=CARTESIAN_POINT('Ctrl Pts',(131.884794428522,-33.0159602268334,-5.7979751587154));
#24671=CARTESIAN_POINT('Ctrl Pts',(132.311702697533,-30.7087191160324,-6.95369978335721));
#24672=CARTESIAN_POINT('Ctrl Pts',(132.432701479047,-28.899900328133,-7.23809523809524));
#24673=CARTESIAN_POINT('Ctrl Pts',(132.432701479047,-28.,-7.23809523809524));
#24674=CARTESIAN_POINT('Ctrl Pts',(130.797619582017,-19.9116739443255,3.77151811328093E-15));
#24675=CARTESIAN_POINT('Ctrl Pts',(130.797619582017,-19.9116739443255,0.871444118239409));
#24676=CARTESIAN_POINT('Ctrl Pts',(130.904854620317,-20.2779548422433,2.61565600775496));
#24677=CARTESIAN_POINT('Ctrl Pts',(131.281531328409,-21.708188149755,4.72991862921347));
#24678=CARTESIAN_POINT('Ctrl Pts',(131.719414102451,-23.7218974853282,6.22503570820278));
#24679=CARTESIAN_POINT('Ctrl Pts',(132.028453321927,-25.9193631660258,6.98506280192702));
#24680=CARTESIAN_POINT('Ctrl Pts',(132.11587023659,-28.0042135305114,7.17959883876305));
#24681=CARTESIAN_POINT('Ctrl Pts',(132.040586744391,-29.7828553823862,7.0126779561723));
#24682=CARTESIAN_POINT('Ctrl Pts',(131.772280317266,-32.0212924370845,6.35840215413888));
#24683=CARTESIAN_POINT('Ctrl Pts',(131.371726605384,-33.9040625167872,5.11517750428116));
#24684=CARTESIAN_POINT('Ctrl Pts',(130.986964315205,-35.4241200681426,3.11366602926504));
#24685=CARTESIAN_POINT('Ctrl Pts',(130.762802930714,-36.2087539292741,0.907657337282378));
#24686=CARTESIAN_POINT('Ctrl Pts',(130.818337477733,-36.0207770197034,-1.78973624622093));
#24687=CARTESIAN_POINT('Ctrl Pts',(131.143137577146,-34.8435410607424,-4.09621049334934));
#24688=CARTESIAN_POINT('Ctrl Pts',(131.574530320972,-33.0022728031349,-5.79592783717056));
#24689=CARTESIAN_POINT('Ctrl Pts',(131.972813117268,-30.6784004498514,-6.86958311925421));
#24690=CARTESIAN_POINT('Ctrl Pts',(132.090706623172,-28.8898366829338,-7.12404769267738));
#24691=CARTESIAN_POINT('Ctrl Pts',(132.090706623172,-28.,-7.12404769267738));
#24692=CARTESIAN_POINT('Ctrl Pts',(130.422671463836,-19.6673355191975,3.85644558968536E-15));
#24693=CARTESIAN_POINT('Ctrl Pts',(130.422671463836,-19.6673355191975,0.89875912168986));
#24694=CARTESIAN_POINT('Ctrl Pts',(130.492531236214,-20.0479409376805,2.70000482740569));
#24695=CARTESIAN_POINT('Ctrl Pts',(130.746197220807,-21.5683467492021,4.86642730881123));
#24696=CARTESIAN_POINT('Ctrl Pts',(131.058780753502,-23.693411959482,6.31024557861326));
#24697=CARTESIAN_POINT('Ctrl Pts',(131.295887389147,-25.9273584681298,6.97089801517722));
#24698=CARTESIAN_POINT('Ctrl Pts',(131.365236878282,-28.003852058009,7.1324715976875));
#24699=CARTESIAN_POINT('Ctrl Pts',(131.30562358689,-29.7764177597774,6.99370296495644));
#24700=CARTESIAN_POINT('Ctrl Pts',(131.098323896218,-32.0392879611942,6.42935129116271));
#24701=CARTESIAN_POINT('Ctrl Pts',(130.809093968724,-34.0199081007393,5.24984625467384));
#24702=CARTESIAN_POINT('Ctrl Pts',(130.547361569822,-35.6366669116509,3.21270790048802));
#24703=CARTESIAN_POINT('Ctrl Pts',(130.400136757993,-36.4582322819073,0.935616039961515));
#24704=CARTESIAN_POINT('Ctrl Pts',(130.436222328538,-36.2637318150002,-1.84562949065027));
#24705=CARTESIAN_POINT('Ctrl Pts',(130.651675521466,-35.0205192781293,-4.22407147338777));
#24706=CARTESIAN_POINT('Ctrl Pts',(130.95294600974,-33.063483218923,-5.910694148768));
#24707=CARTESIAN_POINT('Ctrl Pts',(131.251356220669,-30.6692066978724,-6.87860346375511));
#24708=CARTESIAN_POINT('Ctrl Pts',(131.345673075562,-28.886528158348,-7.0862020745294));
#24709=CARTESIAN_POINT('Ctrl Pts',(131.345673075562,-28.,-7.0862020745294));
#24710=CARTESIAN_POINT('Ctrl Pts',(129.940396279447,-19.0495948139048,4.114252178675E-15));
#24711=CARTESIAN_POINT('Ctrl Pts',(129.940396279447,-19.0495948139048,0.967803292323193));
#24712=CARTESIAN_POINT('Ctrl Pts',(129.957030040264,-19.4304059125673,2.91217238551086));
#24713=CARTESIAN_POINT('Ctrl Pts',(130.02019438173,-21.0455248943075,5.3214716636252));
#24714=CARTESIAN_POINT('Ctrl Pts',(130.103911387302,-23.3810988218184,6.91455756751675));
#24715=CARTESIAN_POINT('Ctrl Pts',(130.172870889547,-25.8015110985969,7.58914966738149));
#24716=CARTESIAN_POINT('Ctrl Pts',(130.193826022536,-28.0039640203118,7.74532468216998));
#24717=CARTESIAN_POINT('Ctrl Pts',(130.175839613167,-29.8846980785751,7.61087423627512));
#24718=CARTESIAN_POINT('Ctrl Pts',(130.115043627593,-32.3241311937622,7.04038481196473));
#24719=CARTESIAN_POINT('Ctrl Pts',(130.036593186443,-34.5048871302672,5.74708243637949));
#24720=CARTESIAN_POINT('Ctrl Pts',(129.970485002834,-36.2397280762142,3.48005578751867));
#24721=CARTESIAN_POINT('Ctrl Pts',(129.934969533044,-37.0771971145615,1.00058657790848));
#24722=CARTESIAN_POINT('Ctrl Pts',(129.943526066177,-36.8840852946024,-1.97963074093526));
#24723=CARTESIAN_POINT('Ctrl Pts',(129.996191137842,-35.5908028312178,-4.60187443924087));
#24724=CARTESIAN_POINT('Ctrl Pts',(130.07473110145,-33.4523790881034,-6.48205257840886));
#24725=CARTESIAN_POINT('Ctrl Pts',(130.159228709516,-30.8349941080606,-7.50348217456204));
#24726=CARTESIAN_POINT('Ctrl Pts',(130.187841976599,-28.9404498479197,-7.70051204451168));
#24727=CARTESIAN_POINT('Ctrl Pts',(130.187841976599,-28.,-7.70051204451168));
#24728=CARTESIAN_POINT('Ctrl Pts',(129.8,-18.4981924307969,4.37121668877661E-15));
#24729=CARTESIAN_POINT('Ctrl Pts',(129.8,-18.4981924307969,1.02942794347193));
#24730=CARTESIAN_POINT('Ctrl Pts',(129.800425634876,-18.8638774763945,3.10110217056979));
#24731=CARTESIAN_POINT('Ctrl Pts',(129.800585502493,-20.5040688923186,5.77582141896866));
#24732=CARTESIAN_POINT('Ctrl Pts',(129.799595280034,-22.9901994383103,7.6330399323527));
#24733=CARTESIAN_POINT('Ctrl Pts',(129.798917565262,-25.6181226009167,8.45634664825776));
#24734=CARTESIAN_POINT('Ctrl Pts',(129.798497161429,-28.0045440318595,8.64969573564895));
#24735=CARTESIAN_POINT('Ctrl Pts',(129.798915409572,-30.0419010743684,8.48314284965744));
#24736=CARTESIAN_POINT('Ctrl Pts',(129.79980293301,-32.6909142565747,7.78606205295877));
#24737=CARTESIAN_POINT('Ctrl Pts',(129.800236816359,-35.0235999478161,6.26044328157787));
#24738=CARTESIAN_POINT('Ctrl Pts',(129.801004712256,-36.8063771223098,3.72609760124849));
#24739=CARTESIAN_POINT('Ctrl Pts',(129.800987139019,-37.6246741986015,1.0561663884385));
#24740=CARTESIAN_POINT('Ctrl Pts',(129.801204967059,-37.440405596014,-2.09611264808735));
#24741=CARTESIAN_POINT('Ctrl Pts',(129.801021929527,-36.1533892376718,-4.96274944615673));
#24742=CARTESIAN_POINT('Ctrl Pts',(129.800421486173,-33.9066423575678,-7.11924690888942));
#24743=CARTESIAN_POINT('Ctrl Pts',(129.799758219885,-31.0743896288208,-8.34843617812973));
#24744=CARTESIAN_POINT('Ctrl Pts',(129.8,-29.0188558496653,-8.59461511716011));
#24745=CARTESIAN_POINT('Ctrl Pts',(129.8,-28.,-8.59461511716011));
#24746=CARTESIAN_POINT('Ctrl Pts',(129.8,-18.1669697220177,4.53337703798322E-15));
#24747=CARTESIAN_POINT('Ctrl Pts',(129.8,-18.1669697220177,1.06646420912009));
#24748=CARTESIAN_POINT('Ctrl Pts',(129.8,-18.5235013453798,3.2144015031083));
#24749=CARTESIAN_POINT('Ctrl Pts',(129.8,-20.1781424757955,6.04867179819866));
#24750=CARTESIAN_POINT('Ctrl Pts',(129.8,-22.7540398357438,8.06622528687979));
#24751=CARTESIAN_POINT('Ctrl Pts',(129.8,-25.5068213458088,8.98108454885427));
#24752=CARTESIAN_POINT('Ctrl Pts',(129.8,-28.0048708711283,9.19767148720769));
#24753=CARTESIAN_POINT('Ctrl Pts',(129.8,-30.1372432217561,9.01104409835271));
#24754=CARTESIAN_POINT('Ctrl Pts',(129.8,-32.912704492555,8.23578485682426));
#24755=CARTESIAN_POINT('Ctrl Pts',(129.8,-35.3359659106613,6.56920417867618));
#24756=CARTESIAN_POINT('Ctrl Pts',(129.8,-37.1469121757438,3.87368039798568));
#24757=CARTESIAN_POINT('Ctrl Pts',(129.8,-37.9534190391165,1.0894602487521));
#24758=CARTESIAN_POINT('Ctrl Pts',(129.8,-37.7745232552706,-2.16589095067385));
#24759=CARTESIAN_POINT('Ctrl Pts',(129.8,-36.4917024138616,-5.17924099653794));
#24760=CARTESIAN_POINT('Ctrl Pts',(129.8,-34.1806914538042,-7.5027269121639));
#24761=CARTESIAN_POINT('Ctrl Pts',(129.8,-31.2194942135712,-8.85890855860159));
#24762=CARTESIAN_POINT('Ctrl Pts',(129.8,-29.0664642091201,-9.13537983414592));
#24763=CARTESIAN_POINT('Ctrl Pts',(129.8,-28.,-9.13537983414592));
#24764=CARTESIAN_POINT('',(129.8,-28.,-9.13537983414592));
#24765=CARTESIAN_POINT('Origin',(131.8,-28.,-9.13537983414592));
#24766=CARTESIAN_POINT('',(129.8,-18.1669697220177,4.71844785465692E-15));
#24767=CARTESIAN_POINT('Ctrl Pts',(129.8,-28.,-9.13537983414592));
#24768=CARTESIAN_POINT('Ctrl Pts',(129.8,-28.2710934566237,-9.13537983414592));
#24769=CARTESIAN_POINT('Ctrl Pts',(129.800000000254,-28.5423900297121,-9.12631611496261));
#24770=CARTESIAN_POINT('Ctrl Pts',(129.800000010001,-28.8129549506681,-9.1080974690796));
#24771=CARTESIAN_POINT('Ctrl Pts',(129.800000012749,-28.8892548171417,-9.1029597733159));
#24772=CARTESIAN_POINT('Ctrl Pts',(129.800000016053,-28.9654968054901,-9.09709411794451));
#24773=CARTESIAN_POINT('Ctrl Pts',(129.800000019417,-29.0416606814196,-9.09049862323265));
#24774=CARTESIAN_POINT('Ctrl Pts',(129.800000030122,-29.284030104473,-9.0695103761331));
#24775=CARTESIAN_POINT('Ctrl Pts',(129.800000031778,-29.5265914722412,-9.04108367787807));
#24776=CARTESIAN_POINT('Ctrl Pts',(129.800000024833,-29.7684741621524,-9.00491149302646));
#24777=CARTESIAN_POINT('Ctrl Pts',(129.800000018035,-30.0052379902963,-8.96950480492925));
#24778=CARTESIAN_POINT('Ctrl Pts',(129.800000005335,-30.2413508050631,-8.92667677470373));
#24779=CARTESIAN_POINT('Ctrl Pts',(129.799999997683,-30.4759872992535,-8.87618791384607));
#24780=CARTESIAN_POINT('Ctrl Pts',(129.799999990032,-30.710623793444,-8.82569905298842));
#24781=CARTESIAN_POINT('Ctrl Pts',(129.799999987709,-30.9437832422619,-8.76754899956281));
#24782=CARTESIAN_POINT('Ctrl Pts',(129.799999993066,-31.1746424139292,-8.70155180091808));
#24783=CARTESIAN_POINT('Ctrl Pts',(129.799999998169,-31.3945493990912,-8.63868557438573));
#24784=CARTESIAN_POINT('Ctrl Pts',(129.800000008838,-31.6123685851659,-8.56869932574673));
#24785=CARTESIAN_POINT('Ctrl Pts',(129.800000024788,-31.827313863548,-8.49162045592886));
#24786=CARTESIAN_POINT('Ctrl Pts',(129.800000040296,-32.0362926162709,-8.41668116813863));
#24787=CARTESIAN_POINT('Ctrl Pts',(129.800000059864,-32.2425542680841,-8.33503768846553));
#24788=CARTESIAN_POINT('Ctrl Pts',(129.800000101707,-32.4453954742136,-8.24676010058969));
#24789=CARTESIAN_POINT('Ctrl Pts',(129.800000128327,-32.5744395368168,-8.19059942794497));
#24790=CARTESIAN_POINT('Ctrl Pts',(129.800000164393,-32.7020996550235,-8.13175463808071));
#24791=CARTESIAN_POINT('Ctrl Pts',(129.80000022104,-32.8282003906212,-8.07025328042285));
#24792=CARTESIAN_POINT('Ctrl Pts',(129.800000300864,-33.0058933182513,-7.98358958061452));
#24793=CARTESIAN_POINT('Ctrl Pts',(129.800000377488,-33.1814457993943,-7.89126827704086));
#24794=CARTESIAN_POINT('Ctrl Pts',(129.800000431821,-33.3542076956327,-7.79326454350896));
#24795=CARTESIAN_POINT('Ctrl Pts',(129.800000484865,-33.5228719225701,-7.69758532075768));
#24796=CARTESIAN_POINT('Ctrl Pts',(129.800000517254,-33.6888758343857,-7.59649010717235));
#24797=CARTESIAN_POINT('Ctrl Pts',(129.800000528243,-33.8516287624338,-7.49000317241242));
#24798=CARTESIAN_POINT('Ctrl Pts',(129.800000533251,-33.9257891309385,-7.44148109408528));
#24799=CARTESIAN_POINT('Ctrl Pts',(129.800000533999,-33.9992747513072,-7.39184019488646));
#24800=CARTESIAN_POINT('Ctrl Pts',(129.80000053125,-34.072031219817,-7.34108608127361));
#24801=CARTESIAN_POINT('Ctrl Pts',(129.800000525348,-34.2282038085113,-7.23214179807585));
#24802=CARTESIAN_POINT('Ctrl Pts',(129.800000502802,-34.3810149199932,-7.11806550802202));
#24803=CARTESIAN_POINT('Ctrl Pts',(129.800000478449,-34.5299490544096,-6.9992289330591));
#24804=CARTESIAN_POINT('Ctrl Pts',(129.800000454184,-34.6783469214609,-6.88082025313308));
#24805=CARTESIAN_POINT('Ctrl Pts',(129.800000428039,-34.8228951901582,-6.75768588000836));
#24806=CARTESIAN_POINT('Ctrl Pts',(129.800000423516,-34.9631160169095,-6.63023387127949));
#24807=CARTESIAN_POINT('Ctrl Pts',(129.800000419042,-35.1018396307111,-6.50414273598408));
#24808=CARTESIAN_POINT('Ctrl Pts',(129.800000435551,-35.2363273181619,-6.3738260917508));
#24809=CARTESIAN_POINT('Ctrl Pts',(129.8000005065,-35.3661544469235,-6.23971268446155));
#24810=CARTESIAN_POINT('Ctrl Pts',(129.800000542169,-35.4314254897008,-6.17228670017229));
#24811=CARTESIAN_POINT('Ctrl Pts',(129.800000591785,-35.4955191647688,-6.10390153542689));
#24812=CARTESIAN_POINT('Ctrl Pts',(129.800000660874,-35.5583856847107,-6.03461443125748));
#24813=CARTESIAN_POINT('Ctrl Pts',(129.800000797243,-35.6824729005216,-5.89785413569915));
#24814=CARTESIAN_POINT('Ctrl Pts',(129.800000888877,-35.8026304832297,-5.75672551648309));
#24815=CARTESIAN_POINT('Ctrl Pts',(129.800000933592,-35.9183208388435,-5.61155087902511));
#24816=CARTESIAN_POINT('Ctrl Pts',(129.800000978028,-36.0332901024865,-5.46728110753362));
#24817=CARTESIAN_POINT('Ctrl Pts',(129.800000976557,-36.1438471657959,-5.31901594976647));
#24818=CARTESIAN_POINT('Ctrl Pts',(129.800000939261,-36.2494959453691,-5.16711228046974));
#24819=CARTESIAN_POINT('Ctrl Pts',(129.800000930872,-36.2732595707179,-5.1329445229163));
#24820=CARTESIAN_POINT('Ctrl Pts',(129.800000920706,-36.2967750114404,-5.09859283065372));
#24821=CARTESIAN_POINT('Ctrl Pts',(129.800000908934,-36.3200368825082,-5.06406152131753));
#24822=CARTESIAN_POINT('Ctrl Pts',(129.800000856842,-36.4229671442463,-4.91126569944354));
#24823=CARTESIAN_POINT('Ctrl Pts',(129.800000772968,-36.5209292387116,-4.7549505850943));
#24824=CARTESIAN_POINT('Ctrl Pts',(129.800000675395,-36.6137381843152,-4.59565457927221));
#24825=CARTESIAN_POINT('Ctrl Pts',(129.800000576889,-36.7074355362313,-4.43483372499716));
#24826=CARTESIAN_POINT('Ctrl Pts',(129.800000464575,-36.79588042377,-4.27097517140965));
#24827=CARTESIAN_POINT('Ctrl Pts',(129.800000359853,-36.8789285269501,-4.1046607860374));
#24828=CARTESIAN_POINT('Ctrl Pts',(129.800000254053,-36.9628311829886,-3.93663504991831));
#24829=CARTESIAN_POINT('Ctrl Pts',(129.800000156076,-37.0412252425313,-3.76610326411397));
#24830=CARTESIAN_POINT('Ctrl Pts',(129.80000008911,-37.1140114128655,-3.59368526445729));
#24831=CARTESIAN_POINT('Ctrl Pts',(129.800000034074,-37.1738304260567,-3.45198424421535));
#24832=CARTESIAN_POINT('Ctrl Pts',(129.8,-37.2298625958302,-3.30900973845834));
#24833=CARTESIAN_POINT('Ctrl Pts',(129.8,-37.2820785495145,-3.16511141418121));
#24834=CARTESIAN_POINT('Ctrl Pts',(129.8,-37.3484560294473,-2.98218632217128));
#24835=CARTESIAN_POINT('Ctrl Pts',(129.800000080133,-37.4091007452409,-2.79654512834284));
#24836=CARTESIAN_POINT('Ctrl Pts',(129.800000206248,-37.4637959430478,-2.60880501888571));
#24837=CARTESIAN_POINT('Ctrl Pts',(129.800000313534,-37.5103245663064,-2.44909650381115));
#24838=CARTESIAN_POINT('Ctrl Pts',(129.800000454017,-37.5525484091508,-2.28786975503681));
#24839=CARTESIAN_POINT('Ctrl Pts',(129.800000603747,-37.5903609896446,-2.12551710040222));
#24840=CARTESIAN_POINT('Ctrl Pts',(129.800000781187,-37.6351715920225,-1.93311763554626));
#24841=CARTESIAN_POINT('Ctrl Pts',(129.800000971388,-37.6737856845845,-1.73913712095642));
#24842=CARTESIAN_POINT('Ctrl Pts',(129.800001132302,-37.7061703661713,-1.54415505986223));
#24843=CARTESIAN_POINT('Ctrl Pts',(129.800001293741,-37.738660806647,-1.34853624444055));
#24844=CARTESIAN_POINT('Ctrl Pts',(129.800001425367,-37.7648810751542,-1.15190984292285));
#24845=CARTESIAN_POINT('Ctrl Pts',(129.800001486965,-37.784850221988,-0.954867005853932));
#24846=CARTESIAN_POINT('Ctrl Pts',(129.800001548546,-37.804813802462,-0.757879094082963));
#24847=CARTESIAN_POINT('Ctrl Pts',(129.800001539778,-37.8185297813407,-0.560475514225451));
#24848=CARTESIAN_POINT('Ctrl Pts',(129.800001427913,-37.8260690978795,-0.363244978850374));
#24849=CARTESIAN_POINT('Ctrl Pts',(129.800001359466,-37.830682188985,-0.242565282781485));
#24850=CARTESIAN_POINT('Ctrl Pts',(129.800001252581,-37.832983833148,-0.121950301222289));
#24851=CARTESIAN_POINT('Ctrl Pts',(129.800001102091,-37.8329997684066,-0.0015332147094816));
#24852=CARTESIAN_POINT('Ctrl Pts',(129.800000850592,-37.8330263993663,0.199707484668333));
#24853=CARTESIAN_POINT('Ctrl Pts',(129.800000660673,-37.8266123822281,0.401429055739714));
#24854=CARTESIAN_POINT('Ctrl Pts',(129.800000514432,-37.8137142562269,0.603017950828346));
#24855=CARTESIAN_POINT('Ctrl Pts',(129.80000040164,-37.8037663599371,0.758496771653588));
#24856=CARTESIAN_POINT('Ctrl Pts',(129.800000314902,-37.7899624204569,0.913896383862366));
#24857=CARTESIAN_POINT('Ctrl Pts',(129.800000247285,-37.7723036328808,1.06893400987562));
#24858=CARTESIAN_POINT('Ctrl Pts',(129.800000159877,-37.7494761710609,1.26935068475925));
#24859=CARTESIAN_POINT('Ctrl Pts',(129.800000104285,-37.7202053021452,1.46916194084438));
#24860=CARTESIAN_POINT('Ctrl Pts',(129.800000068028,-37.6845214547503,1.66772072705263));
#24861=CARTESIAN_POINT('Ctrl Pts',(129.80000003226,-37.6493197354518,1.86359676527837));
#24862=CARTESIAN_POINT('Ctrl Pts',(129.800000015447,-37.6078772734481,2.05825340593417));
#24863=CARTESIAN_POINT('Ctrl Pts',(129.80000000739,-37.5602721024491,2.25108112394059));
#24864=CARTESIAN_POINT('Ctrl Pts',(129.799999999959,-37.5163647521297,2.42893058836005));
#24865=CARTESIAN_POINT('Ctrl Pts',(129.8,-37.467215437465,2.60522401819515));
#24866=CARTESIAN_POINT('Ctrl Pts',(129.8,-37.4129218132307,2.77949806312598));
#24867=CARTESIAN_POINT('Ctrl Pts',(129.8,-37.3553984417258,2.96413909182102));
#24868=CARTESIAN_POINT('Ctrl Pts',(129.800000073857,-37.2917719965685,3.14747629098194));
#24869=CARTESIAN_POINT('Ctrl Pts',(129.800000184787,-37.2220351869846,3.32888387880954));
#24870=CARTESIAN_POINT('Ctrl Pts',(129.800000294156,-37.153279774552,3.50773854098737));
#24871=CARTESIAN_POINT('Ctrl Pts',(129.800000439685,-37.0785848646926,3.68471697306431));
#24872=CARTESIAN_POINT('Ctrl Pts',(129.800000584987,-36.9979923490264,3.85923182135913));
#24873=CARTESIAN_POINT('Ctrl Pts',(129.800000661901,-36.9553317214072,3.9516090464101));
#24874=CARTESIAN_POINT('Ctrl Pts',(129.800000738712,-36.9110194144865,4.04329623882756));
#24875=CARTESIAN_POINT('Ctrl Pts',(129.800000809976,-36.8650671546441,4.13420850839983));
#24876=CARTESIAN_POINT('Ctrl Pts',(129.800000942579,-36.7795634823621,4.30336956664946));
#24877=CARTESIAN_POINT('Ctrl Pts',(129.800001055026,-36.6883793253902,4.46984592494155));
#24878=CARTESIAN_POINT('Ctrl Pts',(129.800001121067,-36.5918570142447,4.63306960800581));
#24879=CARTESIAN_POINT('Ctrl Pts',(129.800001186835,-36.4957337566541,4.79561847309071));
#24880=CARTESIAN_POINT('Ctrl Pts',(129.8000012062,-36.3943167793967,4.95494097982122));
#24881=CARTESIAN_POINT('Ctrl Pts',(129.800001168723,-36.2879846568996,5.11050799627058));
#24882=CARTESIAN_POINT('Ctrl Pts',(129.800001131667,-36.1828466404151,5.26432800057223));
#24883=CARTESIAN_POINT('Ctrl Pts',(129.800001038672,-36.0729036737357,5.41447597179017));
#24884=CARTESIAN_POINT('Ctrl Pts',(129.800000900192,-35.9585552994893,5.56047849998203));
#24885=CARTESIAN_POINT('Ctrl Pts',(129.800000840922,-35.909613657967,5.62296826814189));
#24886=CARTESIAN_POINT('Ctrl Pts',(129.80000077361,-35.8598653835609,5.68469915576676));
#24887=CARTESIAN_POINT('Ctrl Pts',(129.800000700539,-35.8093434235041,5.74563649233914));
#24888=CARTESIAN_POINT('Ctrl Pts',(129.800000634558,-35.7637237600527,5.80066089723016));
#24889=CARTESIAN_POINT('Ctrl Pts',(129.800000575695,-35.7173576466735,5.85516476191921));
#24890=CARTESIAN_POINT('Ctrl Pts',(129.800000523201,-35.6702606155969,5.90911300404228));
#24891=CARTESIAN_POINT('Ctrl Pts',(129.800000390178,-35.5509152099631,6.04581960087493));
#24892=CARTESIAN_POINT('Ctrl Pts',(129.800000297889,-35.4268732339045,6.17895614192948));
#24893=CARTESIAN_POINT('Ctrl Pts',(129.800000232082,-35.2985279351237,6.30821965909818));
#24894=CARTESIAN_POINT('Ctrl Pts',(129.80000016534,-35.1683606080414,6.43931823987149));
#24895=CARTESIAN_POINT('Ctrl Pts',(129.800000125829,-35.0337672516901,6.56643278619385));
#24896=CARTESIAN_POINT('Ctrl Pts',(129.800000100224,-34.8952005298572,6.68928022189627));
#24897=CARTESIAN_POINT('Ctrl Pts',(129.800000074127,-34.7539689311153,6.81449022553994));
#24898=CARTESIAN_POINT('Ctrl Pts',(129.800000062456,-34.608610051288,6.93526709679275));
#24899=CARTESIAN_POINT('Ctrl Pts',(129.800000052925,-34.4596414349555,7.05134961948229));
#24900=CARTESIAN_POINT('Ctrl Pts',(129.800000043317,-34.3094768861733,7.16836406232483));
#24901=CARTESIAN_POINT('Ctrl Pts',(129.800000035855,-34.1556449145912,7.2806082323216));
#24902=CARTESIAN_POINT('Ctrl Pts',(129.800000020148,-33.9987072694013,7.38785752401803));
#24903=CARTESIAN_POINT('Ctrl Pts',(129.800000004335,-33.840706859907,7.49583309600724));
#24904=CARTESIAN_POINT('Ctrl Pts',(129.799999980125,-33.6795591174923,7.59874567871118));
#24905=CARTESIAN_POINT('Ctrl Pts',(129.799999939642,-33.5158612568849,7.6964130662455));
#24906=CARTESIAN_POINT('Ctrl Pts',(129.799999916495,-33.4222649849815,7.75225560032523));
#24907=CARTESIAN_POINT('Ctrl Pts',(129.799999888082,-33.3278354427798,7.80638429637383));
#24908=CARTESIAN_POINT('Ctrl Pts',(129.799999853411,-33.23268668598,7.85877235429687));
#24909=CARTESIAN_POINT('Ctrl Pts',(129.799999781276,-33.0347260541761,7.96776771476434));
#24910=CARTESIAN_POINT('Ctrl Pts',(129.799999677419,-32.8323207055757,8.07008926509624));
#24911=CARTESIAN_POINT('Ctrl Pts',(129.799999565654,-32.6261658853824,8.16533300337038));
#24912=CARTESIAN_POINT('Ctrl Pts',(129.799999487616,-32.482222004947,8.23183522369922));
#24913=CARTESIAN_POINT('Ctrl Pts',(129.799999406892,-32.3364511385822,8.29488741902412));
#24914=CARTESIAN_POINT('Ctrl Pts',(129.799999337055,-32.1891014570786,8.35436170891443));
#24915=CARTESIAN_POINT('Ctrl Pts',(129.799999236438,-31.9768103954567,8.44004808442058));
#24916=CARTESIAN_POINT('Ctrl Pts',(129.799999161317,-31.7612410327654,8.51830550156099));
#24917=CARTESIAN_POINT('Ctrl Pts',(129.799999142915,-31.5432184156714,8.58928340104066));
#24918=CARTESIAN_POINT('Ctrl Pts',(129.799999123369,-31.311641829312,8.6646738347835));
#24919=CARTESIAN_POINT('Ctrl Pts',(129.799999170399,-31.0772979987876,8.73185120061919));
#24920=CARTESIAN_POINT('Ctrl Pts',(129.799999253853,-30.8412069558948,8.7910483680274));
#24921=CARTESIAN_POINT('Ctrl Pts',(129.799999337306,-30.605115913002,8.85024553543562));
#24922=CARTESIAN_POINT('Ctrl Pts',(129.79999945547,-30.3672786267893,8.90146272598421));
#24923=CARTESIAN_POINT('Ctrl Pts',(129.799999505143,-30.1287336314256,8.94498489058459));
#24924=CARTESIAN_POINT('Ctrl Pts',(129.799999540572,-29.9585896989811,8.97602738729393));
#24925=CARTESIAN_POINT('Ctrl Pts',(129.799999538851,-29.7880859291832,9.00315616367553));
#24926=CARTESIAN_POINT('Ctrl Pts',(129.799999455305,-29.6174044031091,9.02642322783757));
#24927=CARTESIAN_POINT('Ctrl Pts',(129.799999350579,-29.4034531173255,9.05558876442715));
#24928=CARTESIAN_POINT('Ctrl Pts',(129.799999255948,-29.1884321010775,9.07885974035984));
#24929=CARTESIAN_POINT('Ctrl Pts',(129.799999182402,-28.9727587444094,9.09626194566826));
#24930=CARTESIAN_POINT('Ctrl Pts',(129.799999107835,-28.754089276615,9.11390590054535));
#24931=CARTESIAN_POINT('Ctrl Pts',(129.799999055151,-28.5347494923584,9.12551691582513));
#24932=CARTESIAN_POINT('Ctrl Pts',(129.799999033247,-28.3151806182946,9.13117521678299));
#24933=CARTESIAN_POINT('Ctrl Pts',(129.799999022883,-28.2112899535657,9.13385248445244));
#24934=CARTESIAN_POINT('Ctrl Pts',(129.799999019353,-28.1073480637685,9.13519783447652));
#24935=CARTESIAN_POINT('Ctrl Pts',(129.799999023188,-28.00340188464,9.13522380628829));
#24936=CARTESIAN_POINT('Ctrl Pts',(129.799999031191,-27.7864545244573,9.13527801237889));
#24937=CARTESIAN_POINT('Ctrl Pts',(129.7999990716,-27.5694888171688,9.12958168360609));
#24938=CARTESIAN_POINT('Ctrl Pts',(129.799999140631,-27.3530624253067,9.11804672246127));
#24939=CARTESIAN_POINT('Ctrl Pts',(129.799999197848,-27.1736750413013,9.10848584364899));
#24940=CARTESIAN_POINT('Ctrl Pts',(129.799999274552,-26.9946582756265,9.0949146064092));
#24941=CARTESIAN_POINT('Ctrl Pts',(129.799999366665,-26.8163256593467,9.07730975400949));
#24942=CARTESIAN_POINT('Ctrl Pts',(129.799999489158,-26.5791782143552,9.05389874903946));
#24943=CARTESIAN_POINT('Ctrl Pts',(129.799999545856,-26.341981406837,9.02318864976405));
#24944=CARTESIAN_POINT('Ctrl Pts',(129.799999563548,-26.1054113455679,8.98495051838404));
#24945=CARTESIAN_POINT('Ctrl Pts',(129.799999569323,-26.0281782992592,8.97246691265732));
#24946=CARTESIAN_POINT('Ctrl Pts',(129.799999571014,-25.9510120755735,8.95918135914482));
#24947=CARTESIAN_POINT('Ctrl Pts',(129.799999569641,-25.8739362147895,8.94508710392248));
#24948=CARTESIAN_POINT('Ctrl Pts',(129.799999565518,-25.642349894167,8.90273873861512));
#24949=CARTESIAN_POINT('Ctrl Pts',(129.799999534226,-25.4115797248202,8.85308564139544));
#24950=CARTESIAN_POINT('Ctrl Pts',(129.799999501623,-25.1825202534547,8.79599159960173));
#24951=CARTESIAN_POINT('Ctrl Pts',(129.799999470053,-24.9607149557348,8.74070569126275));
#24952=CARTESIAN_POINT('Ctrl Pts',(129.799999437428,-24.7405143972207,8.67844279562064));
#24953=CARTESIAN_POINT('Ctrl Pts',(129.799999419512,-24.5227201485777,8.60912629937209));
#24954=CARTESIAN_POINT('Ctrl Pts',(129.799999401972,-24.3094819864445,8.54125985038344));
#24955=CARTESIAN_POINT('Ctrl Pts',(129.799999398573,-24.0985510812376,8.46663187188181));
#24956=CARTESIAN_POINT('Ctrl Pts',(129.799999415083,-23.8906602834359,8.3852152288404));
#24957=CARTESIAN_POINT('Ctrl Pts',(129.799999431062,-23.6894508000853,8.30641520086551));
#24958=CARTESIAN_POINT('Ctrl Pts',(129.79999946563,-23.4910895506826,8.22125598847036));
#24959=CARTESIAN_POINT('Ctrl Pts',(129.799999515702,-23.2962156528616,8.12975391530791));
#24960=CARTESIAN_POINT('Ctrl Pts',(129.799999555263,-23.1422443023712,8.05745743058098));
#24961=CARTESIAN_POINT('Ctrl Pts',(129.799999604328,-22.9904495947184,7.9812020624661));
#24962=CARTESIAN_POINT('Ctrl Pts',(129.799999657982,-22.8411326305199,7.90101415297964));
#24963=CARTESIAN_POINT('Ctrl Pts',(129.799999658949,-22.8384421833811,7.89956929818495));
#24964=CARTESIAN_POINT('Ctrl Pts',(129.799999659917,-22.835752540291,7.89812316708923));
#24965=CARTESIAN_POINT('Ctrl Pts',(129.799999660887,-22.8330637030347,7.89667576089017));
#24966=CARTESIAN_POINT('Ctrl Pts',(129.799999722439,-22.662362016112,7.80478671878978));
#24967=CARTESIAN_POINT('Ctrl Pts',(129.799999764999,-22.4939452362869,7.70717170981652));
#24968=CARTESIAN_POINT('Ctrl Pts',(129.799999830609,-22.3284431873294,7.60404124706532));
#24969=CARTESIAN_POINT('Ctrl Pts',(129.799999896216,-22.1629494633321,7.50091597190547));
#24970=CARTESIAN_POINT('Ctrl Pts',(129.799999986085,-22.0003707418458,7.39227607036555));
#24971=CARTESIAN_POINT('Ctrl Pts',(129.800000113347,-21.8413151221296,7.27837928976005));
#24972=CARTESIAN_POINT('Ctrl Pts',(129.80000023931,-21.6838841539901,7.16564589202987));
#24973=CARTESIAN_POINT('Ctrl Pts',(129.80000040171,-21.5299051675592,7.04776279374741));
#24974=CARTESIAN_POINT('Ctrl Pts',(129.800000577888,-21.3799388716861,6.92502157913105));
#24975=CARTESIAN_POINT('Ctrl Pts',(129.800000752308,-21.2314688855212,6.80350503216388));
#24976=CARTESIAN_POINT('Ctrl Pts',(129.80000093908,-21.0869323471168,6.67722713868374));
#24977=CARTESIAN_POINT('Ctrl Pts',(129.800001091748,-20.9468380388716,6.54650711065002));
#24978=CARTESIAN_POINT('Ctrl Pts',(129.800001241687,-20.809247390563,6.41812321247912));
#24979=CARTESIAN_POINT('Ctrl Pts',(129.800001357032,-20.6759419276993,6.28545484859302));
#24980=CARTESIAN_POINT('Ctrl Pts',(129.800001391451,-20.5473640076158,6.14883492474288));
#24981=CARTESIAN_POINT('Ctrl Pts',(129.800001411037,-20.4741943462765,6.07108881130586));
#24982=CARTESIAN_POINT('Ctrl Pts',(129.800001404497,-20.4025548953712,5.99206356141718));
#24983=CARTESIAN_POINT('Ctrl Pts',(129.800001366462,-20.3325207155241,5.9118244915949));
#24984=CARTESIAN_POINT('Ctrl Pts',(129.80000132551,-20.2571173524217,5.82543387875396));
#24985=CARTESIAN_POINT('Ctrl Pts',(129.80000124789,-20.1835748674122,5.73763626889217));
#24986=CARTESIAN_POINT('Ctrl Pts',(129.800001133642,-20.1119397099029,5.64856846558855));
#24987=CARTESIAN_POINT('Ctrl Pts',(129.800000941388,-19.9913933626716,5.49868677735778));
#24988=CARTESIAN_POINT('Ctrl Pts',(129.800000802801,-19.8755809187763,5.34420807272763));
#24989=CARTESIAN_POINT('Ctrl Pts',(129.800000704905,-19.7648729658217,5.18565120424431));
#24990=CARTESIAN_POINT('Ctrl Pts',(129.800000605327,-19.6522630232855,5.02437029016278));
#24991=CARTESIAN_POINT('Ctrl Pts',(129.800000548124,-19.5449348183843,4.8588703228705));
#24992=CARTESIAN_POINT('Ctrl Pts',(129.80000051896,-19.4432390432031,4.68973446601173));
#24993=CARTESIAN_POINT('Ctrl Pts',(129.800000489668,-19.3410954998061,4.5198539011183));
#24994=CARTESIAN_POINT('Ctrl Pts',(129.800000488609,-19.2446343708263,4.34630591443198));
#24995=CARTESIAN_POINT('Ctrl Pts',(129.800000499014,-19.1541670592512,4.16971083259214));
#24996=CARTESIAN_POINT('Ctrl Pts',(129.800000509398,-19.0638896851603,3.99348651478835));
#24997=CARTESIAN_POINT('Ctrl Pts',(129.800000530948,-18.9795812093161,3.81422846757693));
#24998=CARTESIAN_POINT('Ctrl Pts',(129.800000547183,-18.9015037433399,3.63257374586257));
#24999=CARTESIAN_POINT('Ctrl Pts',(129.800000561419,-18.833039824863,3.47328586551307));
#25000=CARTESIAN_POINT('Ctrl Pts',(129.800000571427,-18.7693663510026,3.31215571629702));
#25001=CARTESIAN_POINT('Ctrl Pts',(129.800000568889,-18.7106279760856,3.14962062448637));
#25002=CARTESIAN_POINT('Ctrl Pts',(129.800000566223,-18.6489651348561,2.97899323524206));
#25003=CARTESIAN_POINT('Ctrl Pts',(129.800000549463,-18.5927410214724,2.80681784335779));
#25004=CARTESIAN_POINT('Ctrl Pts',(129.800000516707,-18.5418874848769,2.63360653112291));
#25005=CARTESIAN_POINT('Ctrl Pts',(129.800000479892,-18.4847332758541,2.4389346123663));
#25006=CARTESIAN_POINT('Ctrl Pts',(129.800000403875,-18.434039176132,2.24191692469441));
#25007=CARTESIAN_POINT('Ctrl Pts',(129.800000328221,-18.3898852098275,2.04317779165805));
#25008=CARTESIAN_POINT('Ctrl Pts',(129.800000250561,-18.3445597096759,1.83916552824253));
#25009=CARTESIAN_POINT('Ctrl Pts',(129.800000174245,-18.3061261971566,1.63333977252411));
#25010=CARTESIAN_POINT('Ctrl Pts',(129.800000119979,-18.2746223705535,1.42640102500768));
#25011=CARTESIAN_POINT('Ctrl Pts',(129.800000064988,-18.2426979670519,1.21669963986911));
#25012=CARTESIAN_POINT('Ctrl Pts',(129.800000032225,-18.2178895579574,1.00585598704665));
#25013=CARTESIAN_POINT('Ctrl Pts',(129.800000016489,-18.2001851255581,0.794615559855742));
#25014=CARTESIAN_POINT('Ctrl Pts',(129.800000000526,-18.182223881897,0.580310989210295));
#25015=CARTESIAN_POINT('Ctrl Pts',(129.800000000194,-18.1715742168204,0.365598745704213));
#25016=CARTESIAN_POINT('Ctrl Pts',(129.80000000003,-18.1681706704168,0.151263981325619));
#25017=CARTESIAN_POINT('Ctrl Pts',(129.799999999991,-18.1673696146262,0.100818333234996));
#25018=CARTESIAN_POINT('Ctrl Pts',(129.8,-18.1669697220177,0.050393597992155));
#25019=CARTESIAN_POINT('Ctrl Pts',(129.8,-18.1669697220177,4.53337703798322E-15));
#25020=CARTESIAN_POINT('Origin',(131.8,-18.1669697220177,4.71844785465692E-15));
#25021=CARTESIAN_POINT('Ctrl Pts',(132.432701479047,-28.,-7.23809523809524));
#25022=CARTESIAN_POINT('Ctrl Pts',(132.432701479047,-26.8009816752416,-7.23809523809524));
#25023=CARTESIAN_POINT('Ctrl Pts',(132.26645359153,-25.0007435382869,-6.85507520667426));
#25024=CARTESIAN_POINT('Ctrl Pts',(131.781589365556,-22.5441190611736,-5.46533378045002));
#25025=CARTESIAN_POINT('Ctrl Pts',(131.341321658826,-21.023111279012,-3.82480829163835));
#25026=CARTESIAN_POINT('Ctrl Pts',(131.053974250738,-20.1562205092697,-1.73171255809164));
#25027=CARTESIAN_POINT('Ctrl Pts',(131.,-20.,-0.573980617392535));
#25028=CARTESIAN_POINT('Ctrl Pts',(131.,-20.,3.98986399474666E-15));
#25029=CARTESIAN_POINT('Ctrl Pts',(132.090706623172,-28.,-7.12404769267737));
#25030=CARTESIAN_POINT('Ctrl Pts',(132.090706623172,-26.8143903768838,-7.12404769267737));
#25031=CARTESIAN_POINT('Ctrl Pts',(131.929220024804,-25.032371992221,-6.78231349114718));
#25032=CARTESIAN_POINT('Ctrl Pts',(131.480860519403,-22.5478129793514,-5.47666315644241));
#25033=CARTESIAN_POINT('Ctrl Pts',(131.091394358315,-20.9713812405232,-3.8623482138183));
#25034=CARTESIAN_POINT('Ctrl Pts',(130.843813934656,-20.0728982691064,-1.75132320290942));
#25035=CARTESIAN_POINT('Ctrl Pts',(130.797619582017,-19.9116739443255,-0.580551775628326));
#25036=CARTESIAN_POINT('Ctrl Pts',(130.797619582017,-19.9116739443255,4.00881225491749E-15));
#25037=CARTESIAN_POINT('Ctrl Pts',(131.345671187872,-28.,-7.08620083875834));
#25038=CARTESIAN_POINT('Ctrl Pts',(131.345671187872,-26.818798622422,-7.08620083875834));
#25039=CARTESIAN_POINT('Ctrl Pts',(131.217018773873,-25.0379511743519,-6.80862333715474));
#25040=CARTESIAN_POINT('Ctrl Pts',(130.885776810888,-22.4629637836557,-5.6034495189424));
#25041=CARTESIAN_POINT('Ctrl Pts',(130.616860535725,-20.7817899251647,-3.98402852846389));
#25042=CARTESIAN_POINT('Ctrl Pts',(130.453039217185,-19.8354212605226,-1.80583906043873));
#25043=CARTESIAN_POINT('Ctrl Pts',(130.4226711313,-19.6673356519921,-0.598748896272704));
#25044=CARTESIAN_POINT('Ctrl Pts',(130.4226711313,-19.6673356519921,4.13658632801098E-15));
#25045=CARTESIAN_POINT('Ctrl Pts',(130.187837825679,-28.,-7.70051010024203));
#25046=CARTESIAN_POINT('Ctrl Pts',(130.187837825679,-26.7469538948703,-7.70051010024203));
#25047=CARTESIAN_POINT('Ctrl Pts',(130.149022478866,-24.8470535326785,-7.43645293090163));
#25048=CARTESIAN_POINT('Ctrl Pts',(130.056596105886,-22.0269455952546,-6.14421728129872));
#25049=CARTESIAN_POINT('Ctrl Pts',(129.987591470929,-20.1995226886221,-4.33137686974819));
#25050=CARTESIAN_POINT('Ctrl Pts',(129.947669172038,-19.2197159043987,-1.94474772386544));
#25051=CARTESIAN_POINT('Ctrl Pts',(129.94039562733,-19.0495950039424,-0.644745782382747));
#25052=CARTESIAN_POINT('Ctrl Pts',(129.94039562733,-19.0495950039424,4.64941528572959E-15));
#25053=CARTESIAN_POINT('Ctrl Pts',(129.8,-28.,-8.59461511716011));
#25054=CARTESIAN_POINT('Ctrl Pts',(129.8,-26.6424865111779,-8.59461511716011));
#25055=CARTESIAN_POINT('Ctrl Pts',(129.799352153585,-24.5784055571512,-8.26261724319198));
#25056=CARTESIAN_POINT('Ctrl Pts',(129.800907688529,-21.5374980704997,-6.72536392331271));
#25057=CARTESIAN_POINT('Ctrl Pts',(129.800369726049,-19.6351532628125,-4.65866809558641));
#25058=CARTESIAN_POINT('Ctrl Pts',(129.800544621058,-18.6635321684884,-2.06928349402084));
#25059=CARTESIAN_POINT('Ctrl Pts',(129.8,-18.4981924307969,-0.685799821188036));
#25060=CARTESIAN_POINT('Ctrl Pts',(129.8,-18.4981924307969,5.22539942166253E-15));
#25061=CARTESIAN_POINT('Ctrl Pts',(129.8,-28.,-9.13537983414593));
#25062=CARTESIAN_POINT('Ctrl Pts',(129.8,-26.5790536024284,-9.13537983414592));
#25063=CARTESIAN_POINT('Ctrl Pts',(129.8,-24.4156431485582,-8.76163646629594));
#25064=CARTESIAN_POINT('Ctrl Pts',(129.8,-21.242356094889,-7.07450440768049));
#25065=CARTESIAN_POINT('Ctrl Pts',(129.8,-19.2957674742455,-4.85510844114429));
#25066=CARTESIAN_POINT('Ctrl Pts',(129.8,-18.3293873963884,-2.14384019547752));
#25067=CARTESIAN_POINT('Ctrl Pts',(129.8,-18.1669697220177,-0.710473198785783));
#25068=CARTESIAN_POINT('Ctrl Pts',(129.8,-18.1669697220177,5.60575888572018E-15));
#25069=CARTESIAN_POINT('Ctrl Pts',(129.8,-18.1669697220177,5.60575888572018E-15));
#25070=CARTESIAN_POINT('Ctrl Pts',(129.8,-18.1669697220177,-0.710473198785783));
#25071=CARTESIAN_POINT('Ctrl Pts',(129.8,-18.3293873963884,-2.14384019547752));
#25072=CARTESIAN_POINT('Ctrl Pts',(129.8,-19.2957674742455,-4.85510844114429));
#25073=CARTESIAN_POINT('Ctrl Pts',(129.8,-21.242356094889,-7.07450440768049));
#25074=CARTESIAN_POINT('Ctrl Pts',(129.8,-24.4156431485582,-8.76163646629594));
#25075=CARTESIAN_POINT('Ctrl Pts',(129.8,-26.5790536024284,-9.13537983414592));
#25076=CARTESIAN_POINT('Ctrl Pts',(129.8,-28.,-9.13537983414593));
#25077=CARTESIAN_POINT('Origin',(129.8,16.6,0.));
#25078=CARTESIAN_POINT('',(129.8,-16.6,-2.03291368658461E-15));
#25079=CARTESIAN_POINT('Origin',(129.8,0.,0.));
#25080=CARTESIAN_POINT('Origin',(160.,-32.,-32.));
#25081=CARTESIAN_POINT('',(160.,-41.8103991881704,-58.2251037704095));
#25082=CARTESIAN_POINT('Origin',(160.,-32.,-32.));
#25083=CARTESIAN_POINT('',(162.,-42.9545404089977,-55.579610777696));
#25084=CARTESIAN_POINT('Ctrl Pts',(162.,-42.9545404089977,-55.579610777696));
#25085=CARTESIAN_POINT('Ctrl Pts',(162.,-43.0271281214294,-55.7530160455202));
#25086=CARTESIAN_POINT('Ctrl Pts',(161.973573983972,-43.0736878043345,-55.9328516982979));
#25087=CARTESIAN_POINT('Ctrl Pts',(161.868475569496,-43.1203520588171,-56.3211207154451));
#25088=CARTESIAN_POINT('Ctrl Pts',(161.784372185244,-43.1115565863127,-56.522998392291));
#25089=CARTESIAN_POINT('Ctrl Pts',(161.547930236135,-43.0311442891192,-56.9623937955494));
#25090=CARTESIAN_POINT('Ctrl Pts',(161.383204155006,-42.9404796484396,-57.1887874178576));
#25091=CARTESIAN_POINT('Ctrl Pts',(161.02783774489,-42.7034153293614,-57.5819163169907));
#25092=CARTESIAN_POINT('Ctrl Pts',(160.835005517045,-42.5553839363861,-57.7505434494708));
#25093=CARTESIAN_POINT('Ctrl Pts',(160.431659980245,-42.2166967899328,-58.0327463433367));
#25094=CARTESIAN_POINT('Ctrl Pts',(160.218422653963,-42.0224470249448,-58.1450131095542));
#25095=CARTESIAN_POINT('Ctrl Pts',(160.004130040426,-41.8144122444641,-58.2235988717642));
#25096=CARTESIAN_POINT('Ctrl Pts',(160.002065019734,-41.812406319229,-58.2243529342229));
#25097=CARTESIAN_POINT('Ctrl Pts',(160.,-41.8103991881673,-58.2251037704106));
#25098=CARTESIAN_POINT('Origin',(162.,-32.,-32.));
#25099=CARTESIAN_POINT('Origin',(162.,-45.,-45.));
#25100=CARTESIAN_POINT('',(162.,-41.7580469908461,-54.4599017271026));
#25101=CARTESIAN_POINT('Origin',(162.,-41.1096563890154,-56.3518820725231));
#25102=CARTESIAN_POINT('Origin',(162.,-45.,-45.));
#25103=CARTESIAN_POINT('',(162.,-45.,-38.5));
#25104=CARTESIAN_POINT('Origin',(162.,-45.,-45.));
#25105=CARTESIAN_POINT('Origin',(160.,-32.,32.));
#25106=CARTESIAN_POINT('',(160.,-58.153393661244,42.));
#25107=CARTESIAN_POINT('',(162.,-55.5753783097334,42.9636461796681));
#25108=CARTESIAN_POINT('Ctrl Pts',(162.,-55.5753783097334,42.9636461796681));
#25109=CARTESIAN_POINT('Ctrl Pts',(162.,-55.6734613307539,43.0052418396728));
#25110=CARTESIAN_POINT('Ctrl Pts',(161.991497625313,-55.774572253448,43.0388739116958));
#25111=CARTESIAN_POINT('Ctrl Pts',(161.943944452234,-56.0679790385642,43.1111756115417));
#25112=CARTESIAN_POINT('Ctrl Pts',(161.886488114777,-56.257458287516,43.1282512264031));
#25113=CARTESIAN_POINT('Ctrl Pts',(161.713845454435,-56.6687617144824,43.1110662555161));
#25114=CARTESIAN_POINT('Ctrl Pts',(161.589392283786,-56.8825885356347,43.0628215369467));
#25115=CARTESIAN_POINT('Ctrl Pts',(161.260245422218,-57.3380017544373,42.8875266559234));
#25116=CARTESIAN_POINT('Ctrl Pts',(161.041527470277,-57.5632038812665,42.7369834456557));
#25117=CARTESIAN_POINT('Ctrl Pts',(160.689312921863,-57.8437159943844,42.4663518758168));
#25118=CARTESIAN_POINT('Ctrl Pts',(160.563162669358,-57.9294120770491,42.3637163836509));
#25119=CARTESIAN_POINT('Ctrl Pts',(160.344401686438,-58.0513270922311,42.1875089376441));
#25120=CARTESIAN_POINT('Ctrl Pts',(160.263056078934,-58.0887104512742,42.1229599723016));
#25121=CARTESIAN_POINT('Ctrl Pts',(160.155587043591,-58.1276579654234,42.0513407387634));
#25122=CARTESIAN_POINT('Ctrl Pts',(160.11788316197,-58.1386506822474,42.0296954878548));
#25123=CARTESIAN_POINT('Ctrl Pts',(160.053942941167,-58.1506706840953,42.0056317234313));
#25124=CARTESIAN_POINT('Ctrl Pts',(160.028265792271,-58.1531925095842,42.0004118971055));
#25125=CARTESIAN_POINT('Ctrl Pts',(160.002031326826,-58.1533898527096,42.0000077985377));
#25126=CARTESIAN_POINT('Ctrl Pts',(160.001014693341,-58.1533936622468,41.9999999973774));
#25127=CARTESIAN_POINT('Ctrl Pts',(160.,-58.1533936622468,41.9999999973774));
#25128=CARTESIAN_POINT('',(162.,-42.9545404089977,55.579610777696));
#25129=CARTESIAN_POINT('Origin',(162.,-32.,32.));
#25130=CARTESIAN_POINT('',(160.,-41.8103991881704,58.2251037704095));
#25131=CARTESIAN_POINT('Ctrl Pts',(160.,-41.8103991881673,58.2251037704106));
#25132=CARTESIAN_POINT('Ctrl Pts',(160.002065019732,-41.8124063192265,58.2243529342238));
#25133=CARTESIAN_POINT('Ctrl Pts',(160.004130040429,-41.8144122444637,58.2235988717643));
#25134=CARTESIAN_POINT('Ctrl Pts',(160.218422653916,-42.022447024985,58.1450131095393));
#25135=CARTESIAN_POINT('Ctrl Pts',(160.431659980247,-42.2166967899343,58.0327463433355));
#25136=CARTESIAN_POINT('Ctrl Pts',(160.835005517045,-42.5553839363861,57.7505434494708));
#25137=CARTESIAN_POINT('Ctrl Pts',(161.02783774489,-42.7034153293614,57.5819163169908));
#25138=CARTESIAN_POINT('Ctrl Pts',(161.383204155006,-42.9404796484396,57.1887874178575));
#25139=CARTESIAN_POINT('Ctrl Pts',(161.547930236135,-43.0311442891192,56.9623937955494));
#25140=CARTESIAN_POINT('Ctrl Pts',(161.784372185244,-43.1115565863127,56.5229983922909));
#25141=CARTESIAN_POINT('Ctrl Pts',(161.868475569496,-43.1203520588171,56.3211207154451));
#25142=CARTESIAN_POINT('Ctrl Pts',(161.973573983972,-43.0736878043345,55.9328516982979));
#25143=CARTESIAN_POINT('Ctrl Pts',(162.,-43.0271281214294,55.7530160455202));
#25144=CARTESIAN_POINT('Ctrl Pts',(162.,-42.9545404089977,55.579610777696));
#25145=CARTESIAN_POINT('Origin',(160.,-32.,32.));
#25146=CARTESIAN_POINT('Origin',(125.8,-32.,32.));
#25147=CARTESIAN_POINT('',(173.,-41.8103991881704,58.2251037704095));
#25148=CARTESIAN_POINT('',(125.8,-41.8103991881704,58.2251037704095));
#25149=CARTESIAN_POINT('',(173.,-32.,60.));
#25150=CARTESIAN_POINT('Origin',(173.,-32.,32.));
#25151=CARTESIAN_POINT('',(127.8,-32.,60.));
#25152=CARTESIAN_POINT('',(125.8,-32.,60.));
#25153=CARTESIAN_POINT('Origin',(127.8,-32.,32.));
#25154=CARTESIAN_POINT('',(125.8,-58.153393661244,42.));
#25155=CARTESIAN_POINT('Origin',(160.,32.,-32.));
#25156=CARTESIAN_POINT('',(160.,58.2251037704095,-41.8103991881704));
#25157=CARTESIAN_POINT('',(162.,55.579610777696,-42.9545404089977));
#25158=CARTESIAN_POINT('Ctrl Pts',(162.,55.579610777696,-42.9545404089977));
#25159=CARTESIAN_POINT('Ctrl Pts',(162.,55.7530160455202,-43.0271281214294));
#25160=CARTESIAN_POINT('Ctrl Pts',(161.973573983972,55.9328516982979,-43.0736878043345));
#25161=CARTESIAN_POINT('Ctrl Pts',(161.868475569496,56.3211207154452,-43.1203520588171));
#25162=CARTESIAN_POINT('Ctrl Pts',(161.784372185244,56.522998392291,-43.1115565863127));
#25163=CARTESIAN_POINT('Ctrl Pts',(161.547930236135,56.9623937955493,-43.0311442891192));
#25164=CARTESIAN_POINT('Ctrl Pts',(161.383204155006,57.1887874178575,-42.9404796484396));
#25165=CARTESIAN_POINT('Ctrl Pts',(161.027837744889,57.5819163169916,-42.7034153293609));
#25166=CARTESIAN_POINT('Ctrl Pts',(160.835005517043,57.7505434494722,-42.5553839363849));
#25167=CARTESIAN_POINT('Ctrl Pts',(160.431659980243,58.0327463433376,-42.2166967899313));
#25168=CARTESIAN_POINT('Ctrl Pts',(160.218422653911,58.1450131095417,-42.0224470249804));
#25169=CARTESIAN_POINT('Ctrl Pts',(160.004130040426,58.2235988717657,-41.8144122444601));
#25170=CARTESIAN_POINT('Ctrl Pts',(160.00206501973,58.2243529342232,-41.8124063192281));
#25171=CARTESIAN_POINT('Ctrl Pts',(160.,58.2251037704095,-41.8103991881704));
#25172=CARTESIAN_POINT('',(162.,42.9545404089977,-55.579610777696));
#25173=CARTESIAN_POINT('Origin',(162.,32.,-32.));
#25174=CARTESIAN_POINT('',(160.,41.8103991881704,-58.2251037704095));
#25175=CARTESIAN_POINT('Ctrl Pts',(160.,41.8103991881704,-58.2251037704095));
#25176=CARTESIAN_POINT('Ctrl Pts',(160.002065019731,41.8124063192286,-58.224352934223));
#25177=CARTESIAN_POINT('Ctrl Pts',(160.004130040425,41.8144122444596,-58.2235988717659));
#25178=CARTESIAN_POINT('Ctrl Pts',(160.218422653911,42.0224470249804,-58.1450131095417));
#25179=CARTESIAN_POINT('Ctrl Pts',(160.431659980243,42.2166967899313,-58.0327463433376));
#25180=CARTESIAN_POINT('Ctrl Pts',(160.835005517043,42.5553839363849,-57.7505434494722));
#25181=CARTESIAN_POINT('Ctrl Pts',(161.027837744889,42.7034153293609,-57.5819163169915));
#25182=CARTESIAN_POINT('Ctrl Pts',(161.383204155006,42.9404796484396,-57.1887874178575));
#25183=CARTESIAN_POINT('Ctrl Pts',(161.547930236135,43.0311442891192,-56.9623937955494));
#25184=CARTESIAN_POINT('Ctrl Pts',(161.784372185244,43.1115565863127,-56.522998392291));
#25185=CARTESIAN_POINT('Ctrl Pts',(161.868475569496,43.1203520588171,-56.3211207154451));
#25186=CARTESIAN_POINT('Ctrl Pts',(161.973573983972,43.0736878043345,-55.9328516982979));
#25187=CARTESIAN_POINT('Ctrl Pts',(162.,43.0271281214294,-55.7530160455202));
#25188=CARTESIAN_POINT('Ctrl Pts',(162.,42.9545404089977,-55.579610777696));
#25189=CARTESIAN_POINT('Origin',(160.,32.,-32.));
#25190=CARTESIAN_POINT('Origin',(162.,45.,-45.));
#25191=CARTESIAN_POINT('',(162.,54.4599017271026,-41.7580469908461));
#25192=CARTESIAN_POINT('Origin',(162.,56.3518820725231,-41.1096563890154));
#25193=CARTESIAN_POINT('',(162.,41.7580469908461,-54.4599017271026));
#25194=CARTESIAN_POINT('Origin',(162.,45.,-45.));
#25195=CARTESIAN_POINT('Origin',(162.,41.1096563890154,-56.3518820725231));
#25196=CARTESIAN_POINT('',(162.,45.,-38.5));
#25197=CARTESIAN_POINT('Origin',(162.,45.,-45.));
#25198=CARTESIAN_POINT('Origin',(160.,32.,32.));
#25199=CARTESIAN_POINT('',(160.,41.8103991881704,58.2251037704095));
#25200=CARTESIAN_POINT('',(162.,42.9545404089977,55.579610777696));
#25201=CARTESIAN_POINT('Ctrl Pts',(162.,42.9545404089977,55.579610777696));
#25202=CARTESIAN_POINT('Ctrl Pts',(162.,43.0271281214294,55.7530160455202));
#25203=CARTESIAN_POINT('Ctrl Pts',(161.973573983972,43.0736878043345,55.9328516982979));
#25204=CARTESIAN_POINT('Ctrl Pts',(161.868475569496,43.1203520588171,56.3211207154451));
#25205=CARTESIAN_POINT('Ctrl Pts',(161.784372185244,43.1115565863127,56.522998392291));
#25206=CARTESIAN_POINT('Ctrl Pts',(161.547930236135,43.0311442891192,56.9623937955494));
#25207=CARTESIAN_POINT('Ctrl Pts',(161.383204155006,42.9404796484396,57.1887874178576));
#25208=CARTESIAN_POINT('Ctrl Pts',(161.027837744889,42.7034153293609,57.5819163169915));
#25209=CARTESIAN_POINT('Ctrl Pts',(160.835005517043,42.5553839363849,57.7505434494722));
#25210=CARTESIAN_POINT('Ctrl Pts',(160.431659980243,42.2166967899312,58.0327463433376));
#25211=CARTESIAN_POINT('Ctrl Pts',(160.218422653911,42.0224470249804,58.1450131095417));
#25212=CARTESIAN_POINT('Ctrl Pts',(160.004130040425,41.8144122444596,58.2235988717659));
#25213=CARTESIAN_POINT('Ctrl Pts',(160.002065019731,41.8124063192286,58.224352934223));
#25214=CARTESIAN_POINT('Ctrl Pts',(160.,41.8103991881704,58.2251037704095));
#25215=CARTESIAN_POINT('',(162.,55.579610777696,42.9545404089977));
#25216=CARTESIAN_POINT('Origin',(162.,32.,32.));
#25217=CARTESIAN_POINT('',(160.,58.2251037704095,41.8103991881704));
#25218=CARTESIAN_POINT('Ctrl Pts',(160.,58.2251037704095,41.8103991881704));
#25219=CARTESIAN_POINT('Ctrl Pts',(160.00206501973,58.2243529342232,41.8124063192281));
#25220=CARTESIAN_POINT('Ctrl Pts',(160.004130040426,58.2235988717657,41.8144122444601));
#25221=CARTESIAN_POINT('Ctrl Pts',(160.218422653911,58.1450131095417,42.0224470249804));
#25222=CARTESIAN_POINT('Ctrl Pts',(160.431659980243,58.0327463433376,42.2166967899313));
#25223=CARTESIAN_POINT('Ctrl Pts',(160.835005517043,57.7505434494722,42.5553839363849));
#25224=CARTESIAN_POINT('Ctrl Pts',(161.027837744889,57.5819163169915,42.7034153293609));
#25225=CARTESIAN_POINT('Ctrl Pts',(161.383204155006,57.1887874178575,42.9404796484396));
#25226=CARTESIAN_POINT('Ctrl Pts',(161.547930236135,56.9623937955494,43.0311442891192));
#25227=CARTESIAN_POINT('Ctrl Pts',(161.784372185244,56.522998392291,43.1115565863127));
#25228=CARTESIAN_POINT('Ctrl Pts',(161.868475569496,56.3211207154451,43.1203520588171));
#25229=CARTESIAN_POINT('Ctrl Pts',(161.973573983972,55.9328516982979,43.0736878043345));
#25230=CARTESIAN_POINT('Ctrl Pts',(162.,55.7530160455202,43.0271281214294));
#25231=CARTESIAN_POINT('Ctrl Pts',(162.,55.579610777696,42.9545404089977));
#25232=CARTESIAN_POINT('Origin',(160.,32.,32.));
#25233=CARTESIAN_POINT('Origin',(162.,45.,45.));
#25234=CARTESIAN_POINT('',(162.,41.7580469908461,54.4599017271026));
#25235=CARTESIAN_POINT('Origin',(162.,41.1096563890154,56.3518820725231));
#25236=CARTESIAN_POINT('',(162.,54.4599017271026,41.7580469908461));
#25237=CARTESIAN_POINT('Origin',(162.,45.,45.));
#25238=CARTESIAN_POINT('Origin',(162.,56.3518820725231,41.1096563890154));
#25239=CARTESIAN_POINT('',(162.,45.,51.5));
#25240=CARTESIAN_POINT('Origin',(162.,45.,45.));
#25241=CARTESIAN_POINT('Origin',(127.8,16.,58.));
#25242=CARTESIAN_POINT('',(127.8,32.,60.));
#25243=CARTESIAN_POINT('Origin',(127.8,32.,58.));
#25244=CARTESIAN_POINT('Origin',(127.8,-32.,58.));
#25245=CARTESIAN_POINT('',(127.8,16.,60.));
#25246=CARTESIAN_POINT('Origin',(127.8,-32.,32.));
#25247=CARTESIAN_POINT('Origin',(127.8,32.,32.));
#25248=CARTESIAN_POINT('Origin',(127.8,32.,32.));
#25249=CARTESIAN_POINT('Origin',(125.8,32.,32.));
#25250=CARTESIAN_POINT('',(173.,58.2251037704095,41.8103991881704));
#25251=CARTESIAN_POINT('',(125.8,58.2251037704095,41.8103991881704));
#25252=CARTESIAN_POINT('Origin',(173.,32.,32.));
#25253=CARTESIAN_POINT('',(125.8,59.9821371592664,33.));
#25254=CARTESIAN_POINT('',(173.,32.,60.));
#25255=CARTESIAN_POINT('',(125.8,32.,60.));
#25256=CARTESIAN_POINT('',(173.,41.8103991881704,58.2251037704095));
#25257=CARTESIAN_POINT('Origin',(173.,32.,32.));
#25258=CARTESIAN_POINT('',(125.8,41.8103991881704,58.2251037704095));
#25259=CARTESIAN_POINT('Origin',(125.8,32.,60.));
#25260=CARTESIAN_POINT('',(173.,16.,60.));
#25261=CARTESIAN_POINT('Origin',(173.,-32.,-32.));
#25262=CARTESIAN_POINT('',(173.,-32.,-60.));
#25263=CARTESIAN_POINT('Origin',(173.,-32.,-58.));
#25264=CARTESIAN_POINT('',(173.,-41.8103991881704,-58.2251037704095));
#25265=CARTESIAN_POINT('Origin',(173.,-41.1096563890154,-56.3518820725231));
#25266=CARTESIAN_POINT('Origin',(173.,-32.,-32.));
#25267=CARTESIAN_POINT('Origin',(173.,-16.,-58.));
#25268=CARTESIAN_POINT('',(173.,32.,-60.));
#25269=CARTESIAN_POINT('Origin',(173.,32.,-58.));
#25270=CARTESIAN_POINT('',(173.,-16.,-60.));
#25271=CARTESIAN_POINT('Origin',(173.,32.,-32.));
#25272=CARTESIAN_POINT('',(173.,41.8103991881704,-58.2251037704095));
#25273=CARTESIAN_POINT('Origin',(173.,41.1096563890154,-56.3518820725231));
#25274=CARTESIAN_POINT('Origin',(173.,32.,-32.));
#25275=CARTESIAN_POINT('Origin',(173.,41.1096563890154,-56.3518820725231));
#25276=CARTESIAN_POINT('',(173.,41.7580469908461,-54.4599017271026));
#25277=CARTESIAN_POINT('Origin',(173.,41.1096563890154,-56.3518820725231));
#25278=CARTESIAN_POINT('Origin',(173.,41.1096563890154,-56.3518820725231));
#25279=CARTESIAN_POINT('Origin',(173.,-41.1096563890154,-56.3518820725231));
#25280=CARTESIAN_POINT('',(173.,-41.7580469908461,-54.4599017271026));
#25281=CARTESIAN_POINT('Origin',(173.,-41.1096563890154,-56.3518820725231));
#25282=CARTESIAN_POINT('Origin',(173.,-41.1096563890154,-56.3518820725231));
#25283=CARTESIAN_POINT('Origin',(173.,45.,-45.));
#25284=CARTESIAN_POINT('',(173.,54.4599017271026,-41.7580469908461));
#25285=CARTESIAN_POINT('Origin',(173.,45.,-45.));
#25286=CARTESIAN_POINT('Origin',(173.,56.3518820725231,-41.1096563890154));
#25287=CARTESIAN_POINT('Origin',(125.8,41.1096563890154,-56.3518820725231));
#25288=CARTESIAN_POINT('',(125.8,41.8103991881704,-58.2251037704095));
#25289=CARTESIAN_POINT('',(125.8,41.7580469908461,-54.4599017271026));
#25290=CARTESIAN_POINT('Origin',(125.8,32.,-32.));
#25291=CARTESIAN_POINT('',(173.,58.2251037704095,-41.8103991881704));
#25292=CARTESIAN_POINT('Origin',(173.,32.,-32.));
#25293=CARTESIAN_POINT('',(125.8,58.2251037704095,-41.8103991881704));
#25294=CARTESIAN_POINT('',(125.8,32.,-60.));
#25295=CARTESIAN_POINT('Origin',(125.8,-32.,-60.));
#25296=CARTESIAN_POINT('',(125.8,-32.,-60.));
#25297=CARTESIAN_POINT('Origin',(125.8,-32.,-32.));
#25298=CARTESIAN_POINT('',(125.8,-41.8103991881704,-58.2251037704095));
#25299=CARTESIAN_POINT('Origin',(173.,-30.,40.));
#25300=CARTESIAN_POINT('',(173.,-58.153393661244,42.));
#25301=CARTESIAN_POINT('Ctrl Pts',(173.,-58.1533936609661,42.));
#25302=CARTESIAN_POINT('Ctrl Pts',(173.167046229782,-58.1533936609661,42.));
#25303=CARTESIAN_POINT('Ctrl Pts',(173.335981739515,-58.164172163974,41.9788285866254));
#25304=CARTESIAN_POINT('Ctrl Pts',(173.663743266442,-58.2018772085049,41.8942257523252));
#25305=CARTESIAN_POINT('Ctrl Pts',(173.822610223296,-58.2285507903109,41.8308404000117));
#25306=CARTESIAN_POINT('Ctrl Pts',(174.118673603566,-58.2827371839977,41.6665038929614));
#25307=CARTESIAN_POINT('Ctrl Pts',(174.256201391015,-58.3101344177017,41.5653968322566));
#25308=CARTESIAN_POINT('Ctrl Pts',(174.420873583764,-58.3360427437949,41.4087347797136));
#25309=CARTESIAN_POINT('Ctrl Pts',(174.461424720572,-58.3417521272735,41.3666159110033));
#25310=CARTESIAN_POINT('Ctrl Pts',(174.499999999851,-58.3461592103039,41.3228756557013));
#25311=CARTESIAN_POINT('',(173.,-30.,42.));
#25312=CARTESIAN_POINT('Origin',(150.4,-60.,42.));
#25313=CARTESIAN_POINT('',(125.8,-58.153393661244,42.));
#25314=CARTESIAN_POINT('Origin',(173.,26.5,-31.));
#25315=CARTESIAN_POINT('Origin',(173.,64.,-31.));
#25316=CARTESIAN_POINT('Ctrl Pts',(173.,59.9821371592664,-33.));
#25317=CARTESIAN_POINT('Ctrl Pts',(173.100941314786,59.9821371592664,-33.));
#25318=CARTESIAN_POINT('Ctrl Pts',(173.20122849925,59.9747656314413,-32.9923574576679));
#25319=CARTESIAN_POINT('Ctrl Pts',(173.448747816884,59.9385021348617,-32.9548041970754));
#25320=CARTESIAN_POINT('Ctrl Pts',(173.591032753534,59.9010691778161,-32.9160577581803));
#25321=CARTESIAN_POINT('Ctrl Pts',(173.946053385859,59.7672434939636,-32.7780158331181));
#25322=CARTESIAN_POINT('Ctrl Pts',(174.150696148371,59.6459583395498,-32.6532332234613));
#25323=CARTESIAN_POINT('Ctrl Pts',(174.50787466907,59.3337989076212,-32.3354122100756));
#25324=CARTESIAN_POINT('Ctrl Pts',(174.647363992728,59.1545342172527,-32.1543180026668));
#25325=CARTESIAN_POINT('Ctrl Pts',(174.914204977564,58.6701679370831,-31.6705622009276));
#25326=CARTESIAN_POINT('Ctrl Pts',(174.999017799315,58.3344432492769,-31.3404083795624));
#25327=CARTESIAN_POINT('Ctrl Pts',(174.999997177196,57.9847942903201,-31.0038801897555));
#25328=CARTESIAN_POINT('Ctrl Pts',(175.,57.9827782576495,-31.0019400355805));
#25329=CARTESIAN_POINT('Ctrl Pts',(175.,57.9807621135332,-31.));
#25330=CARTESIAN_POINT('Origin',(173.,64.,-31.));
#25331=CARTESIAN_POINT('Origin',(173.,-45.,-45.));
#25332=CARTESIAN_POINT('Origin',(173.,-45.,-45.));
#25333=CARTESIAN_POINT('Origin',(125.8,-41.1096563890154,-56.3518820725231));
#25334=CARTESIAN_POINT('',(125.8,-41.7580469908461,-54.4599017271026));
#25335=CARTESIAN_POINT('Origin',(125.8,-56.3562342901464,41.1223792414288));
#25336=CARTESIAN_POINT('',(162.,-54.463528575122,41.7686493678573));
#25337=CARTESIAN_POINT('',(125.8,-54.463528575122,41.7686493678573));
#25338=CARTESIAN_POINT('Origin',(162.,-56.3562342901464,41.1223792414288));
#25339=CARTESIAN_POINT('Origin',(175.,-45.,45.));
#25340=CARTESIAN_POINT('',(162.,-41.7580469908461,54.4599017271026));
#25341=CARTESIAN_POINT('',(125.8,-41.7580469908461,54.4599017271026));
#25342=CARTESIAN_POINT('Origin',(162.,-45.,45.));
#25343=CARTESIAN_POINT('Origin',(173.,56.3518820725231,41.1096563890154));
#25344=CARTESIAN_POINT('',(173.,54.4599017271026,41.7580469908461));
#25345=CARTESIAN_POINT('Origin',(173.,56.3518820725231,41.1096563890154));
#25346=CARTESIAN_POINT('Origin',(173.,56.3518820725231,41.1096563890154));
#25347=CARTESIAN_POINT('Origin',(173.,56.3518820725231,41.1096563890154));
#25348=CARTESIAN_POINT('Origin',(173.,41.1096563890154,56.3518820725231));
#25349=CARTESIAN_POINT('',(173.,41.7580469908461,54.4599017271026));
#25350=CARTESIAN_POINT('Origin',(173.,41.1096563890154,56.3518820725231));
#25351=CARTESIAN_POINT('Origin',(173.,41.1096563890154,56.3518820725231));
#25352=CARTESIAN_POINT('Origin',(173.,41.1096563890154,56.3518820725231));
#25353=CARTESIAN_POINT('Origin',(173.,-41.1096563890154,56.3518820725231));
#25354=CARTESIAN_POINT('Origin',(173.,-41.1096563890154,56.3518820725231));
#25355=CARTESIAN_POINT('Origin',(173.,-41.1096563890154,56.3518820725231));
#25356=CARTESIAN_POINT('Origin',(173.,32.,32.));
#25357=CARTESIAN_POINT('Origin',(173.,32.,58.));
#25358=CARTESIAN_POINT('Origin',(173.,16.,58.));
#25359=CARTESIAN_POINT('Origin',(173.,-32.,58.));
#25360=CARTESIAN_POINT('Origin',(173.,-32.,32.));
#25361=CARTESIAN_POINT('Origin',(125.8,-41.1096563890154,56.3518820725231));
#25362=CARTESIAN_POINT('Origin',(162.,-41.1096563890154,56.3518820725231));
#25363=CARTESIAN_POINT('Origin',(173.,45.,45.));
#25364=CARTESIAN_POINT('Origin',(173.,45.,45.));
#25365=CARTESIAN_POINT('Origin',(125.8,41.1096563890154,56.3518820725231));
#25366=CARTESIAN_POINT('',(125.8,41.7580469908461,54.4599017271026));
#25367=CARTESIAN_POINT('Origin',(173.,32.,32.));
#25368=CARTESIAN_POINT('Origin',(125.8,56.3518820725231,41.1096563890154));
#25369=CARTESIAN_POINT('',(125.8,54.4599017271026,41.7580469908461));
#25370=CARTESIAN_POINT('Origin',(175.,45.,45.));
#25371=CARTESIAN_POINT('Origin',(173.,56.3518820725231,-41.1096563890154));
#25372=CARTESIAN_POINT('Origin',(173.,56.3518820725231,-41.1096563890154));
#25373=CARTESIAN_POINT('Origin',(173.,56.3518820725231,-41.1096563890154));
#25374=CARTESIAN_POINT('Origin',(173.,32.,-32.));
#25375=CARTESIAN_POINT('Origin',(125.8,56.3518820725231,-41.1096563890154));
#25376=CARTESIAN_POINT('',(125.8,54.4599017271026,-41.7580469908461));
#25377=CARTESIAN_POINT('Origin',(162.,45.,-45.));
#25378=CARTESIAN_POINT('',(162.,45.,-38.5));
#25379=CARTESIAN_POINT('Origin',(162.,-45.,45.));
#25380=CARTESIAN_POINT('',(162.,-45.,51.5));
#25381=CARTESIAN_POINT('Origin',(162.,-45.,45.));
#25382=CARTESIAN_POINT('',(162.,-45.,51.5));
#25383=CARTESIAN_POINT('Origin',(162.,45.,45.));
#25384=CARTESIAN_POINT('',(162.,45.,51.5));
#25385=CARTESIAN_POINT('Origin',(162.,-45.,-45.));
#25386=CARTESIAN_POINT('',(162.,-45.,-38.5));
#25387=CARTESIAN_POINT('Origin',(175.,45.,-45.));
#25388=CARTESIAN_POINT('Origin',(162.,-45.,45.));
#25389=CARTESIAN_POINT('Origin',(175.,-45.,-45.));
#25390=CARTESIAN_POINT('Origin',(132.15,-62.,34.95));
#25391=CARTESIAN_POINT('Origin',(167.85,-62.,-34.95));
#25392=CARTESIAN_POINT('Origin',(167.85,-62.,34.95));
#25393=CARTESIAN_POINT('Origin',(132.15,-62.,-34.95));
#25394=CARTESIAN_POINT('Origin',(150.,-20.,0.));
#25395=CARTESIAN_POINT('Origin',(138.1,49.,25.4));
#25396=CARTESIAN_POINT('Origin',(161.9,49.,-25.4));
#25397=CARTESIAN_POINT('Origin',(161.9,49.,25.4));
#25398=CARTESIAN_POINT('Origin',(138.1,49.,-25.4));
#25399=CARTESIAN_POINT('Origin',(150.,20.,0.));
#25400=CARTESIAN_POINT('Origin',(128.25,0.,0.));
#25401=CARTESIAN_POINT('',(130.8,-16.6,-2.03291368658461E-15));
#25402=CARTESIAN_POINT('',(128.25,-16.6,-2.03291368658461E-15));
#25403=CARTESIAN_POINT('Origin',(130.8,0.,0.));
#25404=CARTESIAN_POINT('Origin',(130.8,16.505,0.));
#25405=CARTESIAN_POINT('',(130.8,-16.505,-2.02127954199271E-15));
#25406=CARTESIAN_POINT('Origin',(130.8,0.,0.));
#25407=CARTESIAN_POINT('Origin',(140.8,0.,0.));
#25408=CARTESIAN_POINT('',(140.8,-16.505,-2.02127954199271E-15));
#25409=CARTESIAN_POINT('Origin',(154.8,0.,0.));
#25410=CARTESIAN_POINT('Origin',(150.4,53.,33.));
#38476=UNCERTAINTY_MEASURE_WITH_UNIT(LENGTH_MEASURE(0.01),#38508,
'DISTANCE_ACCURACY_VALUE',
'Maximum model space distance between geometric entities at asserted c
onnectivities');
#38490=UNCERTAINTY_MEASURE_WITH_UNIT(LENGTH_MEASURE(0.01),#38508,
'DISTANCE_ACCURACY_VALUE',
'Maximum model space distance between geometric entities at asserted c
onnectivities');
#38493=(
GEOMETRIC_REPRESENTATION_CONTEXT(3)
GLOBAL_UNCERTAINTY_ASSIGNED_CONTEXT((#38476))
GLOBAL_UNIT_ASSIGNED_CONTEXT((#38508,#38510,#38511))
REPRESENTATION_CONTEXT('','3D')
);
#38507=(
GEOMETRIC_REPRESENTATION_CONTEXT(3)
GLOBAL_UNCERTAINTY_ASSIGNED_CONTEXT((#38490))
GLOBAL_UNIT_ASSIGNED_CONTEXT((#38508,#38510,#38511))
REPRESENTATION_CONTEXT('','3D')
);
#38508=(
LENGTH_UNIT()
NAMED_UNIT(*)
SI_UNIT(.MILLI.,.METRE.)
);
#38510=(
NAMED_UNIT(*)
PLANE_ANGLE_UNIT()
SI_UNIT($,.RADIAN.)
);
#38511=(
NAMED_UNIT(*)
SI_UNIT($,.STERADIAN.)
SOLID_ANGLE_UNIT()
);
#38514=SHAPE_DEFINITION_REPRESENTATION(#38530,#38576);
#38530=PRODUCT_DEFINITION_SHAPE('',$,#38593);
#38576=SHAPE_REPRESENTATION('',(#15494),#38493);
#38590=PRODUCT_DEFINITION_CONTEXT('part definition',#38640,'design');
#38593=PRODUCT_DEFINITION('2026-10-26-01-10-37-592',
'02_Port_Plate_Rear_Cap',#38609,#38590);
#38609=PRODUCT_DEFINITION_FORMATION('',$,#38644);
#38640=APPLICATION_CONTEXT(
'Core Data for Automotive Mechanical Design Process');
#38641=PRODUCT_CONTEXT('part definition',#38640,'mechanical');
#38644=PRODUCT('2026-10-26-01-10-37-592','02_Port_Plate_Rear_Cap',$,(#38641));
#38707=COLOUR_RGB('Sky Blue',0.24,0.69,0.87);
#38708=FILL_AREA_STYLE_COLOUR('',#38707);
#38709=FILL_AREA_STYLE('',(#38708));
#38710=SURFACE_STYLE_FILL_AREA(#38709);
#38711=SURFACE_SIDE_STYLE('',(#38710));
#38712=SURFACE_STYLE_USAGE(.BOTH.,#38711);
#38713=PRESENTATION_STYLE_ASSIGNMENT((#38712));
ENDSEC;
END-ISO-10303-21;
